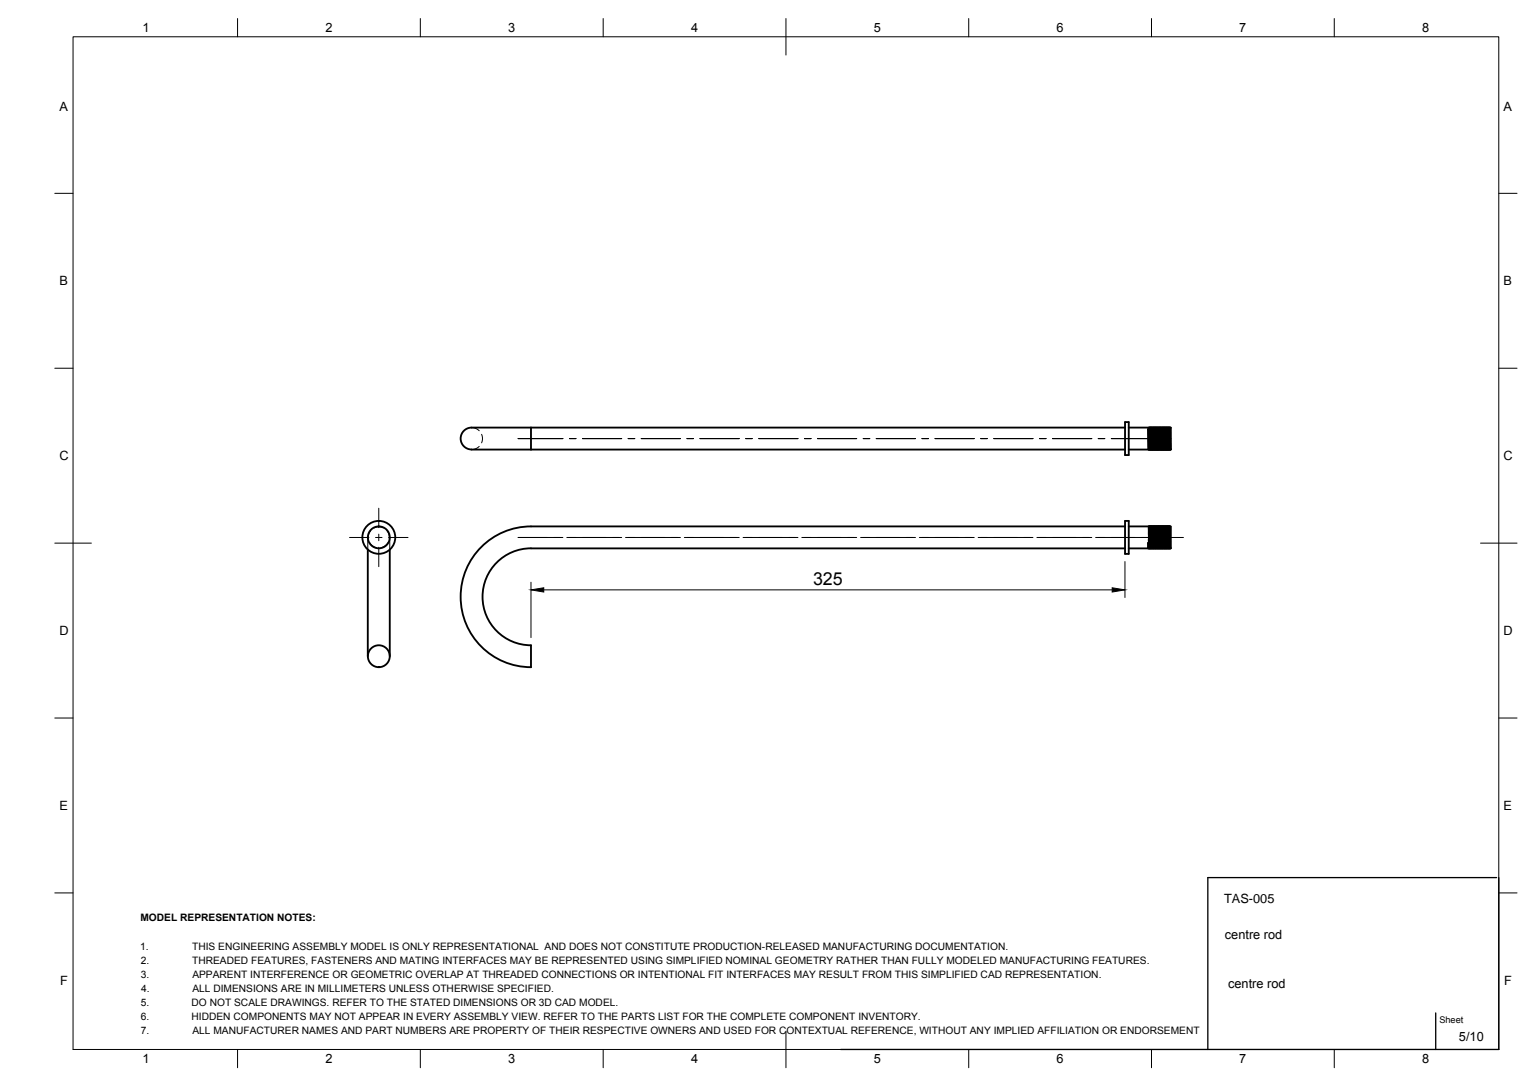
ISO-10303-21;
HEADER;
/* Generated by software containing ST-Developer
 * from STEP Tools, Inc. (www.steptools.com) 
 */

FILE_DESCRIPTION(
/* description */ ('STEP AP214'),
/* implementation_level */ '2;1');

FILE_NAME(
/* name */ 'centre rod.step',
/* time_stamp */ '2026-11-04T19:54:22-08:00',
/* author */ (''),
/* organization */ (''),
/* preprocessor_version */ 'ST-DEVELOPER v20.2',
/* originating_system */ 'Autodesk Translation Framework v15.17.0.0',
/* authorisation */ '');

FILE_SCHEMA (('AUTOMOTIVE_DESIGN { 1 0 10303 214 3 1 1 }'));
ENDSEC;

DATA;
#10=MECHANICAL_DESIGN_GEOMETRIC_PRESENTATION_REPRESENTATION('',(#241),#14084);
#61=(
BOUNDED_SURFACE()
B_SPLINE_SURFACE(1,2,((#7888,#7889,#7890,#7891,#7892,#7893,#7894,#7895,
#7896,#7897,#7898,#7899,#7900,#7901,#7902,#7903,#7904,#7905,#7906,#7907,
#7908,#7909,#7910,#7911,#7912,#7913,#7914,#7915,#7916,#7917,#7918,#7919,
#7920,#7921,#7922,#7923,#7924,#7925,#7926,#7927,#7928,#7929,#7930,#7931,
#7932,#7933,#7934,#7935,#7936,#7937,#7938,#7939,#7940,#7941,#7942,#7943,
#7944,#7945,#7946,#7947,#7948,#7949,#7950,#7951,#7952,#7953,#7954,#7955,
#7956,#7957,#7958,#7959,#7960,#7961,#7962,#7963,#7964,#7965,#7966,#7967,
#7968,#7969,#7970,#7971,#7972,#7973,#7974,#7975,#7976,#7977,#7978,#7979,
#7980,#7981,#7982,#7983,#7984,#7985,#7986,#7987,#7988,#7989,#7990,#7991,
#7992,#7993,#7994,#7995,#7996,#7997,#7998,#7999,#8000,#8001,#8002,#8003,
#8004,#8005,#8006,#8007,#8008,#8009,#8010,#8011,#8012,#8013,#8014,#8015,
#8016,#8017,#8018,#8019,#8020,#8021,#8022,#8023,#8024,#8025,#8026,#8027,
#8028,#8029,#8030,#8031,#8032,#8033,#8034,#8035,#8036,#8037,#8038,#8039,
#8040,#8041,#8042,#8043,#8044,#8045,#8046,#8047,#8048,#8049,#8050,#8051,
#8052,#8053,#8054,#8055,#8056,#8057,#8058,#8059,#8060,#8061,#8062,#8063,
#8064,#8065,#8066,#8067,#8068,#8069,#8070,#8071,#8072,#8073,#8074,#8075,
#8076,#8077,#8078,#8079,#8080,#8081,#8082,#8083,#8084,#8085,#8086,#8087,
#8088,#8089,#8090,#8091,#8092,#8093,#8094,#8095,#8096,#8097,#8098,#8099,
#8100,#8101,#8102,#8103,#8104,#8105,#8106,#8107,#8108,#8109,#8110,#8111,
#8112,#8113,#8114,#8115,#8116,#8117,#8118,#8119,#8120,#8121,#8122,#8123,
#8124,#8125,#8126,#8127,#8128,#8129,#8130,#8131,#8132,#8133,#8134,#8135,
#8136,#8137,#8138,#8139,#8140,#8141,#8142,#8143,#8144,#8145,#8146,#8147,
#8148,#8149,#8150,#8151,#8152,#8153,#8154,#8155,#8156,#8157,#8158,#8159,
#8160,#8161,#8162,#8163,#8164,#8165,#8166,#8167,#8168,#8169,#8170,#8171,
#8172,#8173,#8174,#8175,#8176,#8177,#8178,#8179,#8180,#8181,#8182,#8183,
#8184,#8185,#8186,#8187,#8188,#8189,#8190,#8191,#8192,#8193,#8194,#8195,
#8196,#8197,#8198,#8199,#8200,#8201,#8202,#8203,#8204,#8205,#8206,#8207,
#8208),(#8209,#8210,#8211,#8212,#8213,#8214,#8215,#8216,#8217,#8218,#8219,
#8220,#8221,#8222,#8223,#8224,#8225,#8226,#8227,#8228,#8229,#8230,#8231,
#8232,#8233,#8234,#8235,#8236,#8237,#8238,#8239,#8240,#8241,#8242,#8243,
#8244,#8245,#8246,#8247,#8248,#8249,#8250,#8251,#8252,#8253,#8254,#8255,
#8256,#8257,#8258,#8259,#8260,#8261,#8262,#8263,#8264,#8265,#8266,#8267,
#8268,#8269,#8270,#8271,#8272,#8273,#8274,#8275,#8276,#8277,#8278,#8279,
#8280,#8281,#8282,#8283,#8284,#8285,#8286,#8287,#8288,#8289,#8290,#8291,
#8292,#8293,#8294,#8295,#8296,#8297,#8298,#8299,#8300,#8301,#8302,#8303,
#8304,#8305,#8306,#8307,#8308,#8309,#8310,#8311,#8312,#8313,#8314,#8315,
#8316,#8317,#8318,#8319,#8320,#8321,#8322,#8323,#8324,#8325,#8326,#8327,
#8328,#8329,#8330,#8331,#8332,#8333,#8334,#8335,#8336,#8337,#8338,#8339,
#8340,#8341,#8342,#8343,#8344,#8345,#8346,#8347,#8348,#8349,#8350,#8351,
#8352,#8353,#8354,#8355,#8356,#8357,#8358,#8359,#8360,#8361,#8362,#8363,
#8364,#8365,#8366,#8367,#8368,#8369,#8370,#8371,#8372,#8373,#8374,#8375,
#8376,#8377,#8378,#8379,#8380,#8381,#8382,#8383,#8384,#8385,#8386,#8387,
#8388,#8389,#8390,#8391,#8392,#8393,#8394,#8395,#8396,#8397,#8398,#8399,
#8400,#8401,#8402,#8403,#8404,#8405,#8406,#8407,#8408,#8409,#8410,#8411,
#8412,#8413,#8414,#8415,#8416,#8417,#8418,#8419,#8420,#8421,#8422,#8423,
#8424,#8425,#8426,#8427,#8428,#8429,#8430,#8431,#8432,#8433,#8434,#8435,
#8436,#8437,#8438,#8439,#8440,#8441,#8442,#8443,#8444,#8445,#8446,#8447,
#8448,#8449,#8450,#8451,#8452,#8453,#8454,#8455,#8456,#8457,#8458,#8459,
#8460,#8461,#8462,#8463,#8464,#8465,#8466,#8467,#8468,#8469,#8470,#8471,
#8472,#8473,#8474,#8475,#8476,#8477,#8478,#8479,#8480,#8481,#8482,#8483,
#8484,#8485,#8486,#8487,#8488,#8489,#8490,#8491,#8492,#8493,#8494,#8495,
#8496,#8497,#8498,#8499,#8500,#8501,#8502,#8503,#8504,#8505,#8506,#8507,
#8508,#8509,#8510,#8511,#8512,#8513,#8514,#8515,#8516,#8517,#8518,#8519,
#8520,#8521,#8522,#8523,#8524,#8525,#8526,#8527,#8528,#8529)),
 .UNSPECIFIED.,.F.,.F.,.F.)
B_SPLINE_SURFACE_WITH_KNOTS((2,2),(3,2,2,2,2,2,2,2,2,2,2,2,2,2,2,2,2,2,
2,2,2,2,2,2,2,2,2,2,2,2,2,2,2,2,2,2,2,2,2,2,2,2,2,2,2,2,2,2,2,2,2,2,2,2,
2,2,2,2,2,2,2,2,2,2,2,2,2,2,2,2,2,2,2,2,2,2,2,2,2,2,2,2,2,2,2,2,2,2,2,2,
2,2,2,2,2,2,2,2,2,2,2,2,2,2,2,2,2,2,2,2,2,2,2,2,2,2,2,2,2,2,2,2,2,2,2,2,
2,2,2,2,2,2,2,2,2,2,2,2,2,2,2,2,2,2,2,2,2,2,2,2,2,2,2,2,2,2,2,2,2,2,3),
(0.,1.),(0.,0.00617283950617284,0.0123456790123457,0.0185185185185185,0.0246913580246914,
0.0308641975308642,0.037037037037037,0.0432098765432099,0.0493827160493827,
0.0555555555555556,0.0617283950617284,0.0679012345679012,0.0740740740740741,
0.0802469135802469,0.0864197530864197,0.0925925925925926,0.0987654320987654,
0.104938271604938,0.111111111111111,0.117283950617284,0.123456790123457,
0.12962962962963,0.135802469135802,0.141975308641975,0.148148148148148,
0.154320987654321,0.160493827160494,0.166666666666667,0.172839506172839,
0.179012345679012,0.185185185185185,0.191358024691358,0.197530864197531,
0.203703703703704,0.209876543209877,0.216049382716049,0.222222222222222,
0.228395061728395,0.234567901234568,0.240740740740741,0.246913580246914,
0.253086419753086,0.259259259259259,0.265432098765432,0.271604938271605,
0.277777777777778,0.283950617283951,0.290123456790123,0.296296296296296,
0.302469135802469,0.308641975308642,0.314814814814815,0.320987654320988,
0.327160493827161,0.333333333333333,0.339506172839506,0.345679012345679,
0.351851851851852,0.358024691358025,0.364197530864198,0.37037037037037,
0.376543209876543,0.382716049382716,0.388888888888889,0.395061728395062,
0.401234567901235,0.407407407407407,0.41358024691358,0.419753086419753,
0.425925925925926,0.432098765432099,0.438271604938272,0.444444444444444,
0.450617283950617,0.45679012345679,0.462962962962963,0.469135802469136,
0.475308641975309,0.481481481481481,0.487654320987654,0.493827160493827,
0.5,0.506172839506173,0.512345679012346,0.518518518518518,0.524691358024691,
0.530864197530864,0.537037037037037,0.54320987654321,0.549382716049383,
0.555555555555556,0.561728395061728,0.567901234567901,0.574074074074074,
0.580246913580247,0.58641975308642,0.592592592592593,0.598765432098765,
0.604938271604938,0.611111111111111,0.617283950617284,0.623456790123457,
0.62962962962963,0.635802469135803,0.641975308641975,0.648148148148148,
0.654320987654321,0.660493827160494,0.666666666666667,0.672839506172839,
0.679012345679012,0.685185185185185,0.691358024691358,0.697530864197531,
0.703703703703704,0.709876543209877,0.716049382716049,0.722222222222222,
0.728395061728395,0.734567901234568,0.740740740740741,0.746913580246914,
0.753086419753086,0.759259259259259,0.765432098765432,0.771604938271605,
0.777777777777778,0.783950617283951,0.790123456790123,0.796296296296296,
0.802469135802469,0.808641975308642,0.814814814814815,0.820987654320988,
0.827160493827161,0.833333333333333,0.839506172839506,0.845679012345679,
0.851851851851852,0.858024691358025,0.864197530864197,0.87037037037037,
0.876543209876543,0.882716049382716,0.888888888888889,0.895061728395062,
0.901234567901235,0.907407407407407,0.91358024691358,0.919753086419753,
0.925925925925926,0.932098765432099,0.938271604938272,0.944444444444444,
0.950617283950617,0.95679012345679,0.962962962962963,0.969135802469136,
0.975308641975309,0.981481481481482,0.987654320987654),.UNSPECIFIED.)
GEOMETRIC_REPRESENTATION_ITEM()
RATIONAL_B_SPLINE_SURFACE(((1.,0.866025403784439,1.,0.866025403784439,1.,
0.866025403784439,1.,0.866025403784439,1.,0.866025403784439,1.,0.866025403784439,
1.,0.866025403784439,1.,0.866025403784439,1.,0.866025403784439,1.,0.866025403784439,
1.,0.866025403784439,1.,0.866025403784439,1.,0.866025403784439,1.,0.866025403784439,
1.,0.866025403784439,1.,0.866025403784439,1.,0.866025403784439,1.,0.866025403784439,
1.,0.866025403784439,1.,0.866025403784439,1.,0.866025403784439,1.,0.866025403784439,
1.,0.866025403784439,1.,0.866025403784439,1.,0.866025403784439,1.,0.866025403784439,
1.,0.866025403784439,1.,0.866025403784439,1.,0.866025403784439,1.,0.866025403784439,
1.,0.866025403784439,1.,0.866025403784439,1.,0.866025403784439,1.,0.866025403784439,
1.,0.866025403784439,1.,0.866025403784439,1.,0.866025403784439,1.,0.866025403784439,
1.,0.866025403784439,1.,0.866025403784439,1.,0.866025403784439,1.,0.866025403784439,
1.,0.866025403784439,1.,0.866025403784439,1.,0.866025403784439,1.,0.866025403784439,
1.,0.866025403784439,1.,0.866025403784439,1.,0.866025403784439,1.,0.866025403784439,
1.,0.866025403784439,1.,0.866025403784439,1.,0.866025403784439,1.,0.866025403784439,
1.,0.866025403784439,1.,0.866025403784439,1.,0.866025403784439,1.,0.866025403784439,
1.,0.866025403784439,1.,0.866025403784439,1.,0.866025403784439,1.,0.866025403784439,
1.,0.866025403784439,1.,0.866025403784439,1.,0.866025403784439,1.,0.866025403784439,
1.,0.866025403784439,1.,0.866025403784439,1.,0.866025403784439,1.,0.866025403784439,
1.,0.866025403784439,1.,0.866025403784439,1.,0.866025403784439,1.,0.866025403784439,
1.,0.866025403784439,1.,0.866025403784439,1.,0.866025403784439,1.,0.866025403784439,
1.,0.866025403784439,1.,0.866025403784439,1.,0.866025403784439,1.,0.866025403784439,
1.,0.866025403784439,1.,0.866025403784439,1.,0.866025403784439,1.,0.866025403784439,
1.,0.866025403784439,1.,0.866025403784439,1.,0.866025403784439,1.,0.866025403784439,
1.,0.866025403784439,1.,0.866025403784439,1.,0.866025403784439,1.,0.866025403784439,
1.,0.866025403784439,1.,0.866025403784439,1.,0.866025403784439,1.,0.866025403784439,
1.,0.866025403784439,1.,0.866025403784439,1.,0.866025403784439,1.,0.866025403784439,
1.,0.866025403784439,1.,0.866025403784439,1.,0.866025403784439,1.,0.866025403784439,
1.,0.866025403784439,1.,0.866025403784439,1.,0.866025403784439,1.,0.866025403784439,
1.,0.866025403784439,1.,0.866025403784439,1.,0.866025403784439,1.,0.866025403784439,
1.,0.866025403784439,1.,0.866025403784439,1.,0.866025403784439,1.,0.866025403784439,
1.,0.866025403784439,1.,0.866025403784439,1.,0.866025403784439,1.,0.866025403784439,
1.,0.866025403784439,1.,0.866025403784439,1.,0.866025403784439,1.,0.866025403784439,
1.,0.866025403784439,1.,0.866025403784439,1.,0.866025403784439,1.,0.866025403784439,
1.,0.866025403784439,1.,0.866025403784439,1.,0.866025403784439,1.,0.866025403784439,
1.,0.866025403784439,1.,0.866025403784439,1.,0.866025403784439,1.,0.866025403784439,
1.,0.866025403784439,1.,0.866025403784439,1.,0.866025403784439,1.,0.866025403784439,
1.,0.866025403784439,1.,0.866025403784439,1.,0.866025403784439,1.,0.866025403784439,
1.,0.866025403784439,1.,0.866025403784439,1.,0.866025403784439,1.,0.866025403784439,
1.,0.866025403784439,1.,0.866025403784439,1.,0.866025403784439,1.,0.866025403784439,
1.,0.866025403784439,1.,0.866025403784439,1.,0.866025403784439,1.,0.866025403784439,
1.,0.866025403784439,1.,0.866025403784439,1.),(1.,0.866025403784439,1.,
0.866025403784439,1.,0.866025403784439,1.,0.866025403784439,1.,0.866025403784439,
1.,0.866025403784439,1.,0.866025403784439,1.,0.866025403784439,1.,0.866025403784439,
1.,0.866025403784439,1.,0.866025403784439,1.,0.866025403784439,1.,0.866025403784439,
1.,0.866025403784439,1.,0.866025403784439,1.,0.866025403784439,1.,0.866025403784439,
1.,0.866025403784439,1.,0.866025403784439,1.,0.866025403784439,1.,0.866025403784439,
1.,0.866025403784439,1.,0.866025403784439,1.,0.866025403784439,1.,0.866025403784439,
1.,0.866025403784439,1.,0.866025403784439,1.,0.866025403784439,1.,0.866025403784439,
1.,0.866025403784439,1.,0.866025403784439,1.,0.866025403784439,1.,0.866025403784439,
1.,0.866025403784439,1.,0.866025403784439,1.,0.866025403784439,1.,0.866025403784439,
1.,0.866025403784439,1.,0.866025403784439,1.,0.866025403784439,1.,0.866025403784439,
1.,0.866025403784439,1.,0.866025403784439,1.,0.866025403784439,1.,0.866025403784439,
1.,0.866025403784439,1.,0.866025403784439,1.,0.866025403784439,1.,0.866025403784439,
1.,0.866025403784439,1.,0.866025403784439,1.,0.866025403784439,1.,0.866025403784439,
1.,0.866025403784439,1.,0.866025403784439,1.,0.866025403784439,1.,0.866025403784439,
1.,0.866025403784439,1.,0.866025403784439,1.,0.866025403784439,1.,0.866025403784439,
1.,0.866025403784439,1.,0.866025403784439,1.,0.866025403784439,1.,0.866025403784439,
1.,0.866025403784439,1.,0.866025403784439,1.,0.866025403784439,1.,0.866025403784439,
1.,0.866025403784439,1.,0.866025403784439,1.,0.866025403784439,1.,0.866025403784439,
1.,0.866025403784439,1.,0.866025403784439,1.,0.866025403784439,1.,0.866025403784439,
1.,0.866025403784439,1.,0.866025403784439,1.,0.866025403784439,1.,0.866025403784439,
1.,0.866025403784439,1.,0.866025403784439,1.,0.866025403784439,1.,0.866025403784439,
1.,0.866025403784439,1.,0.866025403784439,1.,0.866025403784439,1.,0.866025403784439,
1.,0.866025403784439,1.,0.866025403784439,1.,0.866025403784439,1.,0.866025403784439,
1.,0.866025403784439,1.,0.866025403784439,1.,0.866025403784439,1.,0.866025403784439,
1.,0.866025403784439,1.,0.866025403784439,1.,0.866025403784439,1.,0.866025403784439,
1.,0.866025403784439,1.,0.866025403784439,1.,0.866025403784439,1.,0.866025403784439,
1.,0.866025403784439,1.,0.866025403784439,1.,0.866025403784439,1.,0.866025403784439,
1.,0.866025403784439,1.,0.866025403784439,1.,0.866025403784439,1.,0.866025403784439,
1.,0.866025403784439,1.,0.866025403784439,1.,0.866025403784439,1.,0.866025403784439,
1.,0.866025403784439,1.,0.866025403784439,1.,0.866025403784439,1.,0.866025403784439,
1.,0.866025403784439,1.,0.866025403784439,1.,0.866025403784439,1.,0.866025403784439,
1.,0.866025403784439,1.,0.866025403784439,1.,0.866025403784439,1.,0.866025403784439,
1.,0.866025403784439,1.,0.866025403784439,1.,0.866025403784439,1.,0.866025403784439,
1.,0.866025403784439,1.,0.866025403784439,1.,0.866025403784439,1.,0.866025403784439,
1.,0.866025403784439,1.,0.866025403784439,1.,0.866025403784439,1.,0.866025403784439,
1.,0.866025403784439,1.,0.866025403784439,1.,0.866025403784439,1.,0.866025403784439,
1.,0.866025403784439,1.,0.866025403784439,1.,0.866025403784439,1.,0.866025403784439,
1.,0.866025403784439,1.,0.866025403784439,1.,0.866025403784439,1.,0.866025403784439,
1.,0.866025403784439,1.,0.866025403784439,1.,0.866025403784439,1.,0.866025403784439,
1.,0.866025403784439,1.,0.866025403784439,1.,0.866025403784439,1.)))
REPRESENTATION_ITEM('')
SURFACE()
);
#62=(
BOUNDED_SURFACE()
B_SPLINE_SURFACE(1,2,((#8545,#8546,#8547,#8548,#8549,#8550,#8551,#8552,
#8553,#8554,#8555,#8556,#8557,#8558,#8559,#8560,#8561,#8562,#8563,#8564,
#8565,#8566,#8567,#8568,#8569,#8570,#8571,#8572,#8573,#8574,#8575,#8576,
#8577,#8578,#8579,#8580,#8581,#8582,#8583,#8584,#8585,#8586,#8587,#8588,
#8589,#8590,#8591,#8592,#8593,#8594,#8595,#8596,#8597,#8598,#8599,#8600,
#8601,#8602,#8603,#8604,#8605,#8606,#8607,#8608,#8609,#8610,#8611,#8612,
#8613,#8614,#8615,#8616,#8617,#8618,#8619,#8620,#8621,#8622,#8623,#8624,
#8625,#8626,#8627,#8628,#8629,#8630,#8631,#8632,#8633,#8634,#8635,#8636,
#8637,#8638,#8639,#8640,#8641,#8642,#8643,#8644,#8645,#8646,#8647,#8648,
#8649,#8650,#8651,#8652,#8653,#8654,#8655,#8656,#8657,#8658,#8659,#8660,
#8661,#8662,#8663,#8664,#8665,#8666,#8667,#8668,#8669,#8670,#8671,#8672,
#8673,#8674,#8675,#8676,#8677,#8678,#8679,#8680,#8681,#8682,#8683,#8684,
#8685,#8686,#8687,#8688,#8689,#8690,#8691,#8692,#8693,#8694,#8695,#8696,
#8697,#8698,#8699,#8700,#8701,#8702,#8703,#8704,#8705,#8706,#8707,#8708,
#8709,#8710,#8711,#8712,#8713,#8714,#8715,#8716,#8717,#8718,#8719,#8720,
#8721,#8722,#8723,#8724,#8725,#8726,#8727,#8728,#8729,#8730,#8731,#8732,
#8733,#8734,#8735,#8736,#8737,#8738,#8739,#8740,#8741,#8742,#8743,#8744,
#8745,#8746,#8747,#8748,#8749,#8750,#8751,#8752,#8753,#8754,#8755,#8756,
#8757,#8758,#8759,#8760,#8761,#8762,#8763,#8764,#8765,#8766,#8767,#8768,
#8769,#8770,#8771,#8772,#8773,#8774,#8775,#8776,#8777,#8778,#8779,#8780,
#8781,#8782,#8783,#8784,#8785,#8786,#8787,#8788,#8789,#8790,#8791,#8792,
#8793,#8794,#8795,#8796,#8797,#8798,#8799,#8800,#8801,#8802,#8803,#8804,
#8805,#8806,#8807,#8808,#8809,#8810,#8811,#8812,#8813,#8814,#8815,#8816,
#8817,#8818,#8819,#8820,#8821,#8822,#8823,#8824,#8825,#8826,#8827,#8828,
#8829,#8830,#8831,#8832,#8833,#8834,#8835,#8836,#8837,#8838,#8839,#8840,
#8841,#8842,#8843,#8844,#8845,#8846,#8847,#8848,#8849,#8850,#8851,#8852,
#8853,#8854,#8855,#8856,#8857,#8858,#8859,#8860,#8861,#8862,#8863,#8864,
#8865),(#8866,#8867,#8868,#8869,#8870,#8871,#8872,#8873,#8874,#8875,#8876,
#8877,#8878,#8879,#8880,#8881,#8882,#8883,#8884,#8885,#8886,#8887,#8888,
#8889,#8890,#8891,#8892,#8893,#8894,#8895,#8896,#8897,#8898,#8899,#8900,
#8901,#8902,#8903,#8904,#8905,#8906,#8907,#8908,#8909,#8910,#8911,#8912,
#8913,#8914,#8915,#8916,#8917,#8918,#8919,#8920,#8921,#8922,#8923,#8924,
#8925,#8926,#8927,#8928,#8929,#8930,#8931,#8932,#8933,#8934,#8935,#8936,
#8937,#8938,#8939,#8940,#8941,#8942,#8943,#8944,#8945,#8946,#8947,#8948,
#8949,#8950,#8951,#8952,#8953,#8954,#8955,#8956,#8957,#8958,#8959,#8960,
#8961,#8962,#8963,#8964,#8965,#8966,#8967,#8968,#8969,#8970,#8971,#8972,
#8973,#8974,#8975,#8976,#8977,#8978,#8979,#8980,#8981,#8982,#8983,#8984,
#8985,#8986,#8987,#8988,#8989,#8990,#8991,#8992,#8993,#8994,#8995,#8996,
#8997,#8998,#8999,#9000,#9001,#9002,#9003,#9004,#9005,#9006,#9007,#9008,
#9009,#9010,#9011,#9012,#9013,#9014,#9015,#9016,#9017,#9018,#9019,#9020,
#9021,#9022,#9023,#9024,#9025,#9026,#9027,#9028,#9029,#9030,#9031,#9032,
#9033,#9034,#9035,#9036,#9037,#9038,#9039,#9040,#9041,#9042,#9043,#9044,
#9045,#9046,#9047,#9048,#9049,#9050,#9051,#9052,#9053,#9054,#9055,#9056,
#9057,#9058,#9059,#9060,#9061,#9062,#9063,#9064,#9065,#9066,#9067,#9068,
#9069,#9070,#9071,#9072,#9073,#9074,#9075,#9076,#9077,#9078,#9079,#9080,
#9081,#9082,#9083,#9084,#9085,#9086,#9087,#9088,#9089,#9090,#9091,#9092,
#9093,#9094,#9095,#9096,#9097,#9098,#9099,#9100,#9101,#9102,#9103,#9104,
#9105,#9106,#9107,#9108,#9109,#9110,#9111,#9112,#9113,#9114,#9115,#9116,
#9117,#9118,#9119,#9120,#9121,#9122,#9123,#9124,#9125,#9126,#9127,#9128,
#9129,#9130,#9131,#9132,#9133,#9134,#9135,#9136,#9137,#9138,#9139,#9140,
#9141,#9142,#9143,#9144,#9145,#9146,#9147,#9148,#9149,#9150,#9151,#9152,
#9153,#9154,#9155,#9156,#9157,#9158,#9159,#9160,#9161,#9162,#9163,#9164,
#9165,#9166,#9167,#9168,#9169,#9170,#9171,#9172,#9173,#9174,#9175,#9176,
#9177,#9178,#9179,#9180,#9181,#9182,#9183,#9184,#9185,#9186)),
 .UNSPECIFIED.,.F.,.F.,.F.)
B_SPLINE_SURFACE_WITH_KNOTS((2,2),(3,2,2,2,2,2,2,2,2,2,2,2,2,2,2,2,2,2,
2,2,2,2,2,2,2,2,2,2,2,2,2,2,2,2,2,2,2,2,2,2,2,2,2,2,2,2,2,2,2,2,2,2,2,2,
2,2,2,2,2,2,2,2,2,2,2,2,2,2,2,2,2,2,2,2,2,2,2,2,2,2,2,2,2,2,2,2,2,2,2,2,
2,2,2,2,2,2,2,2,2,2,2,2,2,2,2,2,2,2,2,2,2,2,2,2,2,2,2,2,2,2,2,2,2,2,2,2,
2,2,2,2,2,2,2,2,2,2,2,2,2,2,2,2,2,2,2,2,2,2,2,2,2,2,2,2,2,2,2,2,2,2,3),
(0.,1.),(0.,0.00617283950617284,0.0123456790123457,0.0185185185185185,0.0246913580246914,
0.0308641975308642,0.037037037037037,0.0432098765432099,0.0493827160493827,
0.0555555555555556,0.0617283950617284,0.0679012345679012,0.0740740740740741,
0.0802469135802469,0.0864197530864197,0.0925925925925926,0.0987654320987654,
0.104938271604938,0.111111111111111,0.117283950617284,0.123456790123457,
0.12962962962963,0.135802469135802,0.141975308641975,0.148148148148148,
0.154320987654321,0.160493827160494,0.166666666666667,0.172839506172839,
0.179012345679012,0.185185185185185,0.191358024691358,0.197530864197531,
0.203703703703704,0.209876543209877,0.216049382716049,0.222222222222222,
0.228395061728395,0.234567901234568,0.240740740740741,0.246913580246914,
0.253086419753086,0.259259259259259,0.265432098765432,0.271604938271605,
0.277777777777778,0.283950617283951,0.290123456790123,0.296296296296296,
0.302469135802469,0.308641975308642,0.314814814814815,0.320987654320988,
0.327160493827161,0.333333333333333,0.339506172839506,0.345679012345679,
0.351851851851852,0.358024691358025,0.364197530864198,0.37037037037037,
0.376543209876543,0.382716049382716,0.388888888888889,0.395061728395062,
0.401234567901235,0.407407407407407,0.41358024691358,0.419753086419753,
0.425925925925926,0.432098765432099,0.438271604938272,0.444444444444444,
0.450617283950617,0.45679012345679,0.462962962962963,0.469135802469136,
0.475308641975309,0.481481481481481,0.487654320987654,0.493827160493827,
0.5,0.506172839506173,0.512345679012346,0.518518518518518,0.524691358024691,
0.530864197530864,0.537037037037037,0.54320987654321,0.549382716049383,
0.555555555555556,0.561728395061728,0.567901234567901,0.574074074074074,
0.580246913580247,0.58641975308642,0.592592592592593,0.598765432098765,
0.604938271604938,0.611111111111111,0.617283950617284,0.623456790123457,
0.62962962962963,0.635802469135803,0.641975308641975,0.648148148148148,
0.654320987654321,0.660493827160494,0.666666666666667,0.672839506172839,
0.679012345679012,0.685185185185185,0.691358024691358,0.697530864197531,
0.703703703703704,0.709876543209877,0.716049382716049,0.722222222222222,
0.728395061728395,0.734567901234568,0.740740740740741,0.746913580246914,
0.753086419753086,0.759259259259259,0.765432098765432,0.771604938271605,
0.777777777777778,0.783950617283951,0.790123456790123,0.796296296296296,
0.802469135802469,0.808641975308642,0.814814814814815,0.820987654320988,
0.827160493827161,0.833333333333333,0.839506172839506,0.845679012345679,
0.851851851851852,0.858024691358025,0.864197530864197,0.87037037037037,
0.876543209876543,0.882716049382716,0.888888888888889,0.895061728395062,
0.901234567901235,0.907407407407407,0.91358024691358,0.919753086419753,
0.925925925925926,0.932098765432099,0.938271604938272,0.944444444444444,
0.950617283950617,0.95679012345679,0.962962962962963,0.969135802469136,
0.975308641975309,0.981481481481482,0.987654320987654),.UNSPECIFIED.)
GEOMETRIC_REPRESENTATION_ITEM()
RATIONAL_B_SPLINE_SURFACE(((1.,0.866025403784439,1.,0.866025403784439,1.,
0.866025403784439,1.,0.866025403784439,1.,0.866025403784439,1.,0.866025403784439,
1.,0.866025403784439,1.,0.866025403784439,1.,0.866025403784439,1.,0.866025403784439,
1.,0.866025403784439,1.,0.866025403784439,1.,0.866025403784439,1.,0.866025403784439,
1.,0.866025403784439,1.,0.866025403784439,1.,0.866025403784439,1.,0.866025403784439,
1.,0.866025403784439,1.,0.866025403784439,1.,0.866025403784439,1.,0.866025403784439,
1.,0.866025403784439,1.,0.866025403784439,1.,0.866025403784439,1.,0.866025403784439,
1.,0.866025403784439,1.,0.866025403784439,1.,0.866025403784439,1.,0.866025403784439,
1.,0.866025403784439,1.,0.866025403784439,1.,0.866025403784439,1.,0.866025403784439,
1.,0.866025403784439,1.,0.866025403784439,1.,0.866025403784439,1.,0.866025403784439,
1.,0.866025403784439,1.,0.866025403784439,1.,0.866025403784439,1.,0.866025403784439,
1.,0.866025403784439,1.,0.866025403784439,1.,0.866025403784439,1.,0.866025403784439,
1.,0.866025403784439,1.,0.866025403784439,1.,0.866025403784439,1.,0.866025403784439,
1.,0.866025403784439,1.,0.866025403784439,1.,0.866025403784439,1.,0.866025403784439,
1.,0.866025403784439,1.,0.866025403784439,1.,0.866025403784439,1.,0.866025403784439,
1.,0.866025403784439,1.,0.866025403784439,1.,0.866025403784439,1.,0.866025403784439,
1.,0.866025403784439,1.,0.866025403784439,1.,0.866025403784439,1.,0.866025403784439,
1.,0.866025403784439,1.,0.866025403784439,1.,0.866025403784439,1.,0.866025403784439,
1.,0.866025403784439,1.,0.866025403784439,1.,0.866025403784439,1.,0.866025403784439,
1.,0.866025403784439,1.,0.866025403784439,1.,0.866025403784439,1.,0.866025403784439,
1.,0.866025403784439,1.,0.866025403784439,1.,0.866025403784439,1.,0.866025403784439,
1.,0.866025403784439,1.,0.866025403784439,1.,0.866025403784439,1.,0.866025403784439,
1.,0.866025403784439,1.,0.866025403784439,1.,0.866025403784439,1.,0.866025403784439,
1.,0.866025403784439,1.,0.866025403784439,1.,0.866025403784439,1.,0.866025403784439,
1.,0.866025403784439,1.,0.866025403784439,1.,0.866025403784439,1.,0.866025403784439,
1.,0.866025403784439,1.,0.866025403784439,1.,0.866025403784439,1.,0.866025403784439,
1.,0.866025403784439,1.,0.866025403784439,1.,0.866025403784439,1.,0.866025403784439,
1.,0.866025403784439,1.,0.866025403784439,1.,0.866025403784439,1.,0.866025403784439,
1.,0.866025403784439,1.,0.866025403784439,1.,0.866025403784439,1.,0.866025403784439,
1.,0.866025403784439,1.,0.866025403784439,1.,0.866025403784439,1.,0.866025403784439,
1.,0.866025403784439,1.,0.866025403784439,1.,0.866025403784439,1.,0.866025403784439,
1.,0.866025403784439,1.,0.866025403784439,1.,0.866025403784439,1.,0.866025403784439,
1.,0.866025403784439,1.,0.866025403784439,1.,0.866025403784439,1.,0.866025403784439,
1.,0.866025403784439,1.,0.866025403784439,1.,0.866025403784439,1.,0.866025403784439,
1.,0.866025403784439,1.,0.866025403784439,1.,0.866025403784439,1.,0.866025403784439,
1.,0.866025403784439,1.,0.866025403784439,1.,0.866025403784439,1.,0.866025403784439,
1.,0.866025403784439,1.,0.866025403784439,1.,0.866025403784439,1.,0.866025403784439,
1.,0.866025403784439,1.,0.866025403784439,1.,0.866025403784439,1.,0.866025403784439,
1.,0.866025403784439,1.,0.866025403784439,1.,0.866025403784439,1.,0.866025403784439,
1.,0.866025403784439,1.,0.866025403784439,1.,0.866025403784439,1.,0.866025403784439,
1.,0.866025403784439,1.,0.866025403784439,1.),(1.,0.866025403784439,1.,
0.866025403784439,1.,0.866025403784439,1.,0.866025403784439,1.,0.866025403784439,
1.,0.866025403784439,1.,0.866025403784439,1.,0.866025403784439,1.,0.866025403784439,
1.,0.866025403784439,1.,0.866025403784439,1.,0.866025403784439,1.,0.866025403784439,
1.,0.866025403784439,1.,0.866025403784439,1.,0.866025403784439,1.,0.866025403784439,
1.,0.866025403784439,1.,0.866025403784439,1.,0.866025403784439,1.,0.866025403784439,
1.,0.866025403784439,1.,0.866025403784439,1.,0.866025403784439,1.,0.866025403784439,
1.,0.866025403784439,1.,0.866025403784439,1.,0.866025403784439,1.,0.866025403784439,
1.,0.866025403784439,1.,0.866025403784439,1.,0.866025403784439,1.,0.866025403784439,
1.,0.866025403784439,1.,0.866025403784439,1.,0.866025403784439,1.,0.866025403784439,
1.,0.866025403784439,1.,0.866025403784439,1.,0.866025403784439,1.,0.866025403784439,
1.,0.866025403784439,1.,0.866025403784439,1.,0.866025403784439,1.,0.866025403784439,
1.,0.866025403784439,1.,0.866025403784439,1.,0.866025403784439,1.,0.866025403784439,
1.,0.866025403784439,1.,0.866025403784439,1.,0.866025403784439,1.,0.866025403784439,
1.,0.866025403784439,1.,0.866025403784439,1.,0.866025403784439,1.,0.866025403784439,
1.,0.866025403784439,1.,0.866025403784439,1.,0.866025403784439,1.,0.866025403784439,
1.,0.866025403784439,1.,0.866025403784439,1.,0.866025403784439,1.,0.866025403784439,
1.,0.866025403784439,1.,0.866025403784439,1.,0.866025403784439,1.,0.866025403784439,
1.,0.866025403784439,1.,0.866025403784439,1.,0.866025403784439,1.,0.866025403784439,
1.,0.866025403784439,1.,0.866025403784439,1.,0.866025403784439,1.,0.866025403784439,
1.,0.866025403784439,1.,0.866025403784439,1.,0.866025403784439,1.,0.866025403784439,
1.,0.866025403784439,1.,0.866025403784439,1.,0.866025403784439,1.,0.866025403784439,
1.,0.866025403784439,1.,0.866025403784439,1.,0.866025403784439,1.,0.866025403784439,
1.,0.866025403784439,1.,0.866025403784439,1.,0.866025403784439,1.,0.866025403784439,
1.,0.866025403784439,1.,0.866025403784439,1.,0.866025403784439,1.,0.866025403784439,
1.,0.866025403784439,1.,0.866025403784439,1.,0.866025403784439,1.,0.866025403784439,
1.,0.866025403784439,1.,0.866025403784439,1.,0.866025403784439,1.,0.866025403784439,
1.,0.866025403784439,1.,0.866025403784439,1.,0.866025403784439,1.,0.866025403784439,
1.,0.866025403784439,1.,0.866025403784439,1.,0.866025403784439,1.,0.866025403784439,
1.,0.866025403784439,1.,0.866025403784439,1.,0.866025403784439,1.,0.866025403784439,
1.,0.866025403784439,1.,0.866025403784439,1.,0.866025403784439,1.,0.866025403784439,
1.,0.866025403784439,1.,0.866025403784439,1.,0.866025403784439,1.,0.866025403784439,
1.,0.866025403784439,1.,0.866025403784439,1.,0.866025403784439,1.,0.866025403784439,
1.,0.866025403784439,1.,0.866025403784439,1.,0.866025403784439,1.,0.866025403784439,
1.,0.866025403784439,1.,0.866025403784439,1.,0.866025403784439,1.,0.866025403784439,
1.,0.866025403784439,1.,0.866025403784439,1.,0.866025403784439,1.,0.866025403784439,
1.,0.866025403784439,1.,0.866025403784439,1.,0.866025403784439,1.,0.866025403784439,
1.,0.866025403784439,1.,0.866025403784439,1.,0.866025403784439,1.,0.866025403784439,
1.,0.866025403784439,1.,0.866025403784439,1.,0.866025403784439,1.,0.866025403784439,
1.,0.866025403784439,1.,0.866025403784439,1.,0.866025403784439,1.,0.866025403784439,
1.,0.866025403784439,1.,0.866025403784439,1.,0.866025403784439,1.)))
REPRESENTATION_ITEM('')
SURFACE()
);
#71=TOROIDAL_SURFACE('',#3707,32.5,6.);
#73=B_SPLINE_CURVE_WITH_KNOTS('',3,(#5793,#5794,#5795,#5796,#5797,#5798,
#5799,#5800,#5801,#5802,#5803,#5804),.UNSPECIFIED.,.F.,.F.,(4,2,2,2,2,4),
(-0.945051167958466,-0.841574089668648,-0.613708642186743,-0.375417318601337,
-0.18453510953063,0.),.UNSPECIFIED.);
#74=B_SPLINE_CURVE_WITH_KNOTS('',3,(#5810,#5811,#5812,#5813,#5814,#5815,
#5816,#5817,#5818,#5819,#5820,#5821,#5822,#5823,#5824,#5825,#5826,#5827,
#5828,#5829,#5830,#5831,#5832,#5833,#5834,#5835,#5836,#5837,#5838,#5839,
#5840,#5841,#5842,#5843,#5844,#5845),.UNSPECIFIED.,.F.,.F.,(4,2,2,2,2,2,
2,2,2,2,2,2,2,2,2,2,2,4),(-4.72701070515396,-4.58342020211309,-4.35573092128894,
-4.11738182551202,-3.88511531766138,-3.65439161452862,-3.41571207551833,
-3.18605838418004,-2.94775202391993,-2.71206608145108,-2.48446949005175,
-2.24614932091124,-2.01315165334969,-1.78371039541636,-1.54421591254515,
-1.3138550329973,-1.07808333104171,-0.945051167958466),.UNSPECIFIED.);
#75=B_SPLINE_CURVE_WITH_KNOTS('',3,(#5849,#5850,#5851,#5852,#5853,#5854,
#5855,#5856,#5857,#5858,#5859,#5860),.UNSPECIFIED.,.F.,.F.,(4,2,2,2,2,4),
(-100.860857186755,-100.719016322246,-100.572167893934,-100.332434988478,
-100.10326726078,-99.9157943215848),.UNSPECIFIED.);
#76=B_SPLINE_CURVE_WITH_KNOTS('',3,(#5865,#5866,#5867,#5868,#5869,#5870,
#5871,#5872,#5873,#5874,#5875,#5876,#5877,#5878,#5879,#5880,#5881,#5882,
#5883,#5884,#5885,#5886,#5887,#5888,#5889,#5890,#5891,#5892,#5893,#5894,
#5895,#5896,#5897,#5898,#5899,#5900),.UNSPECIFIED.,.F.,.F.,(4,2,2,2,2,2,
2,2,2,2,2,2,2,2,2,2,2,4),(-8.50901118085528,-8.32791893771986,-8.0990928267591,
-7.85910788244872,-7.62832437277772,-7.39390458531972,-7.15690768647293,
-6.92871712936123,-6.69044824129429,-6.45624357767479,-6.22815323543594,
-5.98733458562093,-5.75583554263634,-5.52335400543344,-5.28554117046482,
-5.05664510291043,-4.81833115193754,-4.72701070515396),.UNSPECIFIED.);
#77=B_SPLINE_CURVE_WITH_KNOTS('',3,(#5901,#5902,#5903,#5904,#5905,#5906,
#5907,#5908,#5909,#5910,#5911,#5912,#5913,#5914,#5915,#5916,#5917,#5918,
#5919,#5920,#5921,#5922,#5923,#5924,#5925,#5926,#5927,#5928,#5929,#5930,
#5931,#5932,#5933,#5934,#5935,#5936),.UNSPECIFIED.,.F.,.F.,(4,2,2,2,2,2,
2,2,2,2,2,2,2,2,2,2,2,4),(-99.9157943215848,-99.8700528920271,-99.6317245970861,
-99.4040778368149,-99.1681604611512,-98.9305377965158,-98.7006844014331,
-98.4617770049481,-98.2314058094206,-97.9989345477104,-97.7605772193135,
-97.5329301202136,-97.2978042552567,-97.0574907391568,-96.8283107464464,
-96.590175509048,-96.3583458899543,-96.1336669438351),.UNSPECIFIED.);
#78=B_SPLINE_CURVE_WITH_KNOTS('',3,(#5941,#5942,#5943,#5944,#5945,#5946,
#5947,#5948,#5949,#5950,#5951,#5952,#5953,#5954,#5955,#5956,#5957,#5958,
#5959,#5960,#5961,#5962,#5963,#5964,#5965,#5966,#5967,#5968,#5969,#5970,
#5971,#5972,#5973,#5974,#5975,#5976),.UNSPECIFIED.,.F.,.F.,(4,2,2,2,2,2,
2,2,2,2,2,2,2,2,2,2,2,4),(-12.2907867440871,-12.0718236771256,-11.8405116446575,
-11.602154571369,-11.3727826264931,-11.13338422805,-10.8980284551473,-10.670441358598,
-10.4321155432753,-10.1994280209644,-9.96950449632101,-9.73035393254469,
-9.50029148770774,-9.26352608944506,-9.02736214272124,-8.79965739283195,
-8.56136063203866,-8.50901118085528),.UNSPECIFIED.);
#79=B_SPLINE_CURVE_WITH_KNOTS('',3,(#5977,#5978,#5979,#5980,#5981,#5982,
#5983,#5984,#5985,#5986,#5987,#5988,#5989,#5990,#5991,#5992,#5993,#5994,
#5995,#5996,#5997,#5998,#5999,#6000,#6001,#6002,#6003,#6004,#6005,#6006,
#6007,#6008,#6009,#6010,#6011,#6012,#6013,#6014),.UNSPECIFIED.,.F.,.F.,
(4,2,2,2,2,2,2,2,2,2,2,2,2,2,2,2,2,2,4),(-96.1336669438351,-96.1265611334031,
-95.8881753300681,-95.6602076690697,-95.4257999831089,-95.1875195318992,
-94.9591189897511,-94.7218709411051,-94.4879625687659,-94.2569562534328,
-94.0167165913897,-93.7880836305017,-93.5544076599296,-93.3160825836461,
-93.0882520436014,-92.8518366239696,-92.6156796890001,-92.3853966159876,
-92.3513747143654),.UNSPECIFIED.);
#80=B_SPLINE_CURVE_WITH_KNOTS('',3,(#6019,#6020,#6021,#6022,#6023,#6024,
#6025,#6026,#6027,#6028,#6029,#6030,#6031,#6032,#6033,#6034,#6035,#6036,
#6037,#6038,#6039,#6040,#6041,#6042,#6043,#6044,#6045,#6046,#6047,#6048,
#6049,#6050,#6051,#6052,#6053,#6054,#6055,#6056),.UNSPECIFIED.,.F.,.F.,
(4,2,2,2,2,2,2,2,2,2,2,2,2,2,2,2,2,2,4),(-16.0726421798861,-16.0448513456216,
-15.8143696875198,-15.5789960071959,-15.3423470933369,-15.1144009066226,
-14.8761154158147,-14.6422274147382,-14.4138663966335,-14.1733928484136,
-13.9421888767155,-13.708935835368,-13.4714587727836,-13.2428582790979,
-13.0045799578113,-12.7699694473923,-12.5421573893674,-12.3038028906354,
-12.2907867440871),.UNSPECIFIED.);
#81=B_SPLINE_CURVE_WITH_KNOTS('',3,(#6057,#6058,#6059,#6060,#6061,#6062,
#6063,#6064,#6065,#6066,#6067,#6068,#6069,#6070,#6071,#6072,#6073,#6074,
#6075,#6076,#6077,#6078,#6079,#6080,#6081,#6082,#6083,#6084,#6085,#6086,
#6087,#6088,#6089,#6090,#6091,#6092),.UNSPECIFIED.,.F.,.F.,(4,2,2,2,2,2,
2,2,2,2,2,2,2,2,2,2,2,4),(-92.3513747143654,-92.1459953794631,-91.9163548635556,
-91.6834391927834,-91.4450851548889,-91.2174685300907,-90.9818718133715,
-90.7431410078649,-90.5135598140373,-90.2749665782474,-90.044002763264,
-89.8118106876991,-89.5734277997817,-89.345669086319,-89.110837285638,-88.8725049462534,
-88.6436870106884,-88.5689774530533),.UNSPECIFIED.);
#82=B_SPLINE_CURVE_WITH_KNOTS('',3,(#6097,#6098,#6099,#6100,#6101,#6102,
#6103,#6104,#6105,#6106,#6107,#6108,#6109,#6110,#6111,#6112,#6113,#6114,
#6115,#6116,#6117,#6118,#6119,#6120,#6121,#6122,#6123,#6124,#6125,#6126,
#6127,#6128,#6129,#6130,#6131,#6132),.UNSPECIFIED.,.F.,.F.,(4,2,2,2,2,2,
2,2,2,2,2,2,2,2,2,2,2,4),(-19.8545421250936,-19.7886210374653,-19.5595194352788,
-19.3189557440687,-19.0839201041549,-18.8562708334143,-18.6179276836627,
-18.3855426708408,-18.1550554085007,-17.9162429867753,-17.6864737489498,
-17.4486140745901,-17.2127927161367,-16.9851780130659,-16.746863863508,
-16.5137398595355,-16.2844857040836,-16.0726421798861),.UNSPECIFIED.);
#83=B_SPLINE_CURVE_WITH_KNOTS('',3,(#6133,#6134,#6135,#6136,#6137,#6138,
#6139,#6140,#6141,#6142,#6143,#6144,#6145,#6146,#6147,#6148,#6149,#6150,
#6151,#6152,#6153,#6154,#6155,#6156,#6157,#6158,#6159,#6160,#6161,#6162,
#6163,#6164,#6165,#6166,#6167,#6168),.UNSPECIFIED.,.F.,.F.,(4,2,2,2,2,2,
2,2,2,2,2,2,2,2,2,2,2,4),(-88.5689774530533,-88.4059660126083,-88.1731764713921,
-87.9417553066357,-87.7010318555137,-87.4728183271102,-87.2386994385408,
-87.000392596865,-86.7722693783642,-86.5353697816887,-86.3005728167057,
-86.0698705375273,-85.8299838138407,-85.6009757129622,-85.3676210877026,
-85.129286020926,-84.9015921002416,-84.7864811960255),.UNSPECIFIED.);
#84=B_SPLINE_CURVE_WITH_KNOTS('',3,(#6173,#6174,#6175,#6176,#6177,#6178,
#6179,#6180,#6181,#6182,#6183,#6184,#6185,#6186,#6187,#6188,#6189,#6190,
#6191,#6192,#6193,#6194,#6195,#6196,#6197,#6198,#6199,#6200,#6201,#6202,
#6203,#6204,#6205,#6206,#6207,#6208),.UNSPECIFIED.,.F.,.F.,(4,2,2,2,2,2,
2,2,2,2,2,2,2,2,2,2,2,4),(-23.6364428905114,-23.5280727188282,-23.3003170968824,
-23.0620315711668,-22.8284660746515,-22.599797428317,-22.3596760760626,
-22.1287758117826,-21.8947223471241,-21.6575908713894,-21.4292896926289,
-21.1910315806139,-20.9567054769666,-20.7287091966259,-20.4903376329144,
-20.2586320072491,-20.0266683991165,-19.8545421250936),.UNSPECIFIED.);
#85=B_SPLINE_CURVE_WITH_KNOTS('',3,(#6209,#6210,#6211,#6212,#6213,#6214,
#6215,#6216,#6217,#6218,#6219,#6220,#6221,#6222,#6223,#6224,#6225,#6226,
#6227,#6228,#6229,#6230,#6231,#6232,#6233,#6234,#6235,#6236,#6237,#6238,
#6239,#6240,#6241,#6242,#6243,#6244),.UNSPECIFIED.,.F.,.F.,(4,2,2,2,2,2,
2,2,2,2,2,2,2,2,2,2,2,4),(-84.7864811960255,-84.6655244516862,-84.4283266068344,
-84.1983430392082,-83.9592870567852,-83.7291292347511,-83.4965240136712,
-83.2581598823036,-83.0305262715843,-82.795259343992,-82.5553979452392,
-82.3260971111831,-82.0878248655658,-81.8562429676943,-81.6243359927227,
-81.3859432768132,-81.1580373792479,-81.0040618503967),.UNSPECIFIED.);
#86=B_SPLINE_CURVE_WITH_KNOTS('',3,(#6249,#6250,#6251,#6252,#6253,#6254,
#6255,#6256,#6257,#6258,#6259,#6260,#6261,#6262,#6263,#6264,#6265,#6266,
#6267,#6268,#6269,#6270,#6271,#6272,#6273,#6274,#6275,#6276,#6277,#6278,
#6279,#6280,#6281,#6282,#6283,#6284),.UNSPECIFIED.,.F.,.F.,(4,2,2,2,2,2,
2,2,2,2,2,2,2,2,2,2,2,4),(-27.4182083858629,-27.2701824506046,-27.0424357273862,
-26.8040924069698,-26.5720037208871,-26.340949280599,-26.1024683172712,
-25.8729888257624,-25.634057144684,-25.3985738820072,-25.1709986113392,
-24.9326840817343,-24.6998769564909,-24.4701692126494,-24.2308851039948,
-24.0007075184348,-23.7643712325812,-23.6364428905114),.UNSPECIFIED.);
#87=B_SPLINE_CURVE_WITH_KNOTS('',3,(#6285,#6286,#6287,#6288,#6289,#6290,
#6291,#6292,#6293,#6294,#6295,#6296,#6297,#6298,#6299,#6300,#6301,#6302,
#6303,#6304,#6305,#6306,#6307,#6308,#6309,#6310,#6311,#6312,#6313,#6314,
#6315,#6316,#6317,#6318,#6319,#6320),.UNSPECIFIED.,.F.,.F.,(4,2,2,2,2,2,
2,2,2,2,2,2,2,2,2,2,2,4),(-81.0040618503967,-80.92350308096,-80.6852010443942,
-80.4566759266639,-80.2192876137424,-79.9856970630905,-79.7545672730092,
-79.5141847658083,-79.2856734462051,-79.0518665659799,-78.8135388051234,
-78.5856317966836,-78.3490744232575,-78.113299330973,-77.8828928362824,
-77.643349760312,-77.413888713748,-77.2215001553636),.UNSPECIFIED.);
#88=B_SPLINE_CURVE_WITH_KNOTS('',3,(#6325,#6326,#6327,#6328,#6329,#6330,
#6331,#6332,#6333,#6334,#6335,#6336,#6337,#6338,#6339,#6340,#6341,#6342,
#6343,#6344,#6345,#6346,#6347,#6348,#6349,#6350,#6351,#6352,#6353,#6354,
#6355,#6356,#6357,#6358,#6359,#6360),.UNSPECIFIED.,.F.,.F.,(4,2,2,2,2,2,
2,2,2,2,2,2,2,2,2,2,2,4),(-31.2000580417808,-31.0140725636771,-30.7850089289431,
-30.5452410020026,-30.3146451340147,-30.079677015553,-29.8428951155429,
-29.6148653852519,-29.3765956140283,-29.1425869882947,-28.9143527457507,
-28.6737469858917,-28.4424308234987,-28.2095103262391,-27.9719044243992,
-27.7431911460644,-27.5049074861638,-27.4182083858629),.UNSPECIFIED.);
#89=B_SPLINE_CURVE_WITH_KNOTS('',3,(#6361,#6362,#6363,#6364,#6365,#6366,
#6367,#6368,#6369,#6370,#6371,#6372,#6373,#6374,#6375,#6376,#6377,#6378,
#6379,#6380,#6381,#6382,#6383,#6384,#6385,#6386,#6387,#6388,#6389,#6390,
#6391,#6392,#6393,#6394,#6395,#6396,#6397,#6398),.UNSPECIFIED.,.F.,.F.,
(4,2,2,2,2,2,2,2,2,2,2,2,2,2,2,2,2,2,4),(-77.2215001553636,-77.1808445817772,
-76.9424879838381,-76.7148550360144,-76.4791214839487,-76.24081517708,-76.0111164482566,
-75.7723890603129,-75.5416493168672,-75.309337139177,-75.0709516032645,
-74.8432306674689,-74.6082731469132,-74.3699212863644,-74.1409797468126,
-73.9031186514559,-73.6706272268202,-73.4390822861619,-73.4390542992583),
 .UNSPECIFIED.);
#90=B_SPLINE_CURVE_WITH_KNOTS('',3,(#6403,#6404,#6405,#6406,#6407,#6408,
#6409,#6410,#6411,#6412,#6413,#6414,#6415,#6416,#6417,#6418,#6419,#6420,
#6421,#6422,#6423,#6424,#6425,#6426,#6427,#6428,#6429,#6430,#6431,#6432,
#6433,#6434,#6435,#6436,#6437,#6438),.UNSPECIFIED.,.F.,.F.,(4,2,2,2,2,2,
2,2,2,2,2,2,2,2,2,2,2,4),(-34.9817405379481,-34.7583828467543,-34.5266960718299,
-34.2885333255229,-34.0593317151714,-33.8192528633057,-33.5840972266921,
-33.3564889441506,-33.1181617298444,-32.8856634252833,-32.6554200731001,
-32.4164800124183,-32.1866008400906,-31.949200980976,-31.7132497196655,
-31.4856149669365,-31.2473168000567,-31.2000580417808),.UNSPECIFIED.);
#91=B_SPLINE_CURVE_WITH_KNOTS('',3,(#6439,#6440,#6441,#6442,#6443,#6444,
#6445,#6446,#6447,#6448,#6449,#6450,#6451,#6452,#6453,#6454,#6455,#6456,
#6457,#6458,#6459,#6460,#6461,#6462,#6463,#6464,#6465,#6466,#6467,#6468,
#6469,#6470,#6471,#6472,#6473,#6474),.UNSPECIFIED.,.F.,.F.,(4,2,2,2,2,2,
2,2,2,2,2,2,2,2,2,2,2,4),(-73.4390542992583,-73.1982145373766,-72.9700975195046,
-72.7358457406193,-72.4975408236058,-72.2693054491002,-72.0322598549638,
-71.7978365151172,-71.5670068623664,-71.3269726164317,-71.0981253205832,
-70.8646364649506,-70.6263037079221,-70.3985595539543,-70.1623470914066,
-69.9255831849977,-69.6954748942385,-69.6566458982394),.UNSPECIFIED.);
#92=B_SPLINE_CURVE_WITH_KNOTS('',3,(#6479,#6480,#6481,#6482,#6483,#6484,
#6485,#6486,#6487,#6488,#6489,#6490,#6491,#6492,#6493,#6494,#6495,#6496,
#6497,#6498,#6499,#6500,#6501,#6502,#6503,#6504,#6505,#6506,#6507,#6508,
#6509,#6510,#6511,#6512,#6513,#6514,#6515,#6516),.UNSPECIFIED.,.F.,.F.,
(4,2,2,2,2,2,2,2,2,2,2,2,2,2,2,2,2,2,4),(-38.7635679894171,-38.730951426609,
-38.5006459899062,-38.2646912803571,-38.0282461533568,-37.8004147265788,
-37.5621215735029,-37.3284203348966,-37.0998739613677,-36.8596046467075,
-36.6285759264362,-36.3948415542348,-36.1575645239461,-35.9291406831464,
-35.6908838834915,-35.4564528376755,-35.2285451591809,-34.9901894258272,
-34.9817405379481),.UNSPECIFIED.);
#93=B_SPLINE_CURVE_WITH_KNOTS('',3,(#6517,#6518,#6519,#6520,#6521,#6522,
#6523,#6524,#6525,#6526,#6527,#6528,#6529,#6530,#6531,#6532,#6533,#6534,
#6535,#6536,#6537,#6538,#6539,#6540,#6541,#6542,#6543,#6544,#6545,#6546,
#6547,#6548,#6549,#6550,#6551,#6552),.UNSPECIFIED.,.F.,.F.,(4,2,2,2,2,2,
2,2,2,2,2,2,2,2,2,2,2,4),(-69.6566458982394,-69.4562754604573,-69.2263356551233,
-68.9936015034485,-68.7552396899331,-68.5276187183144,-68.292215225518,
-68.052821027123,-67.8234040515846,-67.5849991258093,-67.353674141074,-67.1216493381286,
-66.8832588270564,-66.6554174863463,-66.4207605499414,-66.1824448046608,
-65.9537989682913,-65.8742130838229),.UNSPECIFIED.);
#94=B_SPLINE_CURVE_WITH_KNOTS('',3,(#6557,#6558,#6559,#6560,#6561,#6562,
#6563,#6564,#6565,#6566,#6567,#6568,#6569,#6570,#6571,#6572,#6573,#6574,
#6575,#6576,#6577,#6578,#6579,#6580,#6581,#6582,#6583,#6584,#6585,#6586,
#6587,#6588,#6589,#6590,#6591,#6592),.UNSPECIFIED.,.F.,.F.,(4,2,2,2,2,2,
2,2,2,2,2,2,2,2,2,2,2,4),(-42.5454845738913,-42.4722250372372,-42.2433846535402,
-42.0050768911068,-41.7702225547603,-41.5425130766005,-41.304162127578,
-41.0719495737161,-40.8411173069286,-40.6024982836502,-40.3728973337731,
-40.1343873884848,-39.8987632388426,-39.6711722063643,-39.4328501439237,
-39.1999103036718,-38.9703818511288,-38.7635679894171),.UNSPECIFIED.);
#95=B_SPLINE_CURVE_WITH_KNOTS('',3,(#6593,#6594,#6595,#6596,#6597,#6598,
#6599,#6600,#6601,#6602,#6603,#6604,#6605,#6606,#6607,#6608,#6609,#6610,
#6611,#6612,#6613,#6614,#6615,#6616,#6617,#6618,#6619,#6620,#6621,#6622,
#6623,#6624,#6625,#6626,#6627,#6628),.UNSPECIFIED.,.F.,.F.,(4,2,2,2,2,2,
2,2,2,2,2,2,2,2,2,2,2,4),(-65.8742130838229,-65.7162737876648,-65.4830140253136,
-65.2517643749619,-65.0112419678356,-64.7828569895144,-64.5489221737502,
-64.3106010757685,-64.0826126583152,-63.8459154416866,-63.6105409825893,
-63.3800136247092,-63.1403304694885,-62.9110577329829,-62.6778871130127,
-62.4395373717821,-62.2118860415347,-62.0916342174998),.UNSPECIFIED.);
#96=B_SPLINE_CURVE_WITH_KNOTS('',3,(#6633,#6634,#6635,#6636,#6637,#6638,
#6639,#6640,#6641,#6642,#6643,#6644,#6645,#6646,#6647,#6648,#6649,#6650,
#6651,#6652,#6653,#6654,#6655,#6656,#6657,#6658,#6659,#6660,#6661,#6662,
#6663,#6664,#6665,#6666,#6667,#6668),.UNSPECIFIED.,.F.,.F.,(4,2,2,2,2,2,
2,2,2,2,2,2,2,2,2,2,2,4),(-46.3274862212502,-46.2139349710691,-45.9862520631046,
-45.7479510822666,-45.514570222929,-45.2856655043703,-45.0457476103363,
-44.8150216716406,-44.5804220517271,-44.3434914755233,-44.1153521114665,
-43.877079193963,-43.642934622709,-43.4147962866385,-43.1740430399489,-42.9425997608968,
-42.7099744625215,-42.5454845738913),.UNSPECIFIED.);
#97=B_SPLINE_CURVE_WITH_KNOTS('',3,(#6669,#6670,#6671,#6672,#6673,#6674,
#6675,#6676,#6677,#6678,#6679,#6680,#6681,#6682,#6683,#6684,#6685,#6686,
#6687,#6688,#6689,#6690,#6691,#6692,#6693,#6694,#6695,#6696,#6697,#6698,
#6699,#6700,#6701,#6702,#6703,#6704),.UNSPECIFIED.,.F.,.F.,(4,2,2,2,2,2,
2,2,2,2,2,2,2,2,2,2,2,4),(-62.0916342174998,-61.9760168268649,-61.7381605371751,
-61.5083461244539,-61.2694855976273,-61.0389840970219,-60.80655322902,-60.5681744778011,
-60.3404938262001,-60.1054113560928,-59.8648525874502,-59.6357068116143,
-59.3976125670906,-59.1656371959061,-58.9338869248346,-58.6954797464671,
-58.4674560570048,-58.3090769307648),.UNSPECIFIED.);
#98=B_SPLINE_CURVE_WITH_KNOTS('',3,(#6709,#6710,#6711,#6712,#6713,#6714,
#6715,#6716,#6717,#6718,#6719,#6720,#6721,#6722,#6723,#6724,#6725,#6726,
#6727,#6728,#6729,#6730,#6731,#6732,#6733,#6734,#6735,#6736,#6737,#6738,
#6739,#6740,#6741,#6742,#6743,#6744),.UNSPECIFIED.,.F.,.F.,(4,2,2,2,2,2,
2,2,2,2,2,2,2,2,2,2,2,4),(-50.1093942211471,-49.9567830768948,-49.7289379381517,
-49.4905792650358,-49.2586532650307,-49.0272163525885,-48.7889194778806,
-48.5595999453668,-48.3199763649759,-48.0846826473659,-47.857087398902,
-47.6187573557871,-47.3861282487955,-47.156098687667,-46.9170133518871,
-46.6870073167293,-46.4500330423276,-46.3274862212502),.UNSPECIFIED.);
#99=B_SPLINE_CURVE_WITH_KNOTS('',3,(#6745,#6746,#6747,#6748,#6749,#6750,
#6751,#6752,#6753,#6754,#6755,#6756,#6757,#6758,#6759,#6760,#6761,#6762,
#6763,#6764,#6765,#6766,#6767,#6768,#6769,#6770,#6771,#6772,#6773,#6774,
#6775,#6776,#6777,#6778,#6779,#6780),.UNSPECIFIED.,.F.,.F.,(4,2,2,2,2,2,
2,2,2,2,2,2,2,2,2,2,2,4),(-58.3090769307648,-58.2330845708498,-57.994791177349,
-57.7664459669195,-57.5292676010225,-57.295207858664,-57.064263082704,-56.8240942169975,
-56.595403200837,-56.3617921973811,-56.1234714272172,-55.8956766402114,
-55.6593313097667,-55.4229936465461,-55.1927717434584,-54.9534404271447,
-54.7237149766201,-54.5267363962688),.UNSPECIFIED.);
#100=B_SPLINE_CURVE_WITH_KNOTS('',3,(#6785,#6786,#6787,#6788,#6789,#6790,
#6791,#6792,#6793,#6794,#6795,#6796,#6797,#6798,#6799,#6800,#6801,#6802,
#6803,#6804,#6805,#6806,#6807,#6808,#6809,#6810,#6811,#6812,#6813,#6814,
#6815,#6816,#6817,#6818,#6819,#6820),.UNSPECIFIED.,.F.,.F.,(4,2,2,2,2,2,
2,2,2,2,2,2,2,2,2,2,2,4),(-53.8914326771441,-53.6942463180612,-53.4641320716806,
-53.231536971558,-52.9931960827502,-52.765586112647,-52.5290010051772,-52.30109163005,
-52.0627998313959,-51.828969941831,-51.6005463821193,-51.3601365561174,
-51.1289868370583,-50.8955735447212,-50.6581587562352,-50.4296129262629,
-50.1913380824163,-50.1093942211471),.UNSPECIFIED.);
#101=B_SPLINE_CURVE_WITH_KNOTS('',3,(#6821,#6822,#6823,#6824,#6825,#6826,
#6827,#6828,#6829,#6830,#6831,#6832,#6833,#6834,#6835,#6836,#6837,#6838,
#6839,#6840,#6841,#6842,#6843,#6844,#6845,#6846,#6847,#6848,#6849,#6850,
#6851,#6852,#6853,#6854,#6855,#6856),.UNSPECIFIED.,.F.,.F.,(4,2,2,2,2,2,
2,2,2,2,2,2,2,2,2,2,2,4),(-54.5267363962688,-54.4908627524364,-54.2525129803029,
-54.0249036906896,-53.7893742600372,-53.5504440838935,-53.3209209565464,
-53.0823936458037,-52.8534147673518,-52.6135121188718,-52.382796618409,
-52.1480599607188,-51.911144561536,-51.6830108878803,-51.4447097678497,
-51.2105768919698,-50.9823832511243,-50.744421786252),.UNSPECIFIED.);
#102=B_SPLINE_CURVE_WITH_KNOTS('',3,(#6861,#6862,#6863,#6864,#6865,#6866,
#6867,#6868,#6869,#6870,#6871,#6872,#6873,#6874,#6875,#6876,#6877,#6878,
#6879,#6880,#6881,#6882,#6883,#6884,#6885,#6886,#6887,#6888,#6889,#6890,
#6891,#6892,#6893,#6894,#6895,#6896),.UNSPECIFIED.,.F.,.F.,(4,2,2,2,2,2,
2,2,2,2,2,2,2,2,2,2,2,4),(-57.6734244832962,-57.4356455965062,-57.207463872803,
-56.9733547726644,-56.7350711356582,-56.5069595853773,-56.2700688004548,
-56.0353309893982,-55.8046387301499,-55.5647609815634,-55.3357909413717,
-55.1024459514368,-54.864134125454,-54.6364578442597,-54.400399095822,-54.163266274685,
-53.9332929597696,-53.8914326771441),.UNSPECIFIED.);
#103=B_SPLINE_CURVE_WITH_KNOTS('',3,(#6897,#6898,#6899,#6900,#6901,#6902,
#6903,#6904,#6905,#6906,#6907,#6908,#6909,#6910,#6911,#6912,#6913,#6914,
#6915,#6916,#6917,#6918,#6919,#6920,#6921,#6922,#6923,#6924,#6925,#6926,
#6927,#6928,#6929,#6930,#6931,#6932,#6933,#6934),.UNSPECIFIED.,.F.,.F.,
(4,2,2,2,2,2,2,2,2,2,2,2,2,2,2,2,2,2,4),(-50.744421786252,-50.7416442860852,
-50.5102103743226,-50.2774702301927,-50.0397342334648,-49.8109034923061,
-49.5725737752064,-49.3377290004435,-49.1099815298265,-48.8716037031331,
-48.63939939237,-48.4084741501181,-48.1698667577858,-47.9402736227072,-47.7016109703721,
-47.4659996105955,-47.2383863882127,-47.0000374246888,-46.9621556460553),
 .UNSPECIFIED.);
#104=B_SPLINE_CURVE_WITH_KNOTS('',3,(#6939,#6940,#6941,#6942,#6943,#6944,
#6945,#6946,#6947,#6948,#6949,#6950,#6951,#6952,#6953,#6954,#6955,#6956,
#6957,#6958,#6959,#6960,#6961,#6962,#6963,#6964,#6965,#6966,#6967,#6968,
#6969,#6970,#6971,#6972,#6973,#6974,#6975,#6976),.UNSPECIFIED.,.F.,.F.,
(4,2,2,2,2,2,2,2,2,2,2,2,2,2,2,2,2,2,4),(-61.4554063830696,-61.4176876659541,
-61.1793564073111,-60.9517606003038,-60.7161733529179,-60.4775072406849,
-60.2479368198683,-60.0093536212889,-59.7784342335843,-59.5462529494306,
-59.3078928343578,-59.0801601502359,-58.8453388664692,-58.6070276784985,
-58.3782198817519,-58.140508292822,-57.9077705088657,-57.6763597347384,
-57.6734244832962),.UNSPECIFIED.);
#105=B_SPLINE_CURVE_WITH_KNOTS('',3,(#6977,#6978,#6979,#6980,#6981,#6982,
#6983,#6984,#6985,#6986,#6987,#6988,#6989,#6990,#6991,#6992,#6993,#6994,
#6995,#6996,#6997,#6998,#6999,#7000,#7001,#7002,#7003,#7004,#7005,#7006,
#7007,#7008,#7009,#7010,#7011,#7012),.UNSPECIFIED.,.F.,.F.,(4,2,2,2,2,2,
2,2,2,2,2,2,2,2,2,2,2,4),(-46.9621556460553,-46.7671082522818,-46.5374999065735,
-46.2980833389991,-46.0677874195046,-45.8316925770558,-45.5952617136895,
-45.3674257432928,-45.129105725766,-44.8954158475436,-44.6668066136594,
-44.4265514218191,-44.1955322085225,-43.9616766247489,-43.7244133311704,
-43.4959996459181,-43.2577215083365,-43.1798021454525),.UNSPECIFIED.);
#106=B_SPLINE_CURVE_WITH_KNOTS('',3,(#7017,#7018,#7019,#7020,#7021,#7022,
#7023,#7024,#7025,#7026,#7027,#7028,#7029,#7030,#7031,#7032,#7033,#7034,
#7035,#7036,#7037,#7038,#7039,#7040,#7041,#7042,#7043,#7044,#7045,#7046,
#7047,#7048,#7049,#7050,#7051,#7052),.UNSPECIFIED.,.F.,.F.,(4,2,2,2,2,2,
2,2,2,2,2,2,2,2,2,2,2,4),(-65.2374739513206,-65.1597137841198,-64.9214542750747,
-64.6930636066121,-64.4558247570368,-64.2219705028162,-63.9909744370199,
-63.7507440295899,-63.5221454619045,-63.2884792888966,-63.0501769792657,
-62.8223614114859,-62.5859549937987,-62.3498585298257,-62.1195856839448,
-61.8801937683809,-61.6505933291242,-61.4554063830696),.UNSPECIFIED.);
#107=B_SPLINE_CURVE_WITH_KNOTS('',3,(#7053,#7054,#7055,#7056,#7057,#7058,
#7059,#7060,#7061,#7062,#7063,#7064,#7065,#7066,#7067,#7068,#7069,#7070,
#7071,#7072,#7073,#7074,#7075,#7076,#7077,#7078,#7079,#7080,#7081,#7082,
#7083,#7084,#7085,#7086,#7087,#7088),.UNSPECIFIED.,.F.,.F.,(4,2,2,2,2,2,
2,2,2,2,2,2,2,2,2,2,2,4),(-43.1798021454525,-43.0233005184053,-42.7953477083257,
-42.5569663446575,-42.3251688520465,-42.0933816876821,-41.8552316604598,
-41.6260390539229,-41.3857985088062,-41.1506571598224,-40.9230178905739,
-40.6846650171423,-40.4521792375946,-40.2218455910818,-39.9829216392961,
-39.7530542026248,-39.5155007168095,-39.3976161936097),.UNSPECIFIED.);
#108=B_SPLINE_CURVE_WITH_KNOTS('',3,(#7093,#7094,#7095,#7096,#7097,#7098,
#7099,#7100,#7101,#7102,#7103,#7104,#7105,#7106,#7107,#7108,#7109,#7110,
#7111,#7112,#7113,#7114,#7115,#7116,#7117,#7118,#7119,#7120,#7121,#7122,
#7123,#7124,#7125,#7126,#7127,#7128),.UNSPECIFIED.,.F.,.F.,(4,2,2,2,2,2,
2,2,2,2,2,2,2,2,2,2,2,4),(-69.019372509275,-68.9016766044539,-68.6641192632124,
-68.434275259458,-68.1953763224697,-67.9650488487731,-67.7325868762516,
-67.4942519163572,-67.266628578738,-67.0315115784664,-66.7912661109365,
-66.5620964052668,-66.3239707395895,-66.0921882104742,-65.8604138727514,
-65.6220504300927,-65.3941112139331,-65.2374739513206),.UNSPECIFIED.);
#109=B_SPLINE_CURVE_WITH_KNOTS('',3,(#7129,#7130,#7131,#7132,#7133,#7134,
#7135,#7136,#7137,#7138,#7139,#7140,#7141,#7142,#7143,#7144,#7145,#7146,
#7147,#7148,#7149,#7150,#7151,#7152,#7153,#7154,#7155,#7156,#7157,#7158,
#7159,#7160,#7161,#7162,#7163,#7164),.UNSPECIFIED.,.F.,.F.,(4,2,2,2,2,2,
2,2,2,2,2,2,2,2,2,2,2,4),(-39.3976161936097,-39.2795664375483,-39.0519185558299,
-38.8135947219172,-38.580364848747,-38.3512267997343,-38.1114765039187,
-37.8808934389617,-37.6457880904805,-37.4090238643793,-37.1809993170469,
-36.9427039654236,-36.7087096301277,-36.4804196120852,-36.2398308864171,
-36.0085267678092,-35.7754906149688,-35.6153851283096),.UNSPECIFIED.);
#110=B_SPLINE_CURVE_WITH_KNOTS('',3,(#7169,#7170,#7171,#7172,#7173,#7174,
#7175,#7176,#7177,#7178,#7179,#7180,#7181,#7182,#7183,#7184,#7185,#7186,
#7187,#7188,#7189,#7190,#7191,#7192,#7193,#7194,#7195,#7196,#7197,#7198,
#7199,#7200,#7201,#7202,#7203,#7204),.UNSPECIFIED.,.F.,.F.,(4,2,2,2,2,2,
2,2,2,2,2,2,2,2,2,2,2,4),(-72.8013143187673,-72.6413921294953,-72.4083580675375,
-72.1770775857943,-71.9365142073292,-71.7082359793028,-71.4742659088467,
-71.2359884777822,-71.0079860078507,-70.771246873831,-70.5361401782511,
-70.3055808023638,-70.0658558659785,-69.8367265402269,-69.6035208632225,
-69.3652149385238,-69.1375859965796,-69.019372509275),.UNSPECIFIED.);
#111=B_SPLINE_CURVE_WITH_KNOTS('',3,(#7205,#7206,#7207,#7208,#7209,#7210,
#7211,#7212,#7213,#7214,#7215,#7216,#7217,#7218,#7219,#7220,#7221,#7222,
#7223,#7224,#7225,#7226,#7227,#7228,#7229,#7230,#7231,#7232,#7233,#7234,
#7235,#7236,#7237,#7238,#7239,#7240),.UNSPECIFIED.,.F.,.F.,(4,2,2,2,2,2,
2,2,2,2,2,2,2,2,2,2,2,4),(-35.6153851283096,-35.5379009882013,-35.3092001135616,
-35.0708970177155,-34.8361843624883,-34.6083995726921,-34.3700319850573,
-34.137954416543,-33.9068062025092,-33.668339927752,-33.4388711908287,-33.1997849001402,
-32.96431758397,-32.736719856299,-32.4983810318796,-32.2655877758767,-32.0357987356091,
-31.8332798855205),.UNSPECIFIED.);
#112=B_SPLINE_CURVE_WITH_KNOTS('',3,(#7245,#7246,#7247,#7248,#7249,#7250,
#7251,#7252,#7253,#7254,#7255,#7256,#7257,#7258,#7259,#7260,#7261,#7262,
#7263,#7264,#7265,#7266,#7267,#7268,#7269,#7270,#7271,#7272,#7273,#7274,
#7275,#7276,#7277,#7278,#7279,#7280),.UNSPECIFIED.,.F.,.F.,(4,2,2,2,2,2,
2,2,2,2,2,2,2,2,2,2,2,4),(-76.5831287300173,-76.3807946254889,-76.1510131669601,
-75.918244010913,-75.6799233281813,-75.4523429669146,-75.2169003495295,
-74.9778100888382,-74.7483646077869,-74.5099230950359,-74.2787804977059,
-74.0467264872251,-73.8083770487214,-73.580607008871,-73.3459183688024,
-73.1076342303079,-72.8789568137339,-72.8013143187673),.UNSPECIFIED.);
#113=B_SPLINE_CURVE_WITH_KNOTS('',3,(#7281,#7282,#7283,#7284,#7285,#7286,
#7287,#7288,#7289,#7290,#7291,#7292,#7293,#7294,#7295,#7296,#7297,#7298,
#7299,#7300,#7301,#7302,#7303,#7304,#7305,#7306,#7307,#7308,#7309,#7310,
#7311,#7312,#7313,#7314,#7315,#7316,#7317,#7318),.UNSPECIFIED.,.F.,.F.,
(4,2,2,2,2,2,2,2,2,2,2,2,2,2,2,2,2,2,4),(-31.8332798855205,-31.7965319071712,
-31.5663670970833,-31.3298877331002,-31.093607007729,-30.8658469576634,
-30.6275371592618,-30.39398655729,-30.1652536288997,-29.9251501787876,-29.6942629804963,
-29.4600849911831,-29.222971107908,-28.9946824297206,-28.7564001881208,
-28.5220881224759,-28.294045785471,-28.0556511973426,-28.051200537517),
 .UNSPECIFIED.);
#114=B_SPLINE_CURVE_WITH_KNOTS('',3,(#7323,#7324,#7325,#7326,#7327,#7328,
#7329,#7330,#7331,#7332,#7333,#7334,#7335,#7336,#7337,#7338,#7339,#7340,
#7341,#7342,#7343,#7344,#7345,#7346,#7347,#7348,#7349,#7350,#7351,#7352,
#7353,#7354,#7355,#7356,#7357,#7358,#7359,#7360),.UNSPECIFIED.,.F.,.F.,
(4,2,2,2,2,2,2,2,2,2,2,2,2,2,2,2,2,2,4),(-80.3649154835294,-80.3606244670685,
-80.1222482405985,-79.8942192990533,-79.6599315218819,-79.4216674436202,
-79.1934021475701,-78.9563134160552,-78.7221360441692,-78.4912726435801,
-78.251194673345,-78.0224721048771,-77.7889458569104,-77.5506542008286,
-77.3229145925487,-77.086658964388,-76.8501773059356,-76.62003616798,-76.5831287300173),
 .UNSPECIFIED.);
#115=B_SPLINE_CURVE_WITH_KNOTS('',3,(#7361,#7362,#7363,#7364,#7365,#7366,
#7367,#7368,#7369,#7370,#7371,#7372,#7373,#7374,#7375,#7376,#7377,#7378,
#7379,#7380,#7381,#7382,#7383,#7384,#7385,#7386,#7387,#7388,#7389,#7390,
#7391,#7392,#7393,#7394,#7395,#7396),.UNSPECIFIED.,.F.,.F.,(4,2,2,2,2,2,
2,2,2,2,2,2,2,2,2,2,2,4),(-28.051200537517,-27.8239586602662,-27.5918911071802,
-27.3538607998307,-27.1247722659998,-26.8840400858967,-26.6490232225647,
-26.4213420375868,-26.1829758350914,-25.9506078282134,-25.7200260903725,
-25.4812346407419,-25.2514816603531,-25.0134603157911,-24.7776609496024,
-24.5500328914262,-24.3116956709026,-24.2689961176951),.UNSPECIFIED.);
#116=B_SPLINE_CURVE_WITH_KNOTS('',3,(#7401,#7402,#7403,#7404,#7405,#7406,
#7407,#7408,#7409,#7410,#7411,#7412,#7413,#7414,#7415,#7416,#7417,#7418,
#7419,#7420,#7421,#7422,#7423,#7424,#7425,#7426,#7427,#7428,#7429,#7430,
#7431,#7432,#7433,#7434,#7435,#7436),.UNSPECIFIED.,.F.,.F.,(4,2,2,2,2,2,
2,2,2,2,2,2,2,2,2,2,2,4),(-84.1468249045191,-84.1043126875934,-83.8659938152791,
-83.6383846593357,-83.4026110967519,-83.1645843112362,-82.9348555875407,
-82.6960900426385,-82.4655136497021,-82.2331702678459,-81.9948224196279,
-81.7671569850544,-81.5321652925085,-81.2914268126568,-81.0623619202666,
-80.8243567680345,-80.5922931190962,-80.3649154835294),.UNSPECIFIED.);
#117=B_SPLINE_CURVE_WITH_KNOTS('',3,(#7437,#7438,#7439,#7440,#7441,#7442,
#7443,#7444,#7445,#7446,#7447,#7448,#7449,#7450,#7451,#7452,#7453,#7454,
#7455,#7456,#7457,#7458,#7459,#7460,#7461,#7462,#7463,#7464,#7465,#7466,
#7467,#7468,#7469,#7470,#7471,#7472),.UNSPECIFIED.,.F.,.F.,(4,2,2,2,2,2,
2,2,2,2,2,2,2,2,2,2,2,4),(-24.2689961176951,-24.0785909762214,-23.8492583670617,
-23.6096469956339,-23.3791830773827,-23.1436638044798,-22.9070380265563,
-22.6790982154573,-22.4407897223783,-22.2069213281478,-21.9785014716679,
-21.7380506822129,-21.5068639881352,-21.2734876567242,-21.0360326284573,
-20.8074498777589,-20.5691549873554,-20.4866764542111),.UNSPECIFIED.);
#118=B_SPLINE_CURVE_WITH_KNOTS('',3,(#7477,#7478,#7479,#7480,#7481,#7482,
#7483,#7484,#7485,#7486,#7487,#7488,#7489,#7490,#7491,#7492,#7493,#7494,
#7495,#7496,#7497,#7498,#7499,#7500,#7501,#7502,#7503,#7504,#7505,#7506,
#7507,#7508,#7509,#7510,#7511,#7512),.UNSPECIFIED.,.F.,.F.,(4,2,2,2,2,2,
2,2,2,2,2,2,2,2,2,2,2,4),(-87.928847460831,-87.846547736004,-87.6082722965554,
-87.3797139714847,-87.142284932425,-86.9089092219722,-86.6777471135071,
-86.4373227129817,-86.208914054241,-85.9750708910875,-85.7367807546045,
-85.5088632525325,-85.2722635629587,-85.036741320696,-84.8063019891483,
-84.5667169550491,-84.3373922845944,-84.1468249045191),.UNSPECIFIED.);
#119=B_SPLINE_CURVE_WITH_KNOTS('',3,(#7513,#7514,#7515,#7516,#7517,#7518,
#7519,#7520,#7521,#7522,#7523,#7524,#7525,#7526,#7527,#7528,#7529,#7530,
#7531,#7532,#7533,#7534,#7535,#7536,#7537,#7538,#7539,#7540,#7541,#7542,
#7543,#7544,#7545,#7546,#7547,#7548),.UNSPECIFIED.,.F.,.F.,(4,2,2,2,2,2,
2,2,2,2,2,2,2,2,2,2,2,4),(-20.4866764542111,-20.3345622966439,-20.1067107417864,
-19.8683346358064,-19.6363719390965,-19.4049599798345,-19.1666234905078,
-18.9372677343282,-18.6977030787119,-18.4623693329401,-18.2347591407509,
-17.9964116855308,-17.7637440061976,-17.5337330948493,-17.2946063174558,
-17.064562599015,-16.8276419602436,-16.7044808578381),.UNSPECIFIED.);
#120=B_SPLINE_CURVE_WITH_KNOTS('',3,(#7553,#7554,#7555,#7556,#7557,#7558,
#7559,#7560,#7561,#7562,#7563,#7564,#7565,#7566,#7567,#7568,#7569,#7570,
#7571,#7572,#7573,#7574,#7575,#7576,#7577,#7578,#7579,#7580,#7581,#7582,
#7583,#7584,#7585,#7586,#7587,#7588),.UNSPECIFIED.,.F.,.F.,(4,2,2,2,2,2,
2,2,2,2,2,2,2,2,2,2,2,4),(-91.7107443282099,-91.5877900079935,-91.3508647690065,
-91.1208457987438,-90.8817454870173,-90.6517409965148,-90.4190984985508,
-90.1807696362717,-89.9531766812327,-89.7178687370554,-89.478297886019,
-89.2489663680631,-89.0106557095446,-88.7792481826981,-88.5473100207957,
-88.3089525160693,-88.0811154260341,-87.928847460831),.UNSPECIFIED.);
#121=B_SPLINE_CURVE_WITH_KNOTS('',3,(#7589,#7590,#7591,#7592,#7593,#7594,
#7595,#7596,#7597,#7598,#7599,#7600,#7601,#7602,#7603,#7604,#7605,#7606,
#7607,#7608,#7609,#7610,#7611,#7612,#7613,#7614,#7615,#7616,#7617,#7618,
#7619,#7620,#7621,#7622,#7623,#7624),.UNSPECIFIED.,.F.,.F.,(4,2,2,2,2,2,
2,2,2,2,2,2,2,2,2,2,2,4),(-16.7044808578381,-16.5915024478014,-16.3637942465863,
-16.1254758543967,-15.8920554985378,-15.6631600972239,-15.4232000339098,
-15.1924359257727,-14.9578801876124,-14.7209079174785,-14.492733046275,
-14.2544426559687,-14.0202587552228,-13.7921192193288,-13.5513242752337,
-13.3198433681694,-13.0872496764959,-12.9221852831127),.UNSPECIFIED.);
#122=B_SPLINE_CURVE_WITH_KNOTS('',3,(#7629,#7630,#7631,#7632,#7633,#7634,
#7635,#7636,#7637,#7638,#7639,#7640,#7641,#7642,#7643,#7644,#7645,#7646,
#7647,#7648,#7649,#7650,#7651,#7652,#7653,#7654,#7655,#7656,#7657,#7658,
#7659,#7660,#7661,#7662,#7663,#7664),.UNSPECIFIED.,.F.,.F.,(4,2,2,2,2,2,
2,2,2,2,2,2,2,2,2,2,2,4),(-95.4927391051041,-95.3278706246628,-95.0952792884395,
-94.8638231831889,-94.6230548711802,-94.394928126947,-94.160769729705,-93.922497949396,
-93.6943470425071,-93.4574011982426,-93.2228439197167,-92.9921047539345,
-92.7521714347657,-92.523285440264,-92.2898906043006,-92.0515908033591,
-91.8239032182906,-91.7107443282099),.UNSPECIFIED.);
#123=B_SPLINE_CURVE_WITH_KNOTS('',3,(#7665,#7666,#7667,#7668,#7669,#7670,
#7671,#7672,#7673,#7674,#7675,#7676,#7677,#7678,#7679,#7680,#7681,#7682,
#7683,#7684,#7685,#7686,#7687,#7688,#7689,#7690,#7691,#7692,#7693,#7694,
#7695,#7696,#7697,#7698,#7699,#7700),.UNSPECIFIED.,.F.,.F.,(4,2,2,2,2,2,
2,2,2,2,2,2,2,2,2,2,2,4),(-12.9221852831127,-12.849459470145,-12.6205816823612,
-12.3822529170638,-12.1473603796708,-11.9196400813886,-11.681270901826,
-11.4490212687812,-11.2182085684104,-10.9795496790003,-10.7499122681144,
-10.5114542542116,-10.275790022471,-10.0481792806899,-9.80983900430133,
-9.57686066008535,-9.34734453006419,-9.1399695593726),.UNSPECIFIED.);
#124=B_SPLINE_CURVE_WITH_KNOTS('',3,(#7707,#7708,#7709,#7710,#7711,#7712,
#7713,#7714,#7715,#7716,#7717,#7718,#7719,#7720,#7721,#7722),
 .UNSPECIFIED.,.F.,.F.,(4,2,2,2,2,2,2,4),(-1.57584202720539,-1.390382595907,
-1.16132802380548,-0.921516936716486,-0.690881872470536,-0.455956835676362,
-0.224750643073495,0.),.UNSPECIFIED.);
#125=B_SPLINE_CURVE_WITH_KNOTS('',3,(#7726,#7727,#7728,#7729,#7730,#7731,
#7732,#7733,#7734,#7735,#7736,#7737,#7738,#7739,#7740,#7741,#7742,#7743),
 .UNSPECIFIED.,.F.,.F.,(4,2,2,2,2,2,2,2,4),(-100.849969952809,-100.666021642914,
-100.475737478142,-100.237444951456,-100.009605932478,-99.7731459818133,
-99.5372345319227,-99.3069163027839,-99.274652338909),.UNSPECIFIED.);
#126=B_SPLINE_CURVE_WITH_KNOTS('',3,(#7746,#7747,#7748,#7749,#7750,#7751,
#7752,#7753,#7754,#7755,#7756,#7757,#7758,#7759,#7760,#7761,#7762,#7763,
#7764,#7765,#7766,#7767,#7768,#7769,#7770,#7771,#7772,#7773,#7774,#7775,
#7776,#7777,#7778,#7779,#7780,#7781),.UNSPECIFIED.,.F.,.F.,(4,2,2,2,2,2,
2,2,2,2,2,2,2,2,2,2,2,4),(-5.35783695894723,-5.13494169831662,-4.90327828502939,
-4.66507524967157,-4.43583667566184,-4.19581412819847,-3.96061776270199,
-3.73299466112997,-3.49464853513548,-3.26211086848107,-3.03188532854683,
-2.79290302357929,-2.56298530835372,-2.32563744780847,-2.08964389026301,
-1.86198435100643,-1.62366727961924,-1.57584202720539),.UNSPECIFIED.);
#127=B_SPLINE_CURVE_WITH_KNOTS('',3,(#7791,#7792,#7793,#7794,#7795,#7796,
#7797,#7798,#7799,#7800,#7801,#7802,#7803,#7804,#7805,#7806,#7807,#7808,
#7809,#7810,#7811,#7812,#7813,#7814,#7815,#7816,#7817,#7818,#7819,#7820,
#7821,#7822,#7823,#7824,#7825,#7826),.UNSPECIFIED.,.F.,.F.,(4,2,2,2,2,2,
2,2,2,2,2,2,2,2,2,2,2,4),(-99.274652338909,-99.0674710790479,-98.8379634210678,
-98.6050102399715,-98.3666888177901,-98.1390968625289,-97.9034584541038,
-97.664996507285,-97.4353834154336,-97.1967504427233,-96.965943920785,-96.733718950633,
-96.495368632197,-96.2676642307138,-96.0327968656458,-95.7944878626794,
-95.5656346615004,-95.4927391051041),.UNSPECIFIED.);
#128=B_SPLINE_CURVE_WITH_KNOTS('',3,(#7827,#7828,#7829,#7830,#7831,#7832,
#7833,#7834,#7835,#7836,#7837,#7838,#7839,#7840,#7841,#7842,#7843,#7844,
#7845,#7846,#7847,#7848,#7849,#7850,#7851,#7852,#7853,#7854,#7855,#7856,
#7857,#7858,#7859,#7860,#7861,#7862,#7863,#7864),.UNSPECIFIED.,.F.,.F.,
(4,2,2,2,2,2,2,2,2,2,2,2,2,2,2,2,2,2,4),(-9.1399695593726,-9.10787291928304,
-8.87753000492313,-8.64162039097332,-8.40513428345374,-8.17727324440492,
-7.93896185891339,-7.7052216609661,-7.47667817446303,-7.23636744989055,
-7.00530119291182,-6.77160155078404,-6.5342837597148,-6.30582239728129,
-6.06754425945498,-5.83307490876647,-5.60516032837488,-5.36678566314923,
-5.35783695894723),.UNSPECIFIED.);
#151=(
BOUNDED_CURVE()
B_SPLINE_CURVE(2,(#5000,#5001,#5002),.UNSPECIFIED.,.F.,.F.)
B_SPLINE_CURVE_WITH_KNOTS((3,3),(0.981481481481482,0.987654320987654),
 .UNSPECIFIED.)
CURVE()
GEOMETRIC_REPRESENTATION_ITEM()
RATIONAL_B_SPLINE_CURVE((1.,0.866025403784439,1.))
REPRESENTATION_ITEM('')
);
#152=(
BOUNDED_CURVE()
B_SPLINE_CURVE(2,(#5005,#5006,#5007),.UNSPECIFIED.,.F.,.F.)
B_SPLINE_CURVE_WITH_KNOTS((3,3),(0.981481481481482,0.987654320987654),
 .UNSPECIFIED.)
CURVE()
GEOMETRIC_REPRESENTATION_ITEM()
RATIONAL_B_SPLINE_CURVE((1.,0.866025403784439,1.))
REPRESENTATION_ITEM('')
);
#153=(
BOUNDED_CURVE()
B_SPLINE_CURVE(2,(#5012,#5013,#5014,#5015,#5016,#5017,#5018,#5019,#5020,
#5021,#5022,#5023,#5024),.UNSPECIFIED.,.F.,.F.)
B_SPLINE_CURVE_WITH_KNOTS((3,2,2,2,2,2,3),(0.944444444444444,0.950617283950617,
0.95679012345679,0.962962962962963,0.969135802469136,0.975308641975309,
0.981481481481482),.UNSPECIFIED.)
CURVE()
GEOMETRIC_REPRESENTATION_ITEM()
RATIONAL_B_SPLINE_CURVE((1.,0.866025403784439,1.,0.866025403784439,1.,0.866025403784439,
1.,0.866025403784439,1.,0.866025403784439,1.,0.866025403784439,1.))
REPRESENTATION_ITEM('')
);
#154=(
BOUNDED_CURVE()
B_SPLINE_CURVE(2,(#5025,#5026,#5027,#5028,#5029,#5030,#5031,#5032,#5033,
#5034,#5035,#5036,#5037),.UNSPECIFIED.,.F.,.F.)
B_SPLINE_CURVE_WITH_KNOTS((3,2,2,2,2,2,3),(0.944444444444444,0.950617283950617,
0.95679012345679,0.962962962962963,0.969135802469136,0.975308641975309,
0.981481481481482),.UNSPECIFIED.)
CURVE()
GEOMETRIC_REPRESENTATION_ITEM()
RATIONAL_B_SPLINE_CURVE((1.,0.866025403784439,1.,0.866025403784439,1.,0.866025403784439,
1.,0.866025403784439,1.,0.866025403784439,1.,0.866025403784439,1.))
REPRESENTATION_ITEM('')
);
#155=(
BOUNDED_CURVE()
B_SPLINE_CURVE(2,(#5042,#5043,#5044,#5045,#5046,#5047,#5048,#5049,#5050,
#5051,#5052,#5053,#5054),.UNSPECIFIED.,.F.,.F.)
B_SPLINE_CURVE_WITH_KNOTS((3,2,2,2,2,2,3),(0.907407407407407,0.91358024691358,
0.919753086419753,0.925925925925926,0.932098765432099,0.938271604938272,
0.944444444444444),.UNSPECIFIED.)
CURVE()
GEOMETRIC_REPRESENTATION_ITEM()
RATIONAL_B_SPLINE_CURVE((1.,0.866025403784439,1.,0.866025403784439,1.,0.866025403784439,
1.,0.866025403784439,1.,0.866025403784439,1.,0.866025403784439,1.))
REPRESENTATION_ITEM('')
);
#156=(
BOUNDED_CURVE()
B_SPLINE_CURVE(2,(#5055,#5056,#5057,#5058,#5059,#5060,#5061,#5062,#5063,
#5064,#5065,#5066,#5067),.UNSPECIFIED.,.F.,.F.)
B_SPLINE_CURVE_WITH_KNOTS((3,2,2,2,2,2,3),(0.907407407407407,0.91358024691358,
0.919753086419753,0.925925925925926,0.932098765432099,0.938271604938272,
0.944444444444444),.UNSPECIFIED.)
CURVE()
GEOMETRIC_REPRESENTATION_ITEM()
RATIONAL_B_SPLINE_CURVE((1.,0.866025403784439,1.,0.866025403784439,1.,0.866025403784439,
1.,0.866025403784439,1.,0.866025403784439,1.,0.866025403784439,1.))
REPRESENTATION_ITEM('')
);
#157=(
BOUNDED_CURVE()
B_SPLINE_CURVE(2,(#5072,#5073,#5074,#5075,#5076,#5077,#5078,#5079,#5080,
#5081,#5082,#5083,#5084),.UNSPECIFIED.,.F.,.F.)
B_SPLINE_CURVE_WITH_KNOTS((3,2,2,2,2,2,3),(0.87037037037037,0.876543209876543,
0.882716049382716,0.888888888888889,0.895061728395062,0.901234567901235,
0.907407407407407),.UNSPECIFIED.)
CURVE()
GEOMETRIC_REPRESENTATION_ITEM()
RATIONAL_B_SPLINE_CURVE((1.,0.866025403784439,1.,0.866025403784439,1.,0.866025403784439,
1.,0.866025403784439,1.,0.866025403784439,1.,0.866025403784439,1.))
REPRESENTATION_ITEM('')
);
#158=(
BOUNDED_CURVE()
B_SPLINE_CURVE(2,(#5085,#5086,#5087,#5088,#5089,#5090,#5091,#5092,#5093,
#5094,#5095,#5096,#5097),.UNSPECIFIED.,.F.,.F.)
B_SPLINE_CURVE_WITH_KNOTS((3,2,2,2,2,2,3),(0.87037037037037,0.876543209876543,
0.882716049382716,0.888888888888889,0.895061728395062,0.901234567901235,
0.907407407407407),.UNSPECIFIED.)
CURVE()
GEOMETRIC_REPRESENTATION_ITEM()
RATIONAL_B_SPLINE_CURVE((1.,0.866025403784439,1.,0.866025403784439,1.,0.866025403784439,
1.,0.866025403784439,1.,0.866025403784439,1.,0.866025403784439,1.))
REPRESENTATION_ITEM('')
);
#159=(
BOUNDED_CURVE()
B_SPLINE_CURVE(2,(#5102,#5103,#5104,#5105,#5106,#5107,#5108,#5109,#5110,
#5111,#5112,#5113,#5114),.UNSPECIFIED.,.F.,.F.)
B_SPLINE_CURVE_WITH_KNOTS((3,2,2,2,2,2,3),(0.833333333333333,0.839506172839506,
0.845679012345679,0.851851851851852,0.858024691358025,0.864197530864197,
0.87037037037037),.UNSPECIFIED.)
CURVE()
GEOMETRIC_REPRESENTATION_ITEM()
RATIONAL_B_SPLINE_CURVE((1.,0.866025403784439,1.,0.866025403784439,1.,0.866025403784439,
1.,0.866025403784439,1.,0.866025403784439,1.,0.866025403784439,1.))
REPRESENTATION_ITEM('')
);
#160=(
BOUNDED_CURVE()
B_SPLINE_CURVE(2,(#5115,#5116,#5117,#5118,#5119,#5120,#5121,#5122,#5123,
#5124,#5125,#5126,#5127),.UNSPECIFIED.,.F.,.F.)
B_SPLINE_CURVE_WITH_KNOTS((3,2,2,2,2,2,3),(0.833333333333333,0.839506172839506,
0.845679012345679,0.851851851851852,0.858024691358025,0.864197530864197,
0.87037037037037),.UNSPECIFIED.)
CURVE()
GEOMETRIC_REPRESENTATION_ITEM()
RATIONAL_B_SPLINE_CURVE((1.,0.866025403784439,1.,0.866025403784439,1.,0.866025403784439,
1.,0.866025403784439,1.,0.866025403784439,1.,0.866025403784439,1.))
REPRESENTATION_ITEM('')
);
#161=(
BOUNDED_CURVE()
B_SPLINE_CURVE(2,(#5132,#5133,#5134,#5135,#5136,#5137,#5138,#5139,#5140,
#5141,#5142,#5143,#5144),.UNSPECIFIED.,.F.,.F.)
B_SPLINE_CURVE_WITH_KNOTS((3,2,2,2,2,2,3),(0.796296296296296,0.802469135802469,
0.808641975308642,0.814814814814815,0.820987654320988,0.827160493827161,
0.833333333333333),.UNSPECIFIED.)
CURVE()
GEOMETRIC_REPRESENTATION_ITEM()
RATIONAL_B_SPLINE_CURVE((1.,0.866025403784439,1.,0.866025403784439,1.,0.866025403784439,
1.,0.866025403784439,1.,0.866025403784439,1.,0.866025403784439,1.))
REPRESENTATION_ITEM('')
);
#162=(
BOUNDED_CURVE()
B_SPLINE_CURVE(2,(#5145,#5146,#5147,#5148,#5149,#5150,#5151,#5152,#5153,
#5154,#5155,#5156,#5157),.UNSPECIFIED.,.F.,.F.)
B_SPLINE_CURVE_WITH_KNOTS((3,2,2,2,2,2,3),(0.796296296296296,0.802469135802469,
0.808641975308642,0.814814814814815,0.820987654320988,0.827160493827161,
0.833333333333333),.UNSPECIFIED.)
CURVE()
GEOMETRIC_REPRESENTATION_ITEM()
RATIONAL_B_SPLINE_CURVE((1.,0.866025403784439,1.,0.866025403784439,1.,0.866025403784439,
1.,0.866025403784439,1.,0.866025403784439,1.,0.866025403784439,1.))
REPRESENTATION_ITEM('')
);
#163=(
BOUNDED_CURVE()
B_SPLINE_CURVE(2,(#5162,#5163,#5164,#5165,#5166,#5167,#5168,#5169,#5170,
#5171,#5172,#5173,#5174),.UNSPECIFIED.,.F.,.F.)
B_SPLINE_CURVE_WITH_KNOTS((3,2,2,2,2,2,3),(0.759259259259259,0.765432098765432,
0.771604938271605,0.777777777777778,0.783950617283951,0.790123456790123,
0.796296296296296),.UNSPECIFIED.)
CURVE()
GEOMETRIC_REPRESENTATION_ITEM()
RATIONAL_B_SPLINE_CURVE((1.,0.866025403784439,1.,0.866025403784439,1.,0.866025403784439,
1.,0.866025403784439,1.,0.866025403784439,1.,0.866025403784439,1.))
REPRESENTATION_ITEM('')
);
#164=(
BOUNDED_CURVE()
B_SPLINE_CURVE(2,(#5175,#5176,#5177,#5178,#5179,#5180,#5181,#5182,#5183,
#5184,#5185,#5186,#5187),.UNSPECIFIED.,.F.,.F.)
B_SPLINE_CURVE_WITH_KNOTS((3,2,2,2,2,2,3),(0.759259259259259,0.765432098765432,
0.771604938271605,0.777777777777778,0.783950617283951,0.790123456790123,
0.796296296296296),.UNSPECIFIED.)
CURVE()
GEOMETRIC_REPRESENTATION_ITEM()
RATIONAL_B_SPLINE_CURVE((1.,0.866025403784439,1.,0.866025403784439,1.,0.866025403784439,
1.,0.866025403784439,1.,0.866025403784439,1.,0.866025403784439,1.))
REPRESENTATION_ITEM('')
);
#165=(
BOUNDED_CURVE()
B_SPLINE_CURVE(2,(#5192,#5193,#5194,#5195,#5196,#5197,#5198,#5199,#5200,
#5201,#5202,#5203,#5204),.UNSPECIFIED.,.F.,.F.)
B_SPLINE_CURVE_WITH_KNOTS((3,2,2,2,2,2,3),(0.722222222222222,0.728395061728395,
0.734567901234568,0.740740740740741,0.746913580246914,0.753086419753086,
0.759259259259259),.UNSPECIFIED.)
CURVE()
GEOMETRIC_REPRESENTATION_ITEM()
RATIONAL_B_SPLINE_CURVE((1.,0.866025403784439,1.,0.866025403784439,1.,0.866025403784439,
1.,0.866025403784439,1.,0.866025403784439,1.,0.866025403784439,1.))
REPRESENTATION_ITEM('')
);
#166=(
BOUNDED_CURVE()
B_SPLINE_CURVE(2,(#5205,#5206,#5207,#5208,#5209,#5210,#5211,#5212,#5213,
#5214,#5215,#5216,#5217),.UNSPECIFIED.,.F.,.F.)
B_SPLINE_CURVE_WITH_KNOTS((3,2,2,2,2,2,3),(0.722222222222222,0.728395061728395,
0.734567901234568,0.740740740740741,0.746913580246914,0.753086419753086,
0.759259259259259),.UNSPECIFIED.)
CURVE()
GEOMETRIC_REPRESENTATION_ITEM()
RATIONAL_B_SPLINE_CURVE((1.,0.866025403784439,1.,0.866025403784439,1.,0.866025403784439,
1.,0.866025403784439,1.,0.866025403784439,1.,0.866025403784439,1.))
REPRESENTATION_ITEM('')
);
#167=(
BOUNDED_CURVE()
B_SPLINE_CURVE(2,(#5222,#5223,#5224,#5225,#5226,#5227,#5228,#5229,#5230,
#5231,#5232,#5233,#5234),.UNSPECIFIED.,.F.,.F.)
B_SPLINE_CURVE_WITH_KNOTS((3,2,2,2,2,2,3),(0.685185185185185,0.691358024691358,
0.697530864197531,0.703703703703704,0.709876543209877,0.716049382716049,
0.722222222222222),.UNSPECIFIED.)
CURVE()
GEOMETRIC_REPRESENTATION_ITEM()
RATIONAL_B_SPLINE_CURVE((1.,0.866025403784439,1.,0.866025403784439,1.,0.866025403784439,
1.,0.866025403784439,1.,0.866025403784439,1.,0.866025403784439,1.))
REPRESENTATION_ITEM('')
);
#168=(
BOUNDED_CURVE()
B_SPLINE_CURVE(2,(#5235,#5236,#5237,#5238,#5239,#5240,#5241,#5242,#5243,
#5244,#5245,#5246,#5247),.UNSPECIFIED.,.F.,.F.)
B_SPLINE_CURVE_WITH_KNOTS((3,2,2,2,2,2,3),(0.685185185185185,0.691358024691358,
0.697530864197531,0.703703703703704,0.709876543209877,0.716049382716049,
0.722222222222222),.UNSPECIFIED.)
CURVE()
GEOMETRIC_REPRESENTATION_ITEM()
RATIONAL_B_SPLINE_CURVE((1.,0.866025403784439,1.,0.866025403784439,1.,0.866025403784439,
1.,0.866025403784439,1.,0.866025403784439,1.,0.866025403784439,1.))
REPRESENTATION_ITEM('')
);
#169=(
BOUNDED_CURVE()
B_SPLINE_CURVE(2,(#5252,#5253,#5254,#5255,#5256,#5257,#5258,#5259,#5260,
#5261,#5262,#5263,#5264),.UNSPECIFIED.,.F.,.F.)
B_SPLINE_CURVE_WITH_KNOTS((3,2,2,2,2,2,3),(0.648148148148148,0.654320987654321,
0.660493827160494,0.666666666666667,0.672839506172839,0.679012345679012,
0.685185185185185),.UNSPECIFIED.)
CURVE()
GEOMETRIC_REPRESENTATION_ITEM()
RATIONAL_B_SPLINE_CURVE((1.,0.866025403784439,1.,0.866025403784439,1.,0.866025403784439,
1.,0.866025403784439,1.,0.866025403784439,1.,0.866025403784439,1.))
REPRESENTATION_ITEM('')
);
#170=(
BOUNDED_CURVE()
B_SPLINE_CURVE(2,(#5265,#5266,#5267,#5268,#5269,#5270,#5271,#5272,#5273,
#5274,#5275,#5276,#5277),.UNSPECIFIED.,.F.,.F.)
B_SPLINE_CURVE_WITH_KNOTS((3,2,2,2,2,2,3),(0.648148148148148,0.654320987654321,
0.660493827160494,0.666666666666667,0.672839506172839,0.679012345679012,
0.685185185185185),.UNSPECIFIED.)
CURVE()
GEOMETRIC_REPRESENTATION_ITEM()
RATIONAL_B_SPLINE_CURVE((1.,0.866025403784439,1.,0.866025403784439,1.,0.866025403784439,
1.,0.866025403784439,1.,0.866025403784439,1.,0.866025403784439,1.))
REPRESENTATION_ITEM('')
);
#171=(
BOUNDED_CURVE()
B_SPLINE_CURVE(2,(#5282,#5283,#5284,#5285,#5286,#5287,#5288,#5289,#5290,
#5291,#5292,#5293,#5294),.UNSPECIFIED.,.F.,.F.)
B_SPLINE_CURVE_WITH_KNOTS((3,2,2,2,2,2,3),(0.611111111111111,0.617283950617284,
0.623456790123457,0.62962962962963,0.635802469135803,0.641975308641975,
0.648148148148148),.UNSPECIFIED.)
CURVE()
GEOMETRIC_REPRESENTATION_ITEM()
RATIONAL_B_SPLINE_CURVE((1.,0.866025403784439,1.,0.866025403784439,1.,0.866025403784439,
1.,0.866025403784439,1.,0.866025403784439,1.,0.866025403784439,1.))
REPRESENTATION_ITEM('')
);
#172=(
BOUNDED_CURVE()
B_SPLINE_CURVE(2,(#5295,#5296,#5297,#5298,#5299,#5300,#5301,#5302,#5303,
#5304,#5305,#5306,#5307),.UNSPECIFIED.,.F.,.F.)
B_SPLINE_CURVE_WITH_KNOTS((3,2,2,2,2,2,3),(0.611111111111111,0.617283950617284,
0.623456790123457,0.62962962962963,0.635802469135803,0.641975308641975,
0.648148148148148),.UNSPECIFIED.)
CURVE()
GEOMETRIC_REPRESENTATION_ITEM()
RATIONAL_B_SPLINE_CURVE((1.,0.866025403784439,1.,0.866025403784439,1.,0.866025403784439,
1.,0.866025403784439,1.,0.866025403784439,1.,0.866025403784439,1.))
REPRESENTATION_ITEM('')
);
#173=(
BOUNDED_CURVE()
B_SPLINE_CURVE(2,(#5312,#5313,#5314,#5315,#5316,#5317,#5318,#5319,#5320,
#5321,#5322,#5323,#5324),.UNSPECIFIED.,.F.,.F.)
B_SPLINE_CURVE_WITH_KNOTS((3,2,2,2,2,2,3),(0.574074074074074,0.580246913580247,
0.58641975308642,0.592592592592593,0.598765432098765,0.604938271604938,
0.611111111111111),.UNSPECIFIED.)
CURVE()
GEOMETRIC_REPRESENTATION_ITEM()
RATIONAL_B_SPLINE_CURVE((1.,0.866025403784439,1.,0.866025403784439,1.,0.866025403784439,
1.,0.866025403784439,1.,0.866025403784439,1.,0.866025403784439,1.))
REPRESENTATION_ITEM('')
);
#174=(
BOUNDED_CURVE()
B_SPLINE_CURVE(2,(#5325,#5326,#5327,#5328,#5329,#5330,#5331,#5332,#5333,
#5334,#5335,#5336,#5337),.UNSPECIFIED.,.F.,.F.)
B_SPLINE_CURVE_WITH_KNOTS((3,2,2,2,2,2,3),(0.574074074074074,0.580246913580247,
0.58641975308642,0.592592592592593,0.598765432098765,0.604938271604938,
0.611111111111111),.UNSPECIFIED.)
CURVE()
GEOMETRIC_REPRESENTATION_ITEM()
RATIONAL_B_SPLINE_CURVE((1.,0.866025403784439,1.,0.866025403784439,1.,0.866025403784439,
1.,0.866025403784439,1.,0.866025403784439,1.,0.866025403784439,1.))
REPRESENTATION_ITEM('')
);
#175=(
BOUNDED_CURVE()
B_SPLINE_CURVE(2,(#5342,#5343,#5344,#5345,#5346,#5347,#5348,#5349,#5350,
#5351,#5352,#5353,#5354),.UNSPECIFIED.,.F.,.F.)
B_SPLINE_CURVE_WITH_KNOTS((3,2,2,2,2,2,3),(0.537037037037037,0.54320987654321,
0.549382716049383,0.555555555555556,0.561728395061728,0.567901234567901,
0.574074074074074),.UNSPECIFIED.)
CURVE()
GEOMETRIC_REPRESENTATION_ITEM()
RATIONAL_B_SPLINE_CURVE((1.,0.866025403784439,1.,0.866025403784439,1.,0.866025403784439,
1.,0.866025403784439,1.,0.866025403784439,1.,0.866025403784439,1.))
REPRESENTATION_ITEM('')
);
#176=(
BOUNDED_CURVE()
B_SPLINE_CURVE(2,(#5355,#5356,#5357,#5358,#5359,#5360,#5361,#5362,#5363,
#5364,#5365,#5366,#5367),.UNSPECIFIED.,.F.,.F.)
B_SPLINE_CURVE_WITH_KNOTS((3,2,2,2,2,2,3),(0.537037037037037,0.54320987654321,
0.549382716049383,0.555555555555556,0.561728395061728,0.567901234567901,
0.574074074074074),.UNSPECIFIED.)
CURVE()
GEOMETRIC_REPRESENTATION_ITEM()
RATIONAL_B_SPLINE_CURVE((1.,0.866025403784439,1.,0.866025403784439,1.,0.866025403784439,
1.,0.866025403784439,1.,0.866025403784439,1.,0.866025403784439,1.))
REPRESENTATION_ITEM('')
);
#177=(
BOUNDED_CURVE()
B_SPLINE_CURVE(2,(#5372,#5373,#5374,#5375,#5376,#5377,#5378,#5379,#5380,
#5381,#5382,#5383,#5384),.UNSPECIFIED.,.F.,.F.)
B_SPLINE_CURVE_WITH_KNOTS((3,2,2,2,2,2,3),(0.5,0.506172839506173,0.512345679012346,
0.518518518518518,0.524691358024691,0.530864197530864,0.537037037037037),
 .UNSPECIFIED.)
CURVE()
GEOMETRIC_REPRESENTATION_ITEM()
RATIONAL_B_SPLINE_CURVE((1.,0.866025403784439,1.,0.866025403784439,1.,0.866025403784439,
1.,0.866025403784439,1.,0.866025403784439,1.,0.866025403784439,1.))
REPRESENTATION_ITEM('')
);
#178=(
BOUNDED_CURVE()
B_SPLINE_CURVE(2,(#5385,#5386,#5387,#5388,#5389,#5390,#5391,#5392,#5393,
#5394,#5395,#5396,#5397),.UNSPECIFIED.,.F.,.F.)
B_SPLINE_CURVE_WITH_KNOTS((3,2,2,2,2,2,3),(0.5,0.506172839506173,0.512345679012346,
0.518518518518518,0.524691358024691,0.530864197530864,0.537037037037037),
 .UNSPECIFIED.)
CURVE()
GEOMETRIC_REPRESENTATION_ITEM()
RATIONAL_B_SPLINE_CURVE((1.,0.866025403784439,1.,0.866025403784439,1.,0.866025403784439,
1.,0.866025403784439,1.,0.866025403784439,1.,0.866025403784439,1.))
REPRESENTATION_ITEM('')
);
#179=(
BOUNDED_CURVE()
B_SPLINE_CURVE(2,(#5402,#5403,#5404,#5405,#5406,#5407,#5408,#5409,#5410,
#5411,#5412,#5413,#5414),.UNSPECIFIED.,.F.,.F.)
B_SPLINE_CURVE_WITH_KNOTS((3,2,2,2,2,2,3),(0.462962962962963,0.469135802469136,
0.475308641975309,0.481481481481481,0.487654320987654,0.493827160493827,
0.5),.UNSPECIFIED.)
CURVE()
GEOMETRIC_REPRESENTATION_ITEM()
RATIONAL_B_SPLINE_CURVE((1.,0.866025403784439,1.,0.866025403784439,1.,0.866025403784439,
1.,0.866025403784439,1.,0.866025403784439,1.,0.866025403784439,1.))
REPRESENTATION_ITEM('')
);
#180=(
BOUNDED_CURVE()
B_SPLINE_CURVE(2,(#5415,#5416,#5417,#5418,#5419,#5420,#5421,#5422,#5423,
#5424,#5425,#5426,#5427),.UNSPECIFIED.,.F.,.F.)
B_SPLINE_CURVE_WITH_KNOTS((3,2,2,2,2,2,3),(0.462962962962963,0.469135802469136,
0.475308641975309,0.481481481481481,0.487654320987654,0.493827160493827,
0.5),.UNSPECIFIED.)
CURVE()
GEOMETRIC_REPRESENTATION_ITEM()
RATIONAL_B_SPLINE_CURVE((1.,0.866025403784439,1.,0.866025403784439,1.,0.866025403784439,
1.,0.866025403784439,1.,0.866025403784439,1.,0.866025403784439,1.))
REPRESENTATION_ITEM('')
);
#181=(
BOUNDED_CURVE()
B_SPLINE_CURVE(2,(#5432,#5433,#5434,#5435,#5436,#5437,#5438,#5439,#5440,
#5441,#5442,#5443,#5444),.UNSPECIFIED.,.F.,.F.)
B_SPLINE_CURVE_WITH_KNOTS((3,2,2,2,2,2,3),(0.425925925925926,0.432098765432099,
0.438271604938272,0.444444444444444,0.450617283950617,0.45679012345679,
0.462962962962963),.UNSPECIFIED.)
CURVE()
GEOMETRIC_REPRESENTATION_ITEM()
RATIONAL_B_SPLINE_CURVE((1.,0.866025403784439,1.,0.866025403784439,1.,0.866025403784439,
1.,0.866025403784439,1.,0.866025403784439,1.,0.866025403784439,1.))
REPRESENTATION_ITEM('')
);
#182=(
BOUNDED_CURVE()
B_SPLINE_CURVE(2,(#5445,#5446,#5447,#5448,#5449,#5450,#5451,#5452,#5453,
#5454,#5455,#5456,#5457),.UNSPECIFIED.,.F.,.F.)
B_SPLINE_CURVE_WITH_KNOTS((3,2,2,2,2,2,3),(0.425925925925926,0.432098765432099,
0.438271604938272,0.444444444444444,0.450617283950617,0.45679012345679,
0.462962962962963),.UNSPECIFIED.)
CURVE()
GEOMETRIC_REPRESENTATION_ITEM()
RATIONAL_B_SPLINE_CURVE((1.,0.866025403784439,1.,0.866025403784439,1.,0.866025403784439,
1.,0.866025403784439,1.,0.866025403784439,1.,0.866025403784439,1.))
REPRESENTATION_ITEM('')
);
#183=(
BOUNDED_CURVE()
B_SPLINE_CURVE(2,(#5462,#5463,#5464,#5465,#5466,#5467,#5468,#5469,#5470,
#5471,#5472,#5473,#5474),.UNSPECIFIED.,.F.,.F.)
B_SPLINE_CURVE_WITH_KNOTS((3,2,2,2,2,2,3),(0.388888888888889,0.395061728395062,
0.401234567901235,0.407407407407407,0.41358024691358,0.419753086419753,
0.425925925925926),.UNSPECIFIED.)
CURVE()
GEOMETRIC_REPRESENTATION_ITEM()
RATIONAL_B_SPLINE_CURVE((1.,0.866025403784439,1.,0.866025403784439,1.,0.866025403784439,
1.,0.866025403784439,1.,0.866025403784439,1.,0.866025403784439,1.))
REPRESENTATION_ITEM('')
);
#184=(
BOUNDED_CURVE()
B_SPLINE_CURVE(2,(#5475,#5476,#5477,#5478,#5479,#5480,#5481,#5482,#5483,
#5484,#5485,#5486,#5487),.UNSPECIFIED.,.F.,.F.)
B_SPLINE_CURVE_WITH_KNOTS((3,2,2,2,2,2,3),(0.388888888888889,0.395061728395062,
0.401234567901235,0.407407407407407,0.41358024691358,0.419753086419753,
0.425925925925926),.UNSPECIFIED.)
CURVE()
GEOMETRIC_REPRESENTATION_ITEM()
RATIONAL_B_SPLINE_CURVE((1.,0.866025403784439,1.,0.866025403784439,1.,0.866025403784439,
1.,0.866025403784439,1.,0.866025403784439,1.,0.866025403784439,1.))
REPRESENTATION_ITEM('')
);
#185=(
BOUNDED_CURVE()
B_SPLINE_CURVE(2,(#5492,#5493,#5494,#5495,#5496,#5497,#5498,#5499,#5500,
#5501,#5502,#5503,#5504),.UNSPECIFIED.,.F.,.F.)
B_SPLINE_CURVE_WITH_KNOTS((3,2,2,2,2,2,3),(0.351851851851852,0.358024691358025,
0.364197530864198,0.37037037037037,0.376543209876543,0.382716049382716,
0.388888888888889),.UNSPECIFIED.)
CURVE()
GEOMETRIC_REPRESENTATION_ITEM()
RATIONAL_B_SPLINE_CURVE((1.,0.866025403784439,1.,0.866025403784439,1.,0.866025403784439,
1.,0.866025403784439,1.,0.866025403784439,1.,0.866025403784439,1.))
REPRESENTATION_ITEM('')
);
#186=(
BOUNDED_CURVE()
B_SPLINE_CURVE(2,(#5505,#5506,#5507,#5508,#5509,#5510,#5511,#5512,#5513,
#5514,#5515,#5516,#5517),.UNSPECIFIED.,.F.,.F.)
B_SPLINE_CURVE_WITH_KNOTS((3,2,2,2,2,2,3),(0.351851851851852,0.358024691358025,
0.364197530864198,0.37037037037037,0.376543209876543,0.382716049382716,
0.388888888888889),.UNSPECIFIED.)
CURVE()
GEOMETRIC_REPRESENTATION_ITEM()
RATIONAL_B_SPLINE_CURVE((1.,0.866025403784439,1.,0.866025403784439,1.,0.866025403784439,
1.,0.866025403784439,1.,0.866025403784439,1.,0.866025403784439,1.))
REPRESENTATION_ITEM('')
);
#187=(
BOUNDED_CURVE()
B_SPLINE_CURVE(2,(#5522,#5523,#5524,#5525,#5526,#5527,#5528,#5529,#5530,
#5531,#5532,#5533,#5534),.UNSPECIFIED.,.F.,.F.)
B_SPLINE_CURVE_WITH_KNOTS((3,2,2,2,2,2,3),(0.314814814814815,0.320987654320988,
0.327160493827161,0.333333333333333,0.339506172839506,0.345679012345679,
0.351851851851852),.UNSPECIFIED.)
CURVE()
GEOMETRIC_REPRESENTATION_ITEM()
RATIONAL_B_SPLINE_CURVE((1.,0.866025403784439,1.,0.866025403784439,1.,0.866025403784439,
1.,0.866025403784439,1.,0.866025403784439,1.,0.866025403784439,1.))
REPRESENTATION_ITEM('')
);
#188=(
BOUNDED_CURVE()
B_SPLINE_CURVE(2,(#5535,#5536,#5537,#5538,#5539,#5540,#5541,#5542,#5543,
#5544,#5545,#5546,#5547),.UNSPECIFIED.,.F.,.F.)
B_SPLINE_CURVE_WITH_KNOTS((3,2,2,2,2,2,3),(0.314814814814815,0.320987654320988,
0.327160493827161,0.333333333333333,0.339506172839506,0.345679012345679,
0.351851851851852),.UNSPECIFIED.)
CURVE()
GEOMETRIC_REPRESENTATION_ITEM()
RATIONAL_B_SPLINE_CURVE((1.,0.866025403784439,1.,0.866025403784439,1.,0.866025403784439,
1.,0.866025403784439,1.,0.866025403784439,1.,0.866025403784439,1.))
REPRESENTATION_ITEM('')
);
#189=(
BOUNDED_CURVE()
B_SPLINE_CURVE(2,(#5552,#5553,#5554,#5555,#5556,#5557,#5558,#5559,#5560,
#5561,#5562,#5563,#5564),.UNSPECIFIED.,.F.,.F.)
B_SPLINE_CURVE_WITH_KNOTS((3,2,2,2,2,2,3),(0.277777777777778,0.283950617283951,
0.290123456790123,0.296296296296296,0.302469135802469,0.308641975308642,
0.314814814814815),.UNSPECIFIED.)
CURVE()
GEOMETRIC_REPRESENTATION_ITEM()
RATIONAL_B_SPLINE_CURVE((1.,0.866025403784439,1.,0.866025403784439,1.,0.866025403784439,
1.,0.866025403784439,1.,0.866025403784439,1.,0.866025403784439,1.))
REPRESENTATION_ITEM('')
);
#190=(
BOUNDED_CURVE()
B_SPLINE_CURVE(2,(#5565,#5566,#5567,#5568,#5569,#5570,#5571,#5572,#5573,
#5574,#5575,#5576,#5577),.UNSPECIFIED.,.F.,.F.)
B_SPLINE_CURVE_WITH_KNOTS((3,2,2,2,2,2,3),(0.277777777777778,0.283950617283951,
0.290123456790123,0.296296296296296,0.302469135802469,0.308641975308642,
0.314814814814815),.UNSPECIFIED.)
CURVE()
GEOMETRIC_REPRESENTATION_ITEM()
RATIONAL_B_SPLINE_CURVE((1.,0.866025403784439,1.,0.866025403784439,1.,0.866025403784439,
1.,0.866025403784439,1.,0.866025403784439,1.,0.866025403784439,1.))
REPRESENTATION_ITEM('')
);
#191=(
BOUNDED_CURVE()
B_SPLINE_CURVE(2,(#5582,#5583,#5584,#5585,#5586,#5587,#5588,#5589,#5590,
#5591,#5592,#5593,#5594),.UNSPECIFIED.,.F.,.F.)
B_SPLINE_CURVE_WITH_KNOTS((3,2,2,2,2,2,3),(0.240740740740741,0.246913580246914,
0.253086419753086,0.259259259259259,0.265432098765432,0.271604938271605,
0.277777777777778),.UNSPECIFIED.)
CURVE()
GEOMETRIC_REPRESENTATION_ITEM()
RATIONAL_B_SPLINE_CURVE((1.,0.866025403784439,1.,0.866025403784439,1.,0.866025403784439,
1.,0.866025403784439,1.,0.866025403784439,1.,0.866025403784439,1.))
REPRESENTATION_ITEM('')
);
#192=(
BOUNDED_CURVE()
B_SPLINE_CURVE(2,(#5595,#5596,#5597,#5598,#5599,#5600,#5601,#5602,#5603,
#5604,#5605,#5606,#5607),.UNSPECIFIED.,.F.,.F.)
B_SPLINE_CURVE_WITH_KNOTS((3,2,2,2,2,2,3),(0.240740740740741,0.246913580246914,
0.253086419753086,0.259259259259259,0.265432098765432,0.271604938271605,
0.277777777777778),.UNSPECIFIED.)
CURVE()
GEOMETRIC_REPRESENTATION_ITEM()
RATIONAL_B_SPLINE_CURVE((1.,0.866025403784439,1.,0.866025403784439,1.,0.866025403784439,
1.,0.866025403784439,1.,0.866025403784439,1.,0.866025403784439,1.))
REPRESENTATION_ITEM('')
);
#193=(
BOUNDED_CURVE()
B_SPLINE_CURVE(2,(#5612,#5613,#5614,#5615,#5616,#5617,#5618,#5619,#5620,
#5621,#5622,#5623,#5624),.UNSPECIFIED.,.F.,.F.)
B_SPLINE_CURVE_WITH_KNOTS((3,2,2,2,2,2,3),(0.203703703703704,0.209876543209877,
0.216049382716049,0.222222222222222,0.228395061728395,0.234567901234568,
0.240740740740741),.UNSPECIFIED.)
CURVE()
GEOMETRIC_REPRESENTATION_ITEM()
RATIONAL_B_SPLINE_CURVE((1.,0.866025403784439,1.,0.866025403784439,1.,0.866025403784439,
1.,0.866025403784439,1.,0.866025403784439,1.,0.866025403784439,1.))
REPRESENTATION_ITEM('')
);
#194=(
BOUNDED_CURVE()
B_SPLINE_CURVE(2,(#5625,#5626,#5627,#5628,#5629,#5630,#5631,#5632,#5633,
#5634,#5635,#5636,#5637),.UNSPECIFIED.,.F.,.F.)
B_SPLINE_CURVE_WITH_KNOTS((3,2,2,2,2,2,3),(0.203703703703704,0.209876543209877,
0.216049382716049,0.222222222222222,0.228395061728395,0.234567901234568,
0.240740740740741),.UNSPECIFIED.)
CURVE()
GEOMETRIC_REPRESENTATION_ITEM()
RATIONAL_B_SPLINE_CURVE((1.,0.866025403784439,1.,0.866025403784439,1.,0.866025403784439,
1.,0.866025403784439,1.,0.866025403784439,1.,0.866025403784439,1.))
REPRESENTATION_ITEM('')
);
#195=(
BOUNDED_CURVE()
B_SPLINE_CURVE(2,(#5642,#5643,#5644,#5645,#5646,#5647,#5648,#5649,#5650,
#5651,#5652,#5653,#5654),.UNSPECIFIED.,.F.,.F.)
B_SPLINE_CURVE_WITH_KNOTS((3,2,2,2,2,2,3),(0.166666666666667,0.172839506172839,
0.179012345679012,0.185185185185185,0.191358024691358,0.197530864197531,
0.203703703703704),.UNSPECIFIED.)
CURVE()
GEOMETRIC_REPRESENTATION_ITEM()
RATIONAL_B_SPLINE_CURVE((1.,0.866025403784439,1.,0.866025403784439,1.,0.866025403784439,
1.,0.866025403784439,1.,0.866025403784439,1.,0.866025403784439,1.))
REPRESENTATION_ITEM('')
);
#196=(
BOUNDED_CURVE()
B_SPLINE_CURVE(2,(#5655,#5656,#5657,#5658,#5659,#5660,#5661,#5662,#5663,
#5664,#5665,#5666,#5667),.UNSPECIFIED.,.F.,.F.)
B_SPLINE_CURVE_WITH_KNOTS((3,2,2,2,2,2,3),(0.166666666666667,0.172839506172839,
0.179012345679012,0.185185185185185,0.191358024691358,0.197530864197531,
0.203703703703704),.UNSPECIFIED.)
CURVE()
GEOMETRIC_REPRESENTATION_ITEM()
RATIONAL_B_SPLINE_CURVE((1.,0.866025403784439,1.,0.866025403784439,1.,0.866025403784439,
1.,0.866025403784439,1.,0.866025403784439,1.,0.866025403784439,1.))
REPRESENTATION_ITEM('')
);
#197=(
BOUNDED_CURVE()
B_SPLINE_CURVE(2,(#5672,#5673,#5674,#5675,#5676,#5677,#5678,#5679,#5680,
#5681,#5682,#5683,#5684),.UNSPECIFIED.,.F.,.F.)
B_SPLINE_CURVE_WITH_KNOTS((3,2,2,2,2,2,3),(0.12962962962963,0.135802469135802,
0.141975308641975,0.148148148148148,0.154320987654321,0.160493827160494,
0.166666666666667),.UNSPECIFIED.)
CURVE()
GEOMETRIC_REPRESENTATION_ITEM()
RATIONAL_B_SPLINE_CURVE((1.,0.866025403784439,1.,0.866025403784439,1.,0.866025403784439,
1.,0.866025403784439,1.,0.866025403784439,1.,0.866025403784439,1.))
REPRESENTATION_ITEM('')
);
#198=(
BOUNDED_CURVE()
B_SPLINE_CURVE(2,(#5685,#5686,#5687,#5688,#5689,#5690,#5691,#5692,#5693,
#5694,#5695,#5696,#5697),.UNSPECIFIED.,.F.,.F.)
B_SPLINE_CURVE_WITH_KNOTS((3,2,2,2,2,2,3),(0.12962962962963,0.135802469135802,
0.141975308641975,0.148148148148148,0.154320987654321,0.160493827160494,
0.166666666666667),.UNSPECIFIED.)
CURVE()
GEOMETRIC_REPRESENTATION_ITEM()
RATIONAL_B_SPLINE_CURVE((1.,0.866025403784439,1.,0.866025403784439,1.,0.866025403784439,
1.,0.866025403784439,1.,0.866025403784439,1.,0.866025403784439,1.))
REPRESENTATION_ITEM('')
);
#199=(
BOUNDED_CURVE()
B_SPLINE_CURVE(2,(#5702,#5703,#5704,#5705,#5706,#5707,#5708,#5709,#5710,
#5711,#5712,#5713,#5714),.UNSPECIFIED.,.F.,.F.)
B_SPLINE_CURVE_WITH_KNOTS((3,2,2,2,2,2,3),(0.0925925925925926,0.0987654320987654,
0.104938271604938,0.111111111111111,0.117283950617284,0.123456790123457,
0.12962962962963),.UNSPECIFIED.)
CURVE()
GEOMETRIC_REPRESENTATION_ITEM()
RATIONAL_B_SPLINE_CURVE((1.,0.866025403784439,1.,0.866025403784439,1.,0.866025403784439,
1.,0.866025403784439,1.,0.866025403784439,1.,0.866025403784439,1.))
REPRESENTATION_ITEM('')
);
#200=(
BOUNDED_CURVE()
B_SPLINE_CURVE(2,(#5715,#5716,#5717,#5718,#5719,#5720,#5721,#5722,#5723,
#5724,#5725,#5726,#5727),.UNSPECIFIED.,.F.,.F.)
B_SPLINE_CURVE_WITH_KNOTS((3,2,2,2,2,2,3),(0.0925925925925926,0.0987654320987654,
0.104938271604938,0.111111111111111,0.117283950617284,0.123456790123457,
0.12962962962963),.UNSPECIFIED.)
CURVE()
GEOMETRIC_REPRESENTATION_ITEM()
RATIONAL_B_SPLINE_CURVE((1.,0.866025403784439,1.,0.866025403784439,1.,0.866025403784439,
1.,0.866025403784439,1.,0.866025403784439,1.,0.866025403784439,1.))
REPRESENTATION_ITEM('')
);
#201=(
BOUNDED_CURVE()
B_SPLINE_CURVE(2,(#5732,#5733,#5734,#5735,#5736,#5737,#5738,#5739,#5740,
#5741,#5742,#5743,#5744),.UNSPECIFIED.,.F.,.F.)
B_SPLINE_CURVE_WITH_KNOTS((3,2,2,2,2,2,3),(0.0555555555555556,0.0617283950617284,
0.0679012345679012,0.0740740740740741,0.0802469135802469,0.0864197530864197,
0.0925925925925926),.UNSPECIFIED.)
CURVE()
GEOMETRIC_REPRESENTATION_ITEM()
RATIONAL_B_SPLINE_CURVE((1.,0.866025403784439,1.,0.866025403784439,1.,0.866025403784439,
1.,0.866025403784439,1.,0.866025403784439,1.,0.866025403784439,1.))
REPRESENTATION_ITEM('')
);
#202=(
BOUNDED_CURVE()
B_SPLINE_CURVE(2,(#5745,#5746,#5747,#5748,#5749,#5750,#5751,#5752,#5753,
#5754,#5755,#5756,#5757),.UNSPECIFIED.,.F.,.F.)
B_SPLINE_CURVE_WITH_KNOTS((3,2,2,2,2,2,3),(0.0555555555555556,0.0617283950617284,
0.0679012345679012,0.0740740740740741,0.0802469135802469,0.0864197530864197,
0.0925925925925926),.UNSPECIFIED.)
CURVE()
GEOMETRIC_REPRESENTATION_ITEM()
RATIONAL_B_SPLINE_CURVE((1.,0.866025403784439,1.,0.866025403784439,1.,0.866025403784439,
1.,0.866025403784439,1.,0.866025403784439,1.,0.866025403784439,1.))
REPRESENTATION_ITEM('')
);
#203=(
BOUNDED_CURVE()
B_SPLINE_CURVE(2,(#5762,#5763,#5764,#5765,#5766,#5767,#5768,#5769,#5770,
#5771,#5772,#5773,#5774),.UNSPECIFIED.,.F.,.F.)
B_SPLINE_CURVE_WITH_KNOTS((3,2,2,2,2,2,3),(0.0185185185185185,0.0246913580246914,
0.0308641975308642,0.037037037037037,0.0432098765432099,0.0493827160493827,
0.0555555555555556),.UNSPECIFIED.)
CURVE()
GEOMETRIC_REPRESENTATION_ITEM()
RATIONAL_B_SPLINE_CURVE((1.,0.866025403784439,1.,0.866025403784439,1.,0.866025403784439,
1.,0.866025403784439,1.,0.866025403784439,1.,0.866025403784439,1.))
REPRESENTATION_ITEM('')
);
#204=(
BOUNDED_CURVE()
B_SPLINE_CURVE(2,(#5775,#5776,#5777,#5778,#5779,#5780,#5781,#5782,#5783,
#5784,#5785,#5786,#5787),.UNSPECIFIED.,.F.,.F.)
B_SPLINE_CURVE_WITH_KNOTS((3,2,2,2,2,2,3),(0.0185185185185185,0.0246913580246914,
0.0308641975308642,0.037037037037037,0.0432098765432099,0.0493827160493827,
0.0555555555555556),.UNSPECIFIED.)
CURVE()
GEOMETRIC_REPRESENTATION_ITEM()
RATIONAL_B_SPLINE_CURVE((1.,0.866025403784439,1.,0.866025403784439,1.,0.866025403784439,
1.,0.866025403784439,1.,0.866025403784439,1.,0.866025403784439,1.))
REPRESENTATION_ITEM('')
);
#205=(
BOUNDED_CURVE()
B_SPLINE_CURVE(2,(#8530,#8531,#8532,#8533,#8534,#8535,#8536),
 .UNSPECIFIED.,.F.,.F.)
B_SPLINE_CURVE_WITH_KNOTS((3,2,2,3),(0.,0.00617283950617284,0.0123456790123457,
0.0185185185185185),.UNSPECIFIED.)
CURVE()
GEOMETRIC_REPRESENTATION_ITEM()
RATIONAL_B_SPLINE_CURVE((1.,0.866025403784439,1.,0.866025403784439,1.,0.866025403784439,
1.))
REPRESENTATION_ITEM('')
);
#206=(
BOUNDED_CURVE()
B_SPLINE_CURVE(2,(#8538,#8539,#8540,#8541,#8542,#8543,#8544),
 .UNSPECIFIED.,.F.,.F.)
B_SPLINE_CURVE_WITH_KNOTS((3,2,2,3),(0.,0.00617283950617284,0.0123456790123457,
0.0185185185185185),.UNSPECIFIED.)
CURVE()
GEOMETRIC_REPRESENTATION_ITEM()
RATIONAL_B_SPLINE_CURVE((1.,0.866025403784439,1.,0.866025403784439,1.,0.866025403784439,
1.))
REPRESENTATION_ITEM('')
);
#223=SHAPE_REPRESENTATION_RELATIONSHIP('SRR','None',#14122,#232);
#232=ADVANCED_BREP_SHAPE_REPRESENTATION('',(#250),#14077);
#241=STYLED_ITEM('',(#14176),#250);
#250=MANIFOLD_SOLID_BREP('Body1',#3467);
#265=FACE_BOUND('',#673,.T.);
#266=FACE_BOUND('',#675,.T.);
#324=PLANE('',#3718);
#325=PLANE('',#3719);
#326=PLANE('',#3720);
#327=PLANE('',#3721);
#328=PLANE('',#3722);
#329=PLANE('',#3723);
#415=FACE_OUTER_BOUND('',#613,.T.);
#416=FACE_OUTER_BOUND('',#614,.T.);
#417=FACE_OUTER_BOUND('',#615,.T.);
#418=FACE_OUTER_BOUND('',#616,.T.);
#419=FACE_OUTER_BOUND('',#617,.T.);
#420=FACE_OUTER_BOUND('',#618,.T.);
#421=FACE_OUTER_BOUND('',#619,.T.);
#422=FACE_OUTER_BOUND('',#620,.T.);
#423=FACE_OUTER_BOUND('',#621,.T.);
#424=FACE_OUTER_BOUND('',#622,.T.);
#425=FACE_OUTER_BOUND('',#623,.T.);
#426=FACE_OUTER_BOUND('',#624,.T.);
#427=FACE_OUTER_BOUND('',#625,.T.);
#428=FACE_OUTER_BOUND('',#626,.T.);
#429=FACE_OUTER_BOUND('',#627,.T.);
#430=FACE_OUTER_BOUND('',#628,.T.);
#431=FACE_OUTER_BOUND('',#629,.T.);
#432=FACE_OUTER_BOUND('',#630,.T.);
#433=FACE_OUTER_BOUND('',#631,.T.);
#434=FACE_OUTER_BOUND('',#632,.T.);
#435=FACE_OUTER_BOUND('',#633,.T.);
#436=FACE_OUTER_BOUND('',#634,.T.);
#437=FACE_OUTER_BOUND('',#635,.T.);
#438=FACE_OUTER_BOUND('',#636,.T.);
#439=FACE_OUTER_BOUND('',#637,.T.);
#440=FACE_OUTER_BOUND('',#638,.T.);
#441=FACE_OUTER_BOUND('',#639,.T.);
#442=FACE_OUTER_BOUND('',#640,.T.);
#443=FACE_OUTER_BOUND('',#641,.T.);
#444=FACE_OUTER_BOUND('',#642,.T.);
#445=FACE_OUTER_BOUND('',#643,.T.);
#446=FACE_OUTER_BOUND('',#644,.T.);
#447=FACE_OUTER_BOUND('',#645,.T.);
#448=FACE_OUTER_BOUND('',#646,.T.);
#449=FACE_OUTER_BOUND('',#647,.T.);
#450=FACE_OUTER_BOUND('',#648,.T.);
#451=FACE_OUTER_BOUND('',#649,.T.);
#452=FACE_OUTER_BOUND('',#650,.T.);
#453=FACE_OUTER_BOUND('',#651,.T.);
#454=FACE_OUTER_BOUND('',#652,.T.);
#455=FACE_OUTER_BOUND('',#653,.T.);
#456=FACE_OUTER_BOUND('',#654,.T.);
#457=FACE_OUTER_BOUND('',#655,.T.);
#458=FACE_OUTER_BOUND('',#656,.T.);
#459=FACE_OUTER_BOUND('',#657,.T.);
#460=FACE_OUTER_BOUND('',#658,.T.);
#461=FACE_OUTER_BOUND('',#659,.T.);
#462=FACE_OUTER_BOUND('',#660,.T.);
#463=FACE_OUTER_BOUND('',#661,.T.);
#464=FACE_OUTER_BOUND('',#662,.T.);
#465=FACE_OUTER_BOUND('',#663,.T.);
#466=FACE_OUTER_BOUND('',#664,.T.);
#467=FACE_OUTER_BOUND('',#665,.T.);
#468=FACE_OUTER_BOUND('',#666,.T.);
#469=FACE_OUTER_BOUND('',#667,.T.);
#470=FACE_OUTER_BOUND('',#668,.T.);
#471=FACE_OUTER_BOUND('',#669,.T.);
#472=FACE_OUTER_BOUND('',#670,.T.);
#473=FACE_OUTER_BOUND('',#671,.T.);
#474=FACE_OUTER_BOUND('',#672,.T.);
#475=FACE_OUTER_BOUND('',#674,.T.);
#476=FACE_OUTER_BOUND('',#676,.T.);
#477=FACE_OUTER_BOUND('',#677,.T.);
#478=FACE_OUTER_BOUND('',#678,.T.);
#479=FACE_OUTER_BOUND('',#679,.T.);
#480=FACE_OUTER_BOUND('',#680,.T.);
#481=FACE_OUTER_BOUND('',#681,.T.);
#613=EDGE_LOOP('',(#2485,#2486,#2487,#2488));
#614=EDGE_LOOP('',(#2489,#2490,#2491,#2492));
#615=EDGE_LOOP('',(#2493,#2494,#2495,#2496));
#616=EDGE_LOOP('',(#2497,#2498,#2499,#2500));
#617=EDGE_LOOP('',(#2501,#2502,#2503,#2504));
#618=EDGE_LOOP('',(#2505,#2506,#2507,#2508));
#619=EDGE_LOOP('',(#2509,#2510,#2511,#2512));
#620=EDGE_LOOP('',(#2513,#2514,#2515,#2516));
#621=EDGE_LOOP('',(#2517,#2518,#2519,#2520));
#622=EDGE_LOOP('',(#2521,#2522,#2523,#2524));
#623=EDGE_LOOP('',(#2525,#2526,#2527,#2528));
#624=EDGE_LOOP('',(#2529,#2530,#2531,#2532));
#625=EDGE_LOOP('',(#2533,#2534,#2535,#2536));
#626=EDGE_LOOP('',(#2537,#2538,#2539,#2540));
#627=EDGE_LOOP('',(#2541,#2542,#2543,#2544));
#628=EDGE_LOOP('',(#2545,#2546,#2547,#2548));
#629=EDGE_LOOP('',(#2549,#2550,#2551,#2552));
#630=EDGE_LOOP('',(#2553,#2554,#2555,#2556));
#631=EDGE_LOOP('',(#2557,#2558,#2559,#2560));
#632=EDGE_LOOP('',(#2561,#2562,#2563,#2564));
#633=EDGE_LOOP('',(#2565,#2566,#2567,#2568));
#634=EDGE_LOOP('',(#2569,#2570,#2571,#2572));
#635=EDGE_LOOP('',(#2573,#2574,#2575,#2576));
#636=EDGE_LOOP('',(#2577,#2578,#2579,#2580));
#637=EDGE_LOOP('',(#2581,#2582,#2583,#2584));
#638=EDGE_LOOP('',(#2585,#2586,#2587,#2588));
#639=EDGE_LOOP('',(#2589,#2590,#2591,#2592));
#640=EDGE_LOOP('',(#2593,#2594,#2595));
#641=EDGE_LOOP('',(#2596,#2597,#2598,#2599,#2600,#2601));
#642=EDGE_LOOP('',(#2602,#2603,#2604,#2605));
#643=EDGE_LOOP('',(#2606,#2607,#2608,#2609));
#644=EDGE_LOOP('',(#2610,#2611,#2612,#2613));
#645=EDGE_LOOP('',(#2614,#2615,#2616,#2617));
#646=EDGE_LOOP('',(#2618,#2619,#2620,#2621));
#647=EDGE_LOOP('',(#2622,#2623,#2624,#2625));
#648=EDGE_LOOP('',(#2626,#2627,#2628,#2629));
#649=EDGE_LOOP('',(#2630,#2631,#2632,#2633));
#650=EDGE_LOOP('',(#2634,#2635,#2636,#2637));
#651=EDGE_LOOP('',(#2638,#2639,#2640,#2641));
#652=EDGE_LOOP('',(#2642,#2643,#2644,#2645));
#653=EDGE_LOOP('',(#2646,#2647,#2648,#2649));
#654=EDGE_LOOP('',(#2650,#2651,#2652,#2653));
#655=EDGE_LOOP('',(#2654,#2655,#2656,#2657));
#656=EDGE_LOOP('',(#2658,#2659,#2660,#2661));
#657=EDGE_LOOP('',(#2662,#2663,#2664,#2665));
#658=EDGE_LOOP('',(#2666,#2667,#2668,#2669));
#659=EDGE_LOOP('',(#2670,#2671,#2672,#2673));
#660=EDGE_LOOP('',(#2674,#2675,#2676,#2677));
#661=EDGE_LOOP('',(#2678,#2679,#2680,#2681));
#662=EDGE_LOOP('',(#2682,#2683,#2684,#2685));
#663=EDGE_LOOP('',(#2686,#2687,#2688,#2689));
#664=EDGE_LOOP('',(#2690,#2691,#2692,#2693));
#665=EDGE_LOOP('',(#2694,#2695,#2696,#2697));
#666=EDGE_LOOP('',(#2698,#2699,#2700,#2701,#2702,#2703,#2704,#2705));
#667=EDGE_LOOP('',(#2706,#2707,#2708,#2709,#2710));
#668=EDGE_LOOP('',(#2711,#2712,#2713,#2714));
#669=EDGE_LOOP('',(#2715,#2716,#2717,#2718));
#670=EDGE_LOOP('',(#2719,#2720,#2721,#2722,#2723));
#671=EDGE_LOOP('',(#2724));
#672=EDGE_LOOP('',(#2725));
#673=EDGE_LOOP('',(#2726));
#674=EDGE_LOOP('',(#2727));
#675=EDGE_LOOP('',(#2728));
#676=EDGE_LOOP('',(#2729,#2730));
#677=EDGE_LOOP('',(#2731,#2732,#2733,#2734));
#678=EDGE_LOOP('',(#2735,#2736,#2737,#2738));
#679=EDGE_LOOP('',(#2739,#2740,#2741,#2742,#2743,#2744,#2745,#2746,#2747,
#2748,#2749,#2750,#2751,#2752,#2753,#2754,#2755,#2756,#2757,#2758,#2759,
#2760,#2761,#2762,#2763,#2764,#2765,#2766,#2767,#2768,#2769,#2770,#2771,
#2772,#2773,#2774,#2775,#2776,#2777,#2778,#2779,#2780,#2781,#2782,#2783,
#2784,#2785,#2786,#2787,#2788,#2789,#2790,#2791,#2792,#2793,#2794,#2795,
#2796));
#680=EDGE_LOOP('',(#2797,#2798,#2799,#2800));
#681=EDGE_LOOP('',(#2801,#2802,#2803,#2804,#2805,#2806,#2807,#2808,#2809,
#2810,#2811,#2812,#2813,#2814,#2815,#2816,#2817,#2818,#2819,#2820,#2821,
#2822,#2823,#2824,#2825,#2826,#2827,#2828,#2829,#2830,#2831,#2832,#2833,
#2834,#2835,#2836,#2837,#2838,#2839,#2840,#2841,#2842,#2843,#2844,#2845,
#2846,#2847,#2848,#2849,#2850,#2851,#2852,#2853,#2854,#2855,#2856,#2857,
#2858));
#895=LINE('',#4998,#1152);
#896=LINE('',#5004,#1153);
#897=LINE('',#5011,#1154);
#898=LINE('',#5041,#1155);
#899=LINE('',#5071,#1156);
#900=LINE('',#5101,#1157);
#901=LINE('',#5131,#1158);
#902=LINE('',#5161,#1159);
#903=LINE('',#5191,#1160);
#904=LINE('',#5221,#1161);
#905=LINE('',#5251,#1162);
#906=LINE('',#5281,#1163);
#907=LINE('',#5311,#1164);
#908=LINE('',#5341,#1165);
#909=LINE('',#5371,#1166);
#910=LINE('',#5401,#1167);
#911=LINE('',#5431,#1168);
#912=LINE('',#5461,#1169);
#913=LINE('',#5491,#1170);
#914=LINE('',#5521,#1171);
#915=LINE('',#5551,#1172);
#916=LINE('',#5581,#1173);
#917=LINE('',#5611,#1174);
#918=LINE('',#5641,#1175);
#919=LINE('',#5671,#1176);
#920=LINE('',#5701,#1177);
#921=LINE('',#5731,#1178);
#922=LINE('',#5761,#1179);
#923=LINE('',#5791,#1180);
#924=LINE('',#5809,#1181);
#925=LINE('',#5848,#1182);
#926=LINE('',#5864,#1183);
#927=LINE('',#5940,#1184);
#928=LINE('',#6018,#1185);
#929=LINE('',#6096,#1186);
#930=LINE('',#6172,#1187);
#931=LINE('',#6248,#1188);
#932=LINE('',#6324,#1189);
#933=LINE('',#6402,#1190);
#934=LINE('',#6478,#1191);
#935=LINE('',#6556,#1192);
#936=LINE('',#6632,#1193);
#937=LINE('',#6708,#1194);
#938=LINE('',#6784,#1195);
#939=LINE('',#6860,#1196);
#940=LINE('',#6938,#1197);
#941=LINE('',#7016,#1198);
#942=LINE('',#7092,#1199);
#943=LINE('',#7168,#1200);
#944=LINE('',#7244,#1201);
#945=LINE('',#7322,#1202);
#946=LINE('',#7400,#1203);
#947=LINE('',#7476,#1204);
#948=LINE('',#7552,#1205);
#949=LINE('',#7628,#1206);
#950=LINE('',#7705,#1207);
#951=LINE('',#7724,#1208);
#952=LINE('',#7745,#1209);
#953=LINE('',#7869,#1210);
#954=LINE('',#7873,#1211);
#955=LINE('',#7881,#1212);
#956=LINE('',#7883,#1213);
#957=LINE('',#7884,#1214);
#958=LINE('',#7886,#1215);
#959=LINE('',#7887,#1216);
#1152=VECTOR('',#4140,5.75643035625);
#1153=VECTOR('',#4141,10.);
#1154=VECTOR('',#4144,5.75643035625);
#1155=VECTOR('',#4147,5.75643035625);
#1156=VECTOR('',#4150,5.75643035625);
#1157=VECTOR('',#4153,5.75643035625);
#1158=VECTOR('',#4156,5.75643035625);
#1159=VECTOR('',#4159,5.75643035625);
#1160=VECTOR('',#4162,5.75643035625);
#1161=VECTOR('',#4165,5.75643035625);
#1162=VECTOR('',#4168,5.75643035625);
#1163=VECTOR('',#4171,5.75643035625);
#1164=VECTOR('',#4174,5.75643035625);
#1165=VECTOR('',#4177,5.75643035625);
#1166=VECTOR('',#4180,5.75643035625);
#1167=VECTOR('',#4183,5.75643035625);
#1168=VECTOR('',#4186,5.75643035625);
#1169=VECTOR('',#4189,5.75643035625);
#1170=VECTOR('',#4192,5.75643035625);
#1171=VECTOR('',#4195,5.75643035625);
#1172=VECTOR('',#4198,5.75643035625);
#1173=VECTOR('',#4201,5.75643035625);
#1174=VECTOR('',#4204,5.75643035625);
#1175=VECTOR('',#4207,5.75643035625);
#1176=VECTOR('',#4210,5.75643035625);
#1177=VECTOR('',#4213,5.75643035625);
#1178=VECTOR('',#4216,5.75643035625);
#1179=VECTOR('',#4219,5.75643035625);
#1180=VECTOR('',#4222,6.);
#1181=VECTOR('',#4227,6.);
#1182=VECTOR('',#4230,1000.);
#1183=VECTOR('',#4233,6.);
#1184=VECTOR('',#4236,6.);
#1185=VECTOR('',#4239,6.);
#1186=VECTOR('',#4242,6.);
#1187=VECTOR('',#4245,6.);
#1188=VECTOR('',#4248,6.);
#1189=VECTOR('',#4251,6.);
#1190=VECTOR('',#4254,6.);
#1191=VECTOR('',#4257,6.);
#1192=VECTOR('',#4260,6.);
#1193=VECTOR('',#4263,6.);
#1194=VECTOR('',#4266,6.);
#1195=VECTOR('',#4269,6.);
#1196=VECTOR('',#4272,6.);
#1197=VECTOR('',#4275,6.);
#1198=VECTOR('',#4278,6.);
#1199=VECTOR('',#4281,6.);
#1200=VECTOR('',#4284,6.);
#1201=VECTOR('',#4287,6.);
#1202=VECTOR('',#4290,6.);
#1203=VECTOR('',#4293,6.);
#1204=VECTOR('',#4296,6.);
#1205=VECTOR('',#4299,6.);
#1206=VECTOR('',#4302,6.);
#1207=VECTOR('',#4307,6.);
#1208=VECTOR('',#4308,1000.);
#1209=VECTOR('',#4309,6.);
#1210=VECTOR('',#4326,9.);
#1211=VECTOR('',#4331,6.);
#1212=VECTOR('',#4344,1000.);
#1213=VECTOR('',#4345,1000.);
#1214=VECTOR('',#4346,1000.);
#1215=VECTOR('',#4349,10.);
#1216=VECTOR('',#4350,10.);
#1309=CIRCLE('',#3678,6.);
#1310=CIRCLE('',#3680,6.);
#1311=CIRCLE('',#3706,6.);
#1312=CIRCLE('',#3708,6.00000000000001);
#1313=CIRCLE('',#3709,26.5);
#1314=CIRCLE('',#3710,6.);
#1315=CIRCLE('',#3711,6.);
#1316=CIRCLE('',#3714,9.);
#1317=CIRCLE('',#3715,9.);
#1318=CIRCLE('',#3717,6.);
#1473=VERTEX_POINT('',#4996);
#1474=VERTEX_POINT('',#4997);
#1475=VERTEX_POINT('',#4999);
#1476=VERTEX_POINT('',#5003);
#1477=VERTEX_POINT('',#5009);
#1478=VERTEX_POINT('',#5010);
#1479=VERTEX_POINT('',#5039);
#1480=VERTEX_POINT('',#5040);
#1481=VERTEX_POINT('',#5069);
#1482=VERTEX_POINT('',#5070);
#1483=VERTEX_POINT('',#5099);
#1484=VERTEX_POINT('',#5100);
#1485=VERTEX_POINT('',#5129);
#1486=VERTEX_POINT('',#5130);
#1487=VERTEX_POINT('',#5159);
#1488=VERTEX_POINT('',#5160);
#1489=VERTEX_POINT('',#5189);
#1490=VERTEX_POINT('',#5190);
#1491=VERTEX_POINT('',#5219);
#1492=VERTEX_POINT('',#5220);
#1493=VERTEX_POINT('',#5249);
#1494=VERTEX_POINT('',#5250);
#1495=VERTEX_POINT('',#5279);
#1496=VERTEX_POINT('',#5280);
#1497=VERTEX_POINT('',#5309);
#1498=VERTEX_POINT('',#5310);
#1499=VERTEX_POINT('',#5339);
#1500=VERTEX_POINT('',#5340);
#1501=VERTEX_POINT('',#5369);
#1502=VERTEX_POINT('',#5370);
#1503=VERTEX_POINT('',#5399);
#1504=VERTEX_POINT('',#5400);
#1505=VERTEX_POINT('',#5429);
#1506=VERTEX_POINT('',#5430);
#1507=VERTEX_POINT('',#5459);
#1508=VERTEX_POINT('',#5460);
#1509=VERTEX_POINT('',#5489);
#1510=VERTEX_POINT('',#5490);
#1511=VERTEX_POINT('',#5519);
#1512=VERTEX_POINT('',#5520);
#1513=VERTEX_POINT('',#5549);
#1514=VERTEX_POINT('',#5550);
#1515=VERTEX_POINT('',#5579);
#1516=VERTEX_POINT('',#5580);
#1517=VERTEX_POINT('',#5609);
#1518=VERTEX_POINT('',#5610);
#1519=VERTEX_POINT('',#5639);
#1520=VERTEX_POINT('',#5640);
#1521=VERTEX_POINT('',#5669);
#1522=VERTEX_POINT('',#5670);
#1523=VERTEX_POINT('',#5699);
#1524=VERTEX_POINT('',#5700);
#1525=VERTEX_POINT('',#5729);
#1526=VERTEX_POINT('',#5730);
#1527=VERTEX_POINT('',#5759);
#1528=VERTEX_POINT('',#5760);
#1529=VERTEX_POINT('',#5789);
#1530=VERTEX_POINT('',#5790);
#1531=VERTEX_POINT('',#5792);
#1532=VERTEX_POINT('',#5807);
#1533=VERTEX_POINT('',#5808);
#1534=VERTEX_POINT('',#5847);
#1535=VERTEX_POINT('',#5862);
#1536=VERTEX_POINT('',#5863);
#1537=VERTEX_POINT('',#5938);
#1538=VERTEX_POINT('',#5939);
#1539=VERTEX_POINT('',#6016);
#1540=VERTEX_POINT('',#6017);
#1541=VERTEX_POINT('',#6094);
#1542=VERTEX_POINT('',#6095);
#1543=VERTEX_POINT('',#6170);
#1544=VERTEX_POINT('',#6171);
#1545=VERTEX_POINT('',#6246);
#1546=VERTEX_POINT('',#6247);
#1547=VERTEX_POINT('',#6322);
#1548=VERTEX_POINT('',#6323);
#1549=VERTEX_POINT('',#6400);
#1550=VERTEX_POINT('',#6401);
#1551=VERTEX_POINT('',#6476);
#1552=VERTEX_POINT('',#6477);
#1553=VERTEX_POINT('',#6554);
#1554=VERTEX_POINT('',#6555);
#1555=VERTEX_POINT('',#6630);
#1556=VERTEX_POINT('',#6631);
#1557=VERTEX_POINT('',#6706);
#1558=VERTEX_POINT('',#6707);
#1559=VERTEX_POINT('',#6782);
#1560=VERTEX_POINT('',#6783);
#1561=VERTEX_POINT('',#6858);
#1562=VERTEX_POINT('',#6859);
#1563=VERTEX_POINT('',#6936);
#1564=VERTEX_POINT('',#6937);
#1565=VERTEX_POINT('',#7014);
#1566=VERTEX_POINT('',#7015);
#1567=VERTEX_POINT('',#7090);
#1568=VERTEX_POINT('',#7091);
#1569=VERTEX_POINT('',#7166);
#1570=VERTEX_POINT('',#7167);
#1571=VERTEX_POINT('',#7242);
#1572=VERTEX_POINT('',#7243);
#1573=VERTEX_POINT('',#7320);
#1574=VERTEX_POINT('',#7321);
#1575=VERTEX_POINT('',#7398);
#1576=VERTEX_POINT('',#7399);
#1577=VERTEX_POINT('',#7474);
#1578=VERTEX_POINT('',#7475);
#1579=VERTEX_POINT('',#7550);
#1580=VERTEX_POINT('',#7551);
#1581=VERTEX_POINT('',#7626);
#1582=VERTEX_POINT('',#7627);
#1583=VERTEX_POINT('',#7702);
#1584=VERTEX_POINT('',#7704);
#1585=VERTEX_POINT('',#7706);
#1586=VERTEX_POINT('',#7723);
#1587=VERTEX_POINT('',#7725);
#1588=VERTEX_POINT('',#7744);
#1589=VERTEX_POINT('',#7783);
#1590=VERTEX_POINT('',#7785);
#1591=VERTEX_POINT('',#7787);
#1592=VERTEX_POINT('',#7866);
#1593=VERTEX_POINT('',#7868);
#1594=VERTEX_POINT('',#7872);
#1595=VERTEX_POINT('',#7880);
#1596=VERTEX_POINT('',#7882);
#1846=EDGE_CURVE('',#1473,#1474,#895,.T.);
#1847=EDGE_CURVE('',#1473,#1475,#151,.T.);
#1848=EDGE_CURVE('',#1475,#1476,#896,.T.);
#1849=EDGE_CURVE('',#1474,#1476,#152,.T.);
#1850=EDGE_CURVE('',#1477,#1478,#897,.T.);
#1851=EDGE_CURVE('',#1477,#1473,#153,.T.);
#1852=EDGE_CURVE('',#1478,#1474,#154,.T.);
#1853=EDGE_CURVE('',#1479,#1480,#898,.T.);
#1854=EDGE_CURVE('',#1479,#1477,#155,.T.);
#1855=EDGE_CURVE('',#1480,#1478,#156,.T.);
#1856=EDGE_CURVE('',#1481,#1482,#899,.T.);
#1857=EDGE_CURVE('',#1481,#1479,#157,.T.);
#1858=EDGE_CURVE('',#1482,#1480,#158,.T.);
#1859=EDGE_CURVE('',#1483,#1484,#900,.T.);
#1860=EDGE_CURVE('',#1483,#1481,#159,.T.);
#1861=EDGE_CURVE('',#1484,#1482,#160,.T.);
#1862=EDGE_CURVE('',#1485,#1486,#901,.T.);
#1863=EDGE_CURVE('',#1485,#1483,#161,.T.);
#1864=EDGE_CURVE('',#1486,#1484,#162,.T.);
#1865=EDGE_CURVE('',#1487,#1488,#902,.T.);
#1866=EDGE_CURVE('',#1487,#1485,#163,.T.);
#1867=EDGE_CURVE('',#1488,#1486,#164,.T.);
#1868=EDGE_CURVE('',#1489,#1490,#903,.T.);
#1869=EDGE_CURVE('',#1489,#1487,#165,.T.);
#1870=EDGE_CURVE('',#1490,#1488,#166,.T.);
#1871=EDGE_CURVE('',#1491,#1492,#904,.T.);
#1872=EDGE_CURVE('',#1491,#1489,#167,.T.);
#1873=EDGE_CURVE('',#1492,#1490,#168,.T.);
#1874=EDGE_CURVE('',#1493,#1494,#905,.T.);
#1875=EDGE_CURVE('',#1493,#1491,#169,.T.);
#1876=EDGE_CURVE('',#1494,#1492,#170,.T.);
#1877=EDGE_CURVE('',#1495,#1496,#906,.T.);
#1878=EDGE_CURVE('',#1495,#1493,#171,.T.);
#1879=EDGE_CURVE('',#1496,#1494,#172,.T.);
#1880=EDGE_CURVE('',#1497,#1498,#907,.T.);
#1881=EDGE_CURVE('',#1497,#1495,#173,.T.);
#1882=EDGE_CURVE('',#1498,#1496,#174,.T.);
#1883=EDGE_CURVE('',#1499,#1500,#908,.T.);
#1884=EDGE_CURVE('',#1499,#1497,#175,.T.);
#1885=EDGE_CURVE('',#1500,#1498,#176,.T.);
#1886=EDGE_CURVE('',#1501,#1502,#909,.T.);
#1887=EDGE_CURVE('',#1501,#1499,#177,.T.);
#1888=EDGE_CURVE('',#1502,#1500,#178,.T.);
#1889=EDGE_CURVE('',#1503,#1504,#910,.T.);
#1890=EDGE_CURVE('',#1503,#1501,#179,.T.);
#1891=EDGE_CURVE('',#1504,#1502,#180,.T.);
#1892=EDGE_CURVE('',#1505,#1506,#911,.T.);
#1893=EDGE_CURVE('',#1505,#1503,#181,.T.);
#1894=EDGE_CURVE('',#1506,#1504,#182,.T.);
#1895=EDGE_CURVE('',#1507,#1508,#912,.T.);
#1896=EDGE_CURVE('',#1507,#1505,#183,.T.);
#1897=EDGE_CURVE('',#1508,#1506,#184,.T.);
#1898=EDGE_CURVE('',#1509,#1510,#913,.T.);
#1899=EDGE_CURVE('',#1509,#1507,#185,.T.);
#1900=EDGE_CURVE('',#1510,#1508,#186,.T.);
#1901=EDGE_CURVE('',#1511,#1512,#914,.T.);
#1902=EDGE_CURVE('',#1511,#1509,#187,.T.);
#1903=EDGE_CURVE('',#1512,#1510,#188,.T.);
#1904=EDGE_CURVE('',#1513,#1514,#915,.T.);
#1905=EDGE_CURVE('',#1513,#1511,#189,.T.);
#1906=EDGE_CURVE('',#1514,#1512,#190,.T.);
#1907=EDGE_CURVE('',#1515,#1516,#916,.T.);
#1908=EDGE_CURVE('',#1515,#1513,#191,.T.);
#1909=EDGE_CURVE('',#1516,#1514,#192,.T.);
#1910=EDGE_CURVE('',#1517,#1518,#917,.T.);
#1911=EDGE_CURVE('',#1517,#1515,#193,.T.);
#1912=EDGE_CURVE('',#1518,#1516,#194,.T.);
#1913=EDGE_CURVE('',#1519,#1520,#918,.T.);
#1914=EDGE_CURVE('',#1519,#1517,#195,.T.);
#1915=EDGE_CURVE('',#1520,#1518,#196,.T.);
#1916=EDGE_CURVE('',#1521,#1522,#919,.T.);
#1917=EDGE_CURVE('',#1521,#1519,#197,.T.);
#1918=EDGE_CURVE('',#1522,#1520,#198,.T.);
#1919=EDGE_CURVE('',#1523,#1524,#920,.T.);
#1920=EDGE_CURVE('',#1523,#1521,#199,.T.);
#1921=EDGE_CURVE('',#1524,#1522,#200,.T.);
#1922=EDGE_CURVE('',#1525,#1526,#921,.T.);
#1923=EDGE_CURVE('',#1525,#1523,#201,.T.);
#1924=EDGE_CURVE('',#1526,#1524,#202,.T.);
#1925=EDGE_CURVE('',#1527,#1528,#922,.T.);
#1926=EDGE_CURVE('',#1527,#1525,#203,.T.);
#1927=EDGE_CURVE('',#1528,#1526,#204,.T.);
#1928=EDGE_CURVE('',#1529,#1530,#923,.T.);
#1929=EDGE_CURVE('',#1531,#1529,#73,.F.);
#1930=EDGE_CURVE('',#1530,#1531,#1309,.T.);
#1931=EDGE_CURVE('',#1532,#1533,#924,.T.);
#1932=EDGE_CURVE('',#1529,#1532,#74,.F.);
#1933=EDGE_CURVE('',#1531,#1530,#1310,.T.);
#1934=EDGE_CURVE('',#1531,#1534,#925,.T.);
#1935=EDGE_CURVE('',#1534,#1533,#75,.T.);
#1936=EDGE_CURVE('',#1535,#1536,#926,.T.);
#1937=EDGE_CURVE('',#1532,#1535,#76,.F.);
#1938=EDGE_CURVE('',#1533,#1536,#77,.T.);
#1939=EDGE_CURVE('',#1537,#1538,#927,.T.);
#1940=EDGE_CURVE('',#1535,#1537,#78,.F.);
#1941=EDGE_CURVE('',#1536,#1538,#79,.T.);
#1942=EDGE_CURVE('',#1539,#1540,#928,.T.);
#1943=EDGE_CURVE('',#1537,#1539,#80,.F.);
#1944=EDGE_CURVE('',#1538,#1540,#81,.T.);
#1945=EDGE_CURVE('',#1541,#1542,#929,.T.);
#1946=EDGE_CURVE('',#1539,#1541,#82,.F.);
#1947=EDGE_CURVE('',#1540,#1542,#83,.T.);
#1948=EDGE_CURVE('',#1543,#1544,#930,.T.);
#1949=EDGE_CURVE('',#1541,#1543,#84,.F.);
#1950=EDGE_CURVE('',#1542,#1544,#85,.T.);
#1951=EDGE_CURVE('',#1545,#1546,#931,.T.);
#1952=EDGE_CURVE('',#1543,#1545,#86,.F.);
#1953=EDGE_CURVE('',#1544,#1546,#87,.T.);
#1954=EDGE_CURVE('',#1547,#1548,#932,.T.);
#1955=EDGE_CURVE('',#1545,#1547,#88,.F.);
#1956=EDGE_CURVE('',#1546,#1548,#89,.T.);
#1957=EDGE_CURVE('',#1549,#1550,#933,.T.);
#1958=EDGE_CURVE('',#1547,#1549,#90,.F.);
#1959=EDGE_CURVE('',#1548,#1550,#91,.T.);
#1960=EDGE_CURVE('',#1551,#1552,#934,.T.);
#1961=EDGE_CURVE('',#1549,#1551,#92,.F.);
#1962=EDGE_CURVE('',#1550,#1552,#93,.T.);
#1963=EDGE_CURVE('',#1553,#1554,#935,.T.);
#1964=EDGE_CURVE('',#1551,#1553,#94,.F.);
#1965=EDGE_CURVE('',#1552,#1554,#95,.T.);
#1966=EDGE_CURVE('',#1555,#1556,#936,.T.);
#1967=EDGE_CURVE('',#1553,#1555,#96,.F.);
#1968=EDGE_CURVE('',#1554,#1556,#97,.T.);
#1969=EDGE_CURVE('',#1557,#1558,#937,.T.);
#1970=EDGE_CURVE('',#1555,#1557,#98,.F.);
#1971=EDGE_CURVE('',#1556,#1558,#99,.T.);
#1972=EDGE_CURVE('',#1559,#1560,#938,.T.);
#1973=EDGE_CURVE('',#1557,#1559,#100,.F.);
#1974=EDGE_CURVE('',#1558,#1560,#101,.T.);
#1975=EDGE_CURVE('',#1561,#1562,#939,.T.);
#1976=EDGE_CURVE('',#1559,#1561,#102,.F.);
#1977=EDGE_CURVE('',#1560,#1562,#103,.T.);
#1978=EDGE_CURVE('',#1563,#1564,#940,.T.);
#1979=EDGE_CURVE('',#1561,#1563,#104,.F.);
#1980=EDGE_CURVE('',#1562,#1564,#105,.T.);
#1981=EDGE_CURVE('',#1565,#1566,#941,.T.);
#1982=EDGE_CURVE('',#1563,#1565,#106,.F.);
#1983=EDGE_CURVE('',#1564,#1566,#107,.T.);
#1984=EDGE_CURVE('',#1567,#1568,#942,.T.);
#1985=EDGE_CURVE('',#1565,#1567,#108,.F.);
#1986=EDGE_CURVE('',#1566,#1568,#109,.T.);
#1987=EDGE_CURVE('',#1569,#1570,#943,.T.);
#1988=EDGE_CURVE('',#1567,#1569,#110,.F.);
#1989=EDGE_CURVE('',#1568,#1570,#111,.T.);
#1990=EDGE_CURVE('',#1571,#1572,#944,.T.);
#1991=EDGE_CURVE('',#1569,#1571,#112,.F.);
#1992=EDGE_CURVE('',#1570,#1572,#113,.T.);
#1993=EDGE_CURVE('',#1573,#1574,#945,.T.);
#1994=EDGE_CURVE('',#1571,#1573,#114,.F.);
#1995=EDGE_CURVE('',#1572,#1574,#115,.T.);
#1996=EDGE_CURVE('',#1575,#1576,#946,.T.);
#1997=EDGE_CURVE('',#1573,#1575,#116,.F.);
#1998=EDGE_CURVE('',#1574,#1576,#117,.T.);
#1999=EDGE_CURVE('',#1577,#1578,#947,.T.);
#2000=EDGE_CURVE('',#1575,#1577,#118,.F.);
#2001=EDGE_CURVE('',#1576,#1578,#119,.T.);
#2002=EDGE_CURVE('',#1579,#1580,#948,.T.);
#2003=EDGE_CURVE('',#1577,#1579,#120,.F.);
#2004=EDGE_CURVE('',#1578,#1580,#121,.T.);
#2005=EDGE_CURVE('',#1581,#1582,#949,.T.);
#2006=EDGE_CURVE('',#1579,#1581,#122,.F.);
#2007=EDGE_CURVE('',#1580,#1582,#123,.T.);
#2008=EDGE_CURVE('',#1583,#1583,#1311,.T.);
#2009=EDGE_CURVE('',#1583,#1584,#950,.T.);
#2010=EDGE_CURVE('',#1584,#1585,#124,.T.);
#2011=EDGE_CURVE('',#1585,#1586,#951,.T.);
#2012=EDGE_CURVE('',#1587,#1586,#125,.F.);
#2013=EDGE_CURVE('',#1587,#1588,#952,.T.);
#2014=EDGE_CURVE('',#1588,#1584,#126,.T.);
#2015=EDGE_CURVE('',#1589,#1589,#1312,.T.);
#2016=EDGE_CURVE('',#1589,#1590,#1313,.T.);
#2017=EDGE_CURVE('',#1591,#1590,#1314,.T.);
#2018=EDGE_CURVE('',#1590,#1591,#1315,.T.);
#2019=EDGE_CURVE('',#1581,#1587,#127,.F.);
#2020=EDGE_CURVE('',#1582,#1588,#128,.T.);
#2021=EDGE_CURVE('',#1592,#1592,#1316,.T.);
#2022=EDGE_CURVE('',#1592,#1593,#953,.T.);
#2023=EDGE_CURVE('',#1593,#1593,#1317,.T.);
#2024=EDGE_CURVE('',#1591,#1594,#954,.T.);
#2025=EDGE_CURVE('',#1594,#1594,#1318,.T.);
#2026=EDGE_CURVE('',#1595,#1531,#955,.T.);
#2027=EDGE_CURVE('',#1596,#1595,#956,.T.);
#2028=EDGE_CURVE('',#1534,#1596,#957,.T.);
#2029=EDGE_CURVE('',#1586,#1475,#958,.T.);
#2030=EDGE_CURVE('',#1476,#1585,#959,.T.);
#2031=EDGE_CURVE('',#1595,#1527,#205,.T.);
#2032=EDGE_CURVE('',#1596,#1528,#206,.T.);
#2485=ORIENTED_EDGE('',*,*,#1846,.F.);
#2486=ORIENTED_EDGE('',*,*,#1847,.T.);
#2487=ORIENTED_EDGE('',*,*,#1848,.T.);
#2488=ORIENTED_EDGE('',*,*,#1849,.F.);
#2489=ORIENTED_EDGE('',*,*,#1850,.F.);
#2490=ORIENTED_EDGE('',*,*,#1851,.T.);
#2491=ORIENTED_EDGE('',*,*,#1846,.T.);
#2492=ORIENTED_EDGE('',*,*,#1852,.F.);
#2493=ORIENTED_EDGE('',*,*,#1853,.F.);
#2494=ORIENTED_EDGE('',*,*,#1854,.T.);
#2495=ORIENTED_EDGE('',*,*,#1850,.T.);
#2496=ORIENTED_EDGE('',*,*,#1855,.F.);
#2497=ORIENTED_EDGE('',*,*,#1856,.F.);
#2498=ORIENTED_EDGE('',*,*,#1857,.T.);
#2499=ORIENTED_EDGE('',*,*,#1853,.T.);
#2500=ORIENTED_EDGE('',*,*,#1858,.F.);
#2501=ORIENTED_EDGE('',*,*,#1859,.F.);
#2502=ORIENTED_EDGE('',*,*,#1860,.T.);
#2503=ORIENTED_EDGE('',*,*,#1856,.T.);
#2504=ORIENTED_EDGE('',*,*,#1861,.F.);
#2505=ORIENTED_EDGE('',*,*,#1862,.F.);
#2506=ORIENTED_EDGE('',*,*,#1863,.T.);
#2507=ORIENTED_EDGE('',*,*,#1859,.T.);
#2508=ORIENTED_EDGE('',*,*,#1864,.F.);
#2509=ORIENTED_EDGE('',*,*,#1865,.F.);
#2510=ORIENTED_EDGE('',*,*,#1866,.T.);
#2511=ORIENTED_EDGE('',*,*,#1862,.T.);
#2512=ORIENTED_EDGE('',*,*,#1867,.F.);
#2513=ORIENTED_EDGE('',*,*,#1868,.F.);
#2514=ORIENTED_EDGE('',*,*,#1869,.T.);
#2515=ORIENTED_EDGE('',*,*,#1865,.T.);
#2516=ORIENTED_EDGE('',*,*,#1870,.F.);
#2517=ORIENTED_EDGE('',*,*,#1871,.F.);
#2518=ORIENTED_EDGE('',*,*,#1872,.T.);
#2519=ORIENTED_EDGE('',*,*,#1868,.T.);
#2520=ORIENTED_EDGE('',*,*,#1873,.F.);
#2521=ORIENTED_EDGE('',*,*,#1874,.F.);
#2522=ORIENTED_EDGE('',*,*,#1875,.T.);
#2523=ORIENTED_EDGE('',*,*,#1871,.T.);
#2524=ORIENTED_EDGE('',*,*,#1876,.F.);
#2525=ORIENTED_EDGE('',*,*,#1877,.F.);
#2526=ORIENTED_EDGE('',*,*,#1878,.T.);
#2527=ORIENTED_EDGE('',*,*,#1874,.T.);
#2528=ORIENTED_EDGE('',*,*,#1879,.F.);
#2529=ORIENTED_EDGE('',*,*,#1880,.F.);
#2530=ORIENTED_EDGE('',*,*,#1881,.T.);
#2531=ORIENTED_EDGE('',*,*,#1877,.T.);
#2532=ORIENTED_EDGE('',*,*,#1882,.F.);
#2533=ORIENTED_EDGE('',*,*,#1883,.F.);
#2534=ORIENTED_EDGE('',*,*,#1884,.T.);
#2535=ORIENTED_EDGE('',*,*,#1880,.T.);
#2536=ORIENTED_EDGE('',*,*,#1885,.F.);
#2537=ORIENTED_EDGE('',*,*,#1886,.F.);
#2538=ORIENTED_EDGE('',*,*,#1887,.T.);
#2539=ORIENTED_EDGE('',*,*,#1883,.T.);
#2540=ORIENTED_EDGE('',*,*,#1888,.F.);
#2541=ORIENTED_EDGE('',*,*,#1889,.F.);
#2542=ORIENTED_EDGE('',*,*,#1890,.T.);
#2543=ORIENTED_EDGE('',*,*,#1886,.T.);
#2544=ORIENTED_EDGE('',*,*,#1891,.F.);
#2545=ORIENTED_EDGE('',*,*,#1892,.F.);
#2546=ORIENTED_EDGE('',*,*,#1893,.T.);
#2547=ORIENTED_EDGE('',*,*,#1889,.T.);
#2548=ORIENTED_EDGE('',*,*,#1894,.F.);
#2549=ORIENTED_EDGE('',*,*,#1895,.F.);
#2550=ORIENTED_EDGE('',*,*,#1896,.T.);
#2551=ORIENTED_EDGE('',*,*,#1892,.T.);
#2552=ORIENTED_EDGE('',*,*,#1897,.F.);
#2553=ORIENTED_EDGE('',*,*,#1898,.F.);
#2554=ORIENTED_EDGE('',*,*,#1899,.T.);
#2555=ORIENTED_EDGE('',*,*,#1895,.T.);
#2556=ORIENTED_EDGE('',*,*,#1900,.F.);
#2557=ORIENTED_EDGE('',*,*,#1901,.F.);
#2558=ORIENTED_EDGE('',*,*,#1902,.T.);
#2559=ORIENTED_EDGE('',*,*,#1898,.T.);
#2560=ORIENTED_EDGE('',*,*,#1903,.F.);
#2561=ORIENTED_EDGE('',*,*,#1904,.F.);
#2562=ORIENTED_EDGE('',*,*,#1905,.T.);
#2563=ORIENTED_EDGE('',*,*,#1901,.T.);
#2564=ORIENTED_EDGE('',*,*,#1906,.F.);
#2565=ORIENTED_EDGE('',*,*,#1907,.F.);
#2566=ORIENTED_EDGE('',*,*,#1908,.T.);
#2567=ORIENTED_EDGE('',*,*,#1904,.T.);
#2568=ORIENTED_EDGE('',*,*,#1909,.F.);
#2569=ORIENTED_EDGE('',*,*,#1910,.F.);
#2570=ORIENTED_EDGE('',*,*,#1911,.T.);
#2571=ORIENTED_EDGE('',*,*,#1907,.T.);
#2572=ORIENTED_EDGE('',*,*,#1912,.F.);
#2573=ORIENTED_EDGE('',*,*,#1913,.F.);
#2574=ORIENTED_EDGE('',*,*,#1914,.T.);
#2575=ORIENTED_EDGE('',*,*,#1910,.T.);
#2576=ORIENTED_EDGE('',*,*,#1915,.F.);
#2577=ORIENTED_EDGE('',*,*,#1916,.F.);
#2578=ORIENTED_EDGE('',*,*,#1917,.T.);
#2579=ORIENTED_EDGE('',*,*,#1913,.T.);
#2580=ORIENTED_EDGE('',*,*,#1918,.F.);
#2581=ORIENTED_EDGE('',*,*,#1919,.F.);
#2582=ORIENTED_EDGE('',*,*,#1920,.T.);
#2583=ORIENTED_EDGE('',*,*,#1916,.T.);
#2584=ORIENTED_EDGE('',*,*,#1921,.F.);
#2585=ORIENTED_EDGE('',*,*,#1922,.F.);
#2586=ORIENTED_EDGE('',*,*,#1923,.T.);
#2587=ORIENTED_EDGE('',*,*,#1919,.T.);
#2588=ORIENTED_EDGE('',*,*,#1924,.F.);
#2589=ORIENTED_EDGE('',*,*,#1925,.F.);
#2590=ORIENTED_EDGE('',*,*,#1926,.T.);
#2591=ORIENTED_EDGE('',*,*,#1922,.T.);
#2592=ORIENTED_EDGE('',*,*,#1927,.F.);
#2593=ORIENTED_EDGE('',*,*,#1928,.F.);
#2594=ORIENTED_EDGE('',*,*,#1929,.F.);
#2595=ORIENTED_EDGE('',*,*,#1930,.F.);
#2596=ORIENTED_EDGE('',*,*,#1931,.F.);
#2597=ORIENTED_EDGE('',*,*,#1932,.F.);
#2598=ORIENTED_EDGE('',*,*,#1928,.T.);
#2599=ORIENTED_EDGE('',*,*,#1933,.F.);
#2600=ORIENTED_EDGE('',*,*,#1934,.T.);
#2601=ORIENTED_EDGE('',*,*,#1935,.T.);
#2602=ORIENTED_EDGE('',*,*,#1936,.F.);
#2603=ORIENTED_EDGE('',*,*,#1937,.F.);
#2604=ORIENTED_EDGE('',*,*,#1931,.T.);
#2605=ORIENTED_EDGE('',*,*,#1938,.T.);
#2606=ORIENTED_EDGE('',*,*,#1939,.F.);
#2607=ORIENTED_EDGE('',*,*,#1940,.F.);
#2608=ORIENTED_EDGE('',*,*,#1936,.T.);
#2609=ORIENTED_EDGE('',*,*,#1941,.T.);
#2610=ORIENTED_EDGE('',*,*,#1942,.F.);
#2611=ORIENTED_EDGE('',*,*,#1943,.F.);
#2612=ORIENTED_EDGE('',*,*,#1939,.T.);
#2613=ORIENTED_EDGE('',*,*,#1944,.T.);
#2614=ORIENTED_EDGE('',*,*,#1945,.F.);
#2615=ORIENTED_EDGE('',*,*,#1946,.F.);
#2616=ORIENTED_EDGE('',*,*,#1942,.T.);
#2617=ORIENTED_EDGE('',*,*,#1947,.T.);
#2618=ORIENTED_EDGE('',*,*,#1948,.F.);
#2619=ORIENTED_EDGE('',*,*,#1949,.F.);
#2620=ORIENTED_EDGE('',*,*,#1945,.T.);
#2621=ORIENTED_EDGE('',*,*,#1950,.T.);
#2622=ORIENTED_EDGE('',*,*,#1951,.F.);
#2623=ORIENTED_EDGE('',*,*,#1952,.F.);
#2624=ORIENTED_EDGE('',*,*,#1948,.T.);
#2625=ORIENTED_EDGE('',*,*,#1953,.T.);
#2626=ORIENTED_EDGE('',*,*,#1954,.F.);
#2627=ORIENTED_EDGE('',*,*,#1955,.F.);
#2628=ORIENTED_EDGE('',*,*,#1951,.T.);
#2629=ORIENTED_EDGE('',*,*,#1956,.T.);
#2630=ORIENTED_EDGE('',*,*,#1957,.F.);
#2631=ORIENTED_EDGE('',*,*,#1958,.F.);
#2632=ORIENTED_EDGE('',*,*,#1954,.T.);
#2633=ORIENTED_EDGE('',*,*,#1959,.T.);
#2634=ORIENTED_EDGE('',*,*,#1960,.F.);
#2635=ORIENTED_EDGE('',*,*,#1961,.F.);
#2636=ORIENTED_EDGE('',*,*,#1957,.T.);
#2637=ORIENTED_EDGE('',*,*,#1962,.T.);
#2638=ORIENTED_EDGE('',*,*,#1963,.F.);
#2639=ORIENTED_EDGE('',*,*,#1964,.F.);
#2640=ORIENTED_EDGE('',*,*,#1960,.T.);
#2641=ORIENTED_EDGE('',*,*,#1965,.T.);
#2642=ORIENTED_EDGE('',*,*,#1966,.F.);
#2643=ORIENTED_EDGE('',*,*,#1967,.F.);
#2644=ORIENTED_EDGE('',*,*,#1963,.T.);
#2645=ORIENTED_EDGE('',*,*,#1968,.T.);
#2646=ORIENTED_EDGE('',*,*,#1969,.F.);
#2647=ORIENTED_EDGE('',*,*,#1970,.F.);
#2648=ORIENTED_EDGE('',*,*,#1966,.T.);
#2649=ORIENTED_EDGE('',*,*,#1971,.T.);
#2650=ORIENTED_EDGE('',*,*,#1972,.F.);
#2651=ORIENTED_EDGE('',*,*,#1973,.F.);
#2652=ORIENTED_EDGE('',*,*,#1969,.T.);
#2653=ORIENTED_EDGE('',*,*,#1974,.T.);
#2654=ORIENTED_EDGE('',*,*,#1975,.F.);
#2655=ORIENTED_EDGE('',*,*,#1976,.F.);
#2656=ORIENTED_EDGE('',*,*,#1972,.T.);
#2657=ORIENTED_EDGE('',*,*,#1977,.T.);
#2658=ORIENTED_EDGE('',*,*,#1978,.F.);
#2659=ORIENTED_EDGE('',*,*,#1979,.F.);
#2660=ORIENTED_EDGE('',*,*,#1975,.T.);
#2661=ORIENTED_EDGE('',*,*,#1980,.T.);
#2662=ORIENTED_EDGE('',*,*,#1981,.F.);
#2663=ORIENTED_EDGE('',*,*,#1982,.F.);
#2664=ORIENTED_EDGE('',*,*,#1978,.T.);
#2665=ORIENTED_EDGE('',*,*,#1983,.T.);
#2666=ORIENTED_EDGE('',*,*,#1984,.F.);
#2667=ORIENTED_EDGE('',*,*,#1985,.F.);
#2668=ORIENTED_EDGE('',*,*,#1981,.T.);
#2669=ORIENTED_EDGE('',*,*,#1986,.T.);
#2670=ORIENTED_EDGE('',*,*,#1987,.F.);
#2671=ORIENTED_EDGE('',*,*,#1988,.F.);
#2672=ORIENTED_EDGE('',*,*,#1984,.T.);
#2673=ORIENTED_EDGE('',*,*,#1989,.T.);
#2674=ORIENTED_EDGE('',*,*,#1990,.F.);
#2675=ORIENTED_EDGE('',*,*,#1991,.F.);
#2676=ORIENTED_EDGE('',*,*,#1987,.T.);
#2677=ORIENTED_EDGE('',*,*,#1992,.T.);
#2678=ORIENTED_EDGE('',*,*,#1993,.F.);
#2679=ORIENTED_EDGE('',*,*,#1994,.F.);
#2680=ORIENTED_EDGE('',*,*,#1990,.T.);
#2681=ORIENTED_EDGE('',*,*,#1995,.T.);
#2682=ORIENTED_EDGE('',*,*,#1996,.F.);
#2683=ORIENTED_EDGE('',*,*,#1997,.F.);
#2684=ORIENTED_EDGE('',*,*,#1993,.T.);
#2685=ORIENTED_EDGE('',*,*,#1998,.T.);
#2686=ORIENTED_EDGE('',*,*,#1999,.F.);
#2687=ORIENTED_EDGE('',*,*,#2000,.F.);
#2688=ORIENTED_EDGE('',*,*,#1996,.T.);
#2689=ORIENTED_EDGE('',*,*,#2001,.T.);
#2690=ORIENTED_EDGE('',*,*,#2002,.F.);
#2691=ORIENTED_EDGE('',*,*,#2003,.F.);
#2692=ORIENTED_EDGE('',*,*,#1999,.T.);
#2693=ORIENTED_EDGE('',*,*,#2004,.T.);
#2694=ORIENTED_EDGE('',*,*,#2005,.F.);
#2695=ORIENTED_EDGE('',*,*,#2006,.F.);
#2696=ORIENTED_EDGE('',*,*,#2002,.T.);
#2697=ORIENTED_EDGE('',*,*,#2007,.T.);
#2698=ORIENTED_EDGE('',*,*,#2008,.T.);
#2699=ORIENTED_EDGE('',*,*,#2009,.T.);
#2700=ORIENTED_EDGE('',*,*,#2010,.T.);
#2701=ORIENTED_EDGE('',*,*,#2011,.T.);
#2702=ORIENTED_EDGE('',*,*,#2012,.F.);
#2703=ORIENTED_EDGE('',*,*,#2013,.T.);
#2704=ORIENTED_EDGE('',*,*,#2014,.T.);
#2705=ORIENTED_EDGE('',*,*,#2009,.F.);
#2706=ORIENTED_EDGE('',*,*,#2015,.T.);
#2707=ORIENTED_EDGE('',*,*,#2016,.T.);
#2708=ORIENTED_EDGE('',*,*,#2017,.F.);
#2709=ORIENTED_EDGE('',*,*,#2018,.F.);
#2710=ORIENTED_EDGE('',*,*,#2016,.F.);
#2711=ORIENTED_EDGE('',*,*,#2013,.F.);
#2712=ORIENTED_EDGE('',*,*,#2019,.F.);
#2713=ORIENTED_EDGE('',*,*,#2005,.T.);
#2714=ORIENTED_EDGE('',*,*,#2020,.T.);
#2715=ORIENTED_EDGE('',*,*,#2021,.T.);
#2716=ORIENTED_EDGE('',*,*,#2022,.T.);
#2717=ORIENTED_EDGE('',*,*,#2023,.F.);
#2718=ORIENTED_EDGE('',*,*,#2022,.F.);
#2719=ORIENTED_EDGE('',*,*,#2017,.T.);
#2720=ORIENTED_EDGE('',*,*,#2018,.T.);
#2721=ORIENTED_EDGE('',*,*,#2024,.T.);
#2722=ORIENTED_EDGE('',*,*,#2025,.F.);
#2723=ORIENTED_EDGE('',*,*,#2024,.F.);
#2724=ORIENTED_EDGE('',*,*,#2015,.F.);
#2725=ORIENTED_EDGE('',*,*,#2023,.T.);
#2726=ORIENTED_EDGE('',*,*,#2008,.F.);
#2727=ORIENTED_EDGE('',*,*,#2021,.F.);
#2728=ORIENTED_EDGE('',*,*,#2025,.T.);
#2729=ORIENTED_EDGE('',*,*,#1933,.T.);
#2730=ORIENTED_EDGE('',*,*,#1930,.T.);
#2731=ORIENTED_EDGE('',*,*,#2026,.F.);
#2732=ORIENTED_EDGE('',*,*,#2027,.F.);
#2733=ORIENTED_EDGE('',*,*,#2028,.F.);
#2734=ORIENTED_EDGE('',*,*,#1934,.F.);
#2735=ORIENTED_EDGE('',*,*,#2029,.F.);
#2736=ORIENTED_EDGE('',*,*,#2011,.F.);
#2737=ORIENTED_EDGE('',*,*,#2030,.F.);
#2738=ORIENTED_EDGE('',*,*,#1848,.F.);
#2739=ORIENTED_EDGE('',*,*,#2026,.T.);
#2740=ORIENTED_EDGE('',*,*,#1929,.T.);
#2741=ORIENTED_EDGE('',*,*,#1932,.T.);
#2742=ORIENTED_EDGE('',*,*,#1937,.T.);
#2743=ORIENTED_EDGE('',*,*,#1940,.T.);
#2744=ORIENTED_EDGE('',*,*,#1943,.T.);
#2745=ORIENTED_EDGE('',*,*,#1946,.T.);
#2746=ORIENTED_EDGE('',*,*,#1949,.T.);
#2747=ORIENTED_EDGE('',*,*,#1952,.T.);
#2748=ORIENTED_EDGE('',*,*,#1955,.T.);
#2749=ORIENTED_EDGE('',*,*,#1958,.T.);
#2750=ORIENTED_EDGE('',*,*,#1961,.T.);
#2751=ORIENTED_EDGE('',*,*,#1964,.T.);
#2752=ORIENTED_EDGE('',*,*,#1967,.T.);
#2753=ORIENTED_EDGE('',*,*,#1970,.T.);
#2754=ORIENTED_EDGE('',*,*,#1973,.T.);
#2755=ORIENTED_EDGE('',*,*,#1976,.T.);
#2756=ORIENTED_EDGE('',*,*,#1979,.T.);
#2757=ORIENTED_EDGE('',*,*,#1982,.T.);
#2758=ORIENTED_EDGE('',*,*,#1985,.T.);
#2759=ORIENTED_EDGE('',*,*,#1988,.T.);
#2760=ORIENTED_EDGE('',*,*,#1991,.T.);
#2761=ORIENTED_EDGE('',*,*,#1994,.T.);
#2762=ORIENTED_EDGE('',*,*,#1997,.T.);
#2763=ORIENTED_EDGE('',*,*,#2000,.T.);
#2764=ORIENTED_EDGE('',*,*,#2003,.T.);
#2765=ORIENTED_EDGE('',*,*,#2006,.T.);
#2766=ORIENTED_EDGE('',*,*,#2019,.T.);
#2767=ORIENTED_EDGE('',*,*,#2012,.T.);
#2768=ORIENTED_EDGE('',*,*,#2029,.T.);
#2769=ORIENTED_EDGE('',*,*,#1847,.F.);
#2770=ORIENTED_EDGE('',*,*,#1851,.F.);
#2771=ORIENTED_EDGE('',*,*,#1854,.F.);
#2772=ORIENTED_EDGE('',*,*,#1857,.F.);
#2773=ORIENTED_EDGE('',*,*,#1860,.F.);
#2774=ORIENTED_EDGE('',*,*,#1863,.F.);
#2775=ORIENTED_EDGE('',*,*,#1866,.F.);
#2776=ORIENTED_EDGE('',*,*,#1869,.F.);
#2777=ORIENTED_EDGE('',*,*,#1872,.F.);
#2778=ORIENTED_EDGE('',*,*,#1875,.F.);
#2779=ORIENTED_EDGE('',*,*,#1878,.F.);
#2780=ORIENTED_EDGE('',*,*,#1881,.F.);
#2781=ORIENTED_EDGE('',*,*,#1884,.F.);
#2782=ORIENTED_EDGE('',*,*,#1887,.F.);
#2783=ORIENTED_EDGE('',*,*,#1890,.F.);
#2784=ORIENTED_EDGE('',*,*,#1893,.F.);
#2785=ORIENTED_EDGE('',*,*,#1896,.F.);
#2786=ORIENTED_EDGE('',*,*,#1899,.F.);
#2787=ORIENTED_EDGE('',*,*,#1902,.F.);
#2788=ORIENTED_EDGE('',*,*,#1905,.F.);
#2789=ORIENTED_EDGE('',*,*,#1908,.F.);
#2790=ORIENTED_EDGE('',*,*,#1911,.F.);
#2791=ORIENTED_EDGE('',*,*,#1914,.F.);
#2792=ORIENTED_EDGE('',*,*,#1917,.F.);
#2793=ORIENTED_EDGE('',*,*,#1920,.F.);
#2794=ORIENTED_EDGE('',*,*,#1923,.F.);
#2795=ORIENTED_EDGE('',*,*,#1926,.F.);
#2796=ORIENTED_EDGE('',*,*,#2031,.F.);
#2797=ORIENTED_EDGE('',*,*,#1925,.T.);
#2798=ORIENTED_EDGE('',*,*,#2032,.F.);
#2799=ORIENTED_EDGE('',*,*,#2027,.T.);
#2800=ORIENTED_EDGE('',*,*,#2031,.T.);
#2801=ORIENTED_EDGE('',*,*,#2028,.T.);
#2802=ORIENTED_EDGE('',*,*,#2032,.T.);
#2803=ORIENTED_EDGE('',*,*,#1927,.T.);
#2804=ORIENTED_EDGE('',*,*,#1924,.T.);
#2805=ORIENTED_EDGE('',*,*,#1921,.T.);
#2806=ORIENTED_EDGE('',*,*,#1918,.T.);
#2807=ORIENTED_EDGE('',*,*,#1915,.T.);
#2808=ORIENTED_EDGE('',*,*,#1912,.T.);
#2809=ORIENTED_EDGE('',*,*,#1909,.T.);
#2810=ORIENTED_EDGE('',*,*,#1906,.T.);
#2811=ORIENTED_EDGE('',*,*,#1903,.T.);
#2812=ORIENTED_EDGE('',*,*,#1900,.T.);
#2813=ORIENTED_EDGE('',*,*,#1897,.T.);
#2814=ORIENTED_EDGE('',*,*,#1894,.T.);
#2815=ORIENTED_EDGE('',*,*,#1891,.T.);
#2816=ORIENTED_EDGE('',*,*,#1888,.T.);
#2817=ORIENTED_EDGE('',*,*,#1885,.T.);
#2818=ORIENTED_EDGE('',*,*,#1882,.T.);
#2819=ORIENTED_EDGE('',*,*,#1879,.T.);
#2820=ORIENTED_EDGE('',*,*,#1876,.T.);
#2821=ORIENTED_EDGE('',*,*,#1873,.T.);
#2822=ORIENTED_EDGE('',*,*,#1870,.T.);
#2823=ORIENTED_EDGE('',*,*,#1867,.T.);
#2824=ORIENTED_EDGE('',*,*,#1864,.T.);
#2825=ORIENTED_EDGE('',*,*,#1861,.T.);
#2826=ORIENTED_EDGE('',*,*,#1858,.T.);
#2827=ORIENTED_EDGE('',*,*,#1855,.T.);
#2828=ORIENTED_EDGE('',*,*,#1852,.T.);
#2829=ORIENTED_EDGE('',*,*,#1849,.T.);
#2830=ORIENTED_EDGE('',*,*,#2030,.T.);
#2831=ORIENTED_EDGE('',*,*,#2010,.F.);
#2832=ORIENTED_EDGE('',*,*,#2014,.F.);
#2833=ORIENTED_EDGE('',*,*,#2020,.F.);
#2834=ORIENTED_EDGE('',*,*,#2007,.F.);
#2835=ORIENTED_EDGE('',*,*,#2004,.F.);
#2836=ORIENTED_EDGE('',*,*,#2001,.F.);
#2837=ORIENTED_EDGE('',*,*,#1998,.F.);
#2838=ORIENTED_EDGE('',*,*,#1995,.F.);
#2839=ORIENTED_EDGE('',*,*,#1992,.F.);
#2840=ORIENTED_EDGE('',*,*,#1989,.F.);
#2841=ORIENTED_EDGE('',*,*,#1986,.F.);
#2842=ORIENTED_EDGE('',*,*,#1983,.F.);
#2843=ORIENTED_EDGE('',*,*,#1980,.F.);
#2844=ORIENTED_EDGE('',*,*,#1977,.F.);
#2845=ORIENTED_EDGE('',*,*,#1974,.F.);
#2846=ORIENTED_EDGE('',*,*,#1971,.F.);
#2847=ORIENTED_EDGE('',*,*,#1968,.F.);
#2848=ORIENTED_EDGE('',*,*,#1965,.F.);
#2849=ORIENTED_EDGE('',*,*,#1962,.F.);
#2850=ORIENTED_EDGE('',*,*,#1959,.F.);
#2851=ORIENTED_EDGE('',*,*,#1956,.F.);
#2852=ORIENTED_EDGE('',*,*,#1953,.F.);
#2853=ORIENTED_EDGE('',*,*,#1950,.F.);
#2854=ORIENTED_EDGE('',*,*,#1947,.F.);
#2855=ORIENTED_EDGE('',*,*,#1944,.F.);
#2856=ORIENTED_EDGE('',*,*,#1941,.F.);
#2857=ORIENTED_EDGE('',*,*,#1938,.F.);
#2858=ORIENTED_EDGE('',*,*,#1935,.F.);
#3198=CYLINDRICAL_SURFACE('',#3650,5.75643035625);
#3199=CYLINDRICAL_SURFACE('',#3651,5.75643035625);
#3200=CYLINDRICAL_SURFACE('',#3652,5.75643035625);
#3201=CYLINDRICAL_SURFACE('',#3653,5.75643035625);
#3202=CYLINDRICAL_SURFACE('',#3654,5.75643035625);
#3203=CYLINDRICAL_SURFACE('',#3655,5.75643035625);
#3204=CYLINDRICAL_SURFACE('',#3656,5.75643035625);
#3205=CYLINDRICAL_SURFACE('',#3657,5.75643035625);
#3206=CYLINDRICAL_SURFACE('',#3658,5.75643035625);
#3207=CYLINDRICAL_SURFACE('',#3659,5.75643035625);
#3208=CYLINDRICAL_SURFACE('',#3660,5.75643035625);
#3209=CYLINDRICAL_SURFACE('',#3661,5.75643035625);
#3210=CYLINDRICAL_SURFACE('',#3662,5.75643035625);
#3211=CYLINDRICAL_SURFACE('',#3663,5.75643035625);
#3212=CYLINDRICAL_SURFACE('',#3664,5.75643035625);
#3213=CYLINDRICAL_SURFACE('',#3665,5.75643035625);
#3214=CYLINDRICAL_SURFACE('',#3666,5.75643035625);
#3215=CYLINDRICAL_SURFACE('',#3667,5.75643035625);
#3216=CYLINDRICAL_SURFACE('',#3668,5.75643035625);
#3217=CYLINDRICAL_SURFACE('',#3669,5.75643035625);
#3218=CYLINDRICAL_SURFACE('',#3670,5.75643035625);
#3219=CYLINDRICAL_SURFACE('',#3671,5.75643035625);
#3220=CYLINDRICAL_SURFACE('',#3672,5.75643035625);
#3221=CYLINDRICAL_SURFACE('',#3673,5.75643035625);
#3222=CYLINDRICAL_SURFACE('',#3674,5.75643035625);
#3223=CYLINDRICAL_SURFACE('',#3675,5.75643035625);
#3224=CYLINDRICAL_SURFACE('',#3676,5.75643035625);
#3225=CYLINDRICAL_SURFACE('',#3677,6.);
#3226=CYLINDRICAL_SURFACE('',#3679,6.);
#3227=CYLINDRICAL_SURFACE('',#3681,6.);
#3228=CYLINDRICAL_SURFACE('',#3682,6.);
#3229=CYLINDRICAL_SURFACE('',#3683,6.);
#3230=CYLINDRICAL_SURFACE('',#3684,6.);
#3231=CYLINDRICAL_SURFACE('',#3685,6.);
#3232=CYLINDRICAL_SURFACE('',#3686,6.);
#3233=CYLINDRICAL_SURFACE('',#3687,6.);
#3234=CYLINDRICAL_SURFACE('',#3688,6.);
#3235=CYLINDRICAL_SURFACE('',#3689,6.);
#3236=CYLINDRICAL_SURFACE('',#3690,6.);
#3237=CYLINDRICAL_SURFACE('',#3691,6.);
#3238=CYLINDRICAL_SURFACE('',#3692,6.);
#3239=CYLINDRICAL_SURFACE('',#3693,6.);
#3240=CYLINDRICAL_SURFACE('',#3694,6.);
#3241=CYLINDRICAL_SURFACE('',#3695,6.);
#3242=CYLINDRICAL_SURFACE('',#3696,6.);
#3243=CYLINDRICAL_SURFACE('',#3697,6.);
#3244=CYLINDRICAL_SURFACE('',#3698,6.);
#3245=CYLINDRICAL_SURFACE('',#3699,6.);
#3246=CYLINDRICAL_SURFACE('',#3700,6.);
#3247=CYLINDRICAL_SURFACE('',#3701,6.);
#3248=CYLINDRICAL_SURFACE('',#3702,6.);
#3249=CYLINDRICAL_SURFACE('',#3703,6.);
#3250=CYLINDRICAL_SURFACE('',#3704,6.);
#3251=CYLINDRICAL_SURFACE('',#3705,6.);
#3252=CYLINDRICAL_SURFACE('',#3712,6.);
#3253=CYLINDRICAL_SURFACE('',#3713,9.);
#3254=CYLINDRICAL_SURFACE('',#3716,6.);
#3255=CYLINDRICAL_SURFACE('',#3724,5.75643035625);
#3325=ADVANCED_FACE('',(#415),#3198,.T.);
#3326=ADVANCED_FACE('',(#416),#3199,.T.);
#3327=ADVANCED_FACE('',(#417),#3200,.T.);
#3328=ADVANCED_FACE('',(#418),#3201,.T.);
#3329=ADVANCED_FACE('',(#419),#3202,.T.);
#3330=ADVANCED_FACE('',(#420),#3203,.T.);
#3331=ADVANCED_FACE('',(#421),#3204,.T.);
#3332=ADVANCED_FACE('',(#422),#3205,.T.);
#3333=ADVANCED_FACE('',(#423),#3206,.T.);
#3334=ADVANCED_FACE('',(#424),#3207,.T.);
#3335=ADVANCED_FACE('',(#425),#3208,.T.);
#3336=ADVANCED_FACE('',(#426),#3209,.T.);
#3337=ADVANCED_FACE('',(#427),#3210,.T.);
#3338=ADVANCED_FACE('',(#428),#3211,.T.);
#3339=ADVANCED_FACE('',(#429),#3212,.T.);
#3340=ADVANCED_FACE('',(#430),#3213,.T.);
#3341=ADVANCED_FACE('',(#431),#3214,.T.);
#3342=ADVANCED_FACE('',(#432),#3215,.T.);
#3343=ADVANCED_FACE('',(#433),#3216,.T.);
#3344=ADVANCED_FACE('',(#434),#3217,.T.);
#3345=ADVANCED_FACE('',(#435),#3218,.T.);
#3346=ADVANCED_FACE('',(#436),#3219,.T.);
#3347=ADVANCED_FACE('',(#437),#3220,.T.);
#3348=ADVANCED_FACE('',(#438),#3221,.T.);
#3349=ADVANCED_FACE('',(#439),#3222,.T.);
#3350=ADVANCED_FACE('',(#440),#3223,.T.);
#3351=ADVANCED_FACE('',(#441),#3224,.T.);
#3352=ADVANCED_FACE('',(#442),#3225,.T.);
#3353=ADVANCED_FACE('',(#443),#3226,.T.);
#3354=ADVANCED_FACE('',(#444),#3227,.T.);
#3355=ADVANCED_FACE('',(#445),#3228,.T.);
#3356=ADVANCED_FACE('',(#446),#3229,.T.);
#3357=ADVANCED_FACE('',(#447),#3230,.T.);
#3358=ADVANCED_FACE('',(#448),#3231,.T.);
#3359=ADVANCED_FACE('',(#449),#3232,.T.);
#3360=ADVANCED_FACE('',(#450),#3233,.T.);
#3361=ADVANCED_FACE('',(#451),#3234,.T.);
#3362=ADVANCED_FACE('',(#452),#3235,.T.);
#3363=ADVANCED_FACE('',(#453),#3236,.T.);
#3364=ADVANCED_FACE('',(#454),#3237,.T.);
#3365=ADVANCED_FACE('',(#455),#3238,.T.);
#3366=ADVANCED_FACE('',(#456),#3239,.T.);
#3367=ADVANCED_FACE('',(#457),#3240,.T.);
#3368=ADVANCED_FACE('',(#458),#3241,.T.);
#3369=ADVANCED_FACE('',(#459),#3242,.T.);
#3370=ADVANCED_FACE('',(#460),#3243,.T.);
#3371=ADVANCED_FACE('',(#461),#3244,.T.);
#3372=ADVANCED_FACE('',(#462),#3245,.T.);
#3373=ADVANCED_FACE('',(#463),#3246,.T.);
#3374=ADVANCED_FACE('',(#464),#3247,.T.);
#3375=ADVANCED_FACE('',(#465),#3248,.T.);
#3376=ADVANCED_FACE('',(#466),#3249,.T.);
#3377=ADVANCED_FACE('',(#467),#3250,.T.);
#3378=ADVANCED_FACE('',(#468),#3251,.T.);
#3379=ADVANCED_FACE('',(#469),#71,.T.);
#3380=ADVANCED_FACE('',(#470),#3252,.T.);
#3381=ADVANCED_FACE('',(#471),#3253,.T.);
#3382=ADVANCED_FACE('',(#472),#3254,.T.);
#3383=ADVANCED_FACE('',(#473),#324,.F.);
#3384=ADVANCED_FACE('',(#474,#265),#325,.T.);
#3385=ADVANCED_FACE('',(#475,#266),#326,.F.);
#3386=ADVANCED_FACE('',(#476),#327,.T.);
#3387=ADVANCED_FACE('',(#477),#328,.F.);
#3388=ADVANCED_FACE('',(#478),#329,.T.);
#3389=ADVANCED_FACE('',(#479),#61,.T.);
#3390=ADVANCED_FACE('',(#480),#3255,.T.);
#3391=ADVANCED_FACE('',(#481),#62,.T.);
#3467=CLOSED_SHELL('',(#3325,#3326,#3327,#3328,#3329,#3330,#3331,#3332,
#3333,#3334,#3335,#3336,#3337,#3338,#3339,#3340,#3341,#3342,#3343,#3344,
#3345,#3346,#3347,#3348,#3349,#3350,#3351,#3352,#3353,#3354,#3355,#3356,
#3357,#3358,#3359,#3360,#3361,#3362,#3363,#3364,#3365,#3366,#3367,#3368,
#3369,#3370,#3371,#3372,#3373,#3374,#3375,#3376,#3377,#3378,#3379,#3380,
#3381,#3382,#3383,#3384,#3385,#3386,#3387,#3388,#3389,#3390,#3391));
#3649=AXIS2_PLACEMENT_3D('',#4994,#4136,#4137);
#3650=AXIS2_PLACEMENT_3D('',#4995,#4138,#4139);
#3651=AXIS2_PLACEMENT_3D('',#5008,#4142,#4143);
#3652=AXIS2_PLACEMENT_3D('',#5038,#4145,#4146);
#3653=AXIS2_PLACEMENT_3D('',#5068,#4148,#4149);
#3654=AXIS2_PLACEMENT_3D('',#5098,#4151,#4152);
#3655=AXIS2_PLACEMENT_3D('',#5128,#4154,#4155);
#3656=AXIS2_PLACEMENT_3D('',#5158,#4157,#4158);
#3657=AXIS2_PLACEMENT_3D('',#5188,#4160,#4161);
#3658=AXIS2_PLACEMENT_3D('',#5218,#4163,#4164);
#3659=AXIS2_PLACEMENT_3D('',#5248,#4166,#4167);
#3660=AXIS2_PLACEMENT_3D('',#5278,#4169,#4170);
#3661=AXIS2_PLACEMENT_3D('',#5308,#4172,#4173);
#3662=AXIS2_PLACEMENT_3D('',#5338,#4175,#4176);
#3663=AXIS2_PLACEMENT_3D('',#5368,#4178,#4179);
#3664=AXIS2_PLACEMENT_3D('',#5398,#4181,#4182);
#3665=AXIS2_PLACEMENT_3D('',#5428,#4184,#4185);
#3666=AXIS2_PLACEMENT_3D('',#5458,#4187,#4188);
#3667=AXIS2_PLACEMENT_3D('',#5488,#4190,#4191);
#3668=AXIS2_PLACEMENT_3D('',#5518,#4193,#4194);
#3669=AXIS2_PLACEMENT_3D('',#5548,#4196,#4197);
#3670=AXIS2_PLACEMENT_3D('',#5578,#4199,#4200);
#3671=AXIS2_PLACEMENT_3D('',#5608,#4202,#4203);
#3672=AXIS2_PLACEMENT_3D('',#5638,#4205,#4206);
#3673=AXIS2_PLACEMENT_3D('',#5668,#4208,#4209);
#3674=AXIS2_PLACEMENT_3D('',#5698,#4211,#4212);
#3675=AXIS2_PLACEMENT_3D('',#5728,#4214,#4215);
#3676=AXIS2_PLACEMENT_3D('',#5758,#4217,#4218);
#3677=AXIS2_PLACEMENT_3D('',#5788,#4220,#4221);
#3678=AXIS2_PLACEMENT_3D('',#5805,#4223,#4224);
#3679=AXIS2_PLACEMENT_3D('',#5806,#4225,#4226);
#3680=AXIS2_PLACEMENT_3D('',#5846,#4228,#4229);
#3681=AXIS2_PLACEMENT_3D('',#5861,#4231,#4232);
#3682=AXIS2_PLACEMENT_3D('',#5937,#4234,#4235);
#3683=AXIS2_PLACEMENT_3D('',#6015,#4237,#4238);
#3684=AXIS2_PLACEMENT_3D('',#6093,#4240,#4241);
#3685=AXIS2_PLACEMENT_3D('',#6169,#4243,#4244);
#3686=AXIS2_PLACEMENT_3D('',#6245,#4246,#4247);
#3687=AXIS2_PLACEMENT_3D('',#6321,#4249,#4250);
#3688=AXIS2_PLACEMENT_3D('',#6399,#4252,#4253);
#3689=AXIS2_PLACEMENT_3D('',#6475,#4255,#4256);
#3690=AXIS2_PLACEMENT_3D('',#6553,#4258,#4259);
#3691=AXIS2_PLACEMENT_3D('',#6629,#4261,#4262);
#3692=AXIS2_PLACEMENT_3D('',#6705,#4264,#4265);
#3693=AXIS2_PLACEMENT_3D('',#6781,#4267,#4268);
#3694=AXIS2_PLACEMENT_3D('',#6857,#4270,#4271);
#3695=AXIS2_PLACEMENT_3D('',#6935,#4273,#4274);
#3696=AXIS2_PLACEMENT_3D('',#7013,#4276,#4277);
#3697=AXIS2_PLACEMENT_3D('',#7089,#4279,#4280);
#3698=AXIS2_PLACEMENT_3D('',#7165,#4282,#4283);
#3699=AXIS2_PLACEMENT_3D('',#7241,#4285,#4286);
#3700=AXIS2_PLACEMENT_3D('',#7319,#4288,#4289);
#3701=AXIS2_PLACEMENT_3D('',#7397,#4291,#4292);
#3702=AXIS2_PLACEMENT_3D('',#7473,#4294,#4295);
#3703=AXIS2_PLACEMENT_3D('',#7549,#4297,#4298);
#3704=AXIS2_PLACEMENT_3D('',#7625,#4300,#4301);
#3705=AXIS2_PLACEMENT_3D('',#7701,#4303,#4304);
#3706=AXIS2_PLACEMENT_3D('',#7703,#4305,#4306);
#3707=AXIS2_PLACEMENT_3D('',#7782,#4310,#4311);
#3708=AXIS2_PLACEMENT_3D('',#7784,#4312,#4313);
#3709=AXIS2_PLACEMENT_3D('',#7786,#4314,#4315);
#3710=AXIS2_PLACEMENT_3D('',#7788,#4316,#4317);
#3711=AXIS2_PLACEMENT_3D('',#7789,#4318,#4319);
#3712=AXIS2_PLACEMENT_3D('',#7790,#4320,#4321);
#3713=AXIS2_PLACEMENT_3D('',#7865,#4322,#4323);
#3714=AXIS2_PLACEMENT_3D('',#7867,#4324,#4325);
#3715=AXIS2_PLACEMENT_3D('',#7870,#4327,#4328);
#3716=AXIS2_PLACEMENT_3D('',#7871,#4329,#4330);
#3717=AXIS2_PLACEMENT_3D('',#7874,#4332,#4333);
#3718=AXIS2_PLACEMENT_3D('',#7875,#4334,#4335);
#3719=AXIS2_PLACEMENT_3D('',#7876,#4336,#4337);
#3720=AXIS2_PLACEMENT_3D('',#7877,#4338,#4339);
#3721=AXIS2_PLACEMENT_3D('',#7878,#4340,#4341);
#3722=AXIS2_PLACEMENT_3D('',#7879,#4342,#4343);
#3723=AXIS2_PLACEMENT_3D('',#7885,#4347,#4348);
#3724=AXIS2_PLACEMENT_3D('',#8537,#4351,#4352);
#4136=DIRECTION('axis',(0.,0.,1.));
#4137=DIRECTION('refdir',(1.,0.,0.));
#4138=DIRECTION('center_axis',(0.,-1.,0.));
#4139=DIRECTION('ref_axis',(1.,0.,4.82166445138931E-17));
#4140=DIRECTION('',(0.,1.,0.));
#4141=DIRECTION('',(0.,1.,0.));
#4142=DIRECTION('center_axis',(0.,-1.,0.));
#4143=DIRECTION('ref_axis',(1.,0.,4.82166445138931E-17));
#4144=DIRECTION('',(0.,1.,0.));
#4145=DIRECTION('center_axis',(0.,-1.,0.));
#4146=DIRECTION('ref_axis',(1.,0.,4.82166445138931E-17));
#4147=DIRECTION('',(0.,1.,0.));
#4148=DIRECTION('center_axis',(0.,-1.,0.));
#4149=DIRECTION('ref_axis',(1.,0.,4.82166445138931E-17));
#4150=DIRECTION('',(0.,1.,0.));
#4151=DIRECTION('center_axis',(0.,-1.,0.));
#4152=DIRECTION('ref_axis',(1.,0.,4.82166445138931E-17));
#4153=DIRECTION('',(0.,1.,0.));
#4154=DIRECTION('center_axis',(0.,-1.,0.));
#4155=DIRECTION('ref_axis',(1.,0.,4.82166445138931E-17));
#4156=DIRECTION('',(0.,1.,0.));
#4157=DIRECTION('center_axis',(0.,-1.,0.));
#4158=DIRECTION('ref_axis',(1.,0.,4.82166445138931E-17));
#4159=DIRECTION('',(0.,1.,0.));
#4160=DIRECTION('center_axis',(0.,-1.,0.));
#4161=DIRECTION('ref_axis',(1.,0.,4.82166445138931E-17));
#4162=DIRECTION('',(0.,1.,0.));
#4163=DIRECTION('center_axis',(0.,-1.,0.));
#4164=DIRECTION('ref_axis',(1.,0.,4.82166445138931E-17));
#4165=DIRECTION('',(0.,1.,0.));
#4166=DIRECTION('center_axis',(0.,-1.,0.));
#4167=DIRECTION('ref_axis',(1.,0.,4.82166445138931E-17));
#4168=DIRECTION('',(0.,1.,0.));
#4169=DIRECTION('center_axis',(0.,-1.,0.));
#4170=DIRECTION('ref_axis',(1.,0.,4.82166445138931E-17));
#4171=DIRECTION('',(0.,1.,0.));
#4172=DIRECTION('center_axis',(0.,-1.,0.));
#4173=DIRECTION('ref_axis',(1.,0.,4.82166445138931E-17));
#4174=DIRECTION('',(0.,1.,0.));
#4175=DIRECTION('center_axis',(0.,-1.,0.));
#4176=DIRECTION('ref_axis',(1.,0.,4.82166445138931E-17));
#4177=DIRECTION('',(0.,1.,0.));
#4178=DIRECTION('center_axis',(0.,-1.,0.));
#4179=DIRECTION('ref_axis',(1.,0.,4.82166445138931E-17));
#4180=DIRECTION('',(0.,1.,0.));
#4181=DIRECTION('center_axis',(0.,-1.,0.));
#4182=DIRECTION('ref_axis',(1.,0.,4.82166445138931E-17));
#4183=DIRECTION('',(0.,1.,0.));
#4184=DIRECTION('center_axis',(0.,-1.,0.));
#4185=DIRECTION('ref_axis',(1.,0.,4.82166445138931E-17));
#4186=DIRECTION('',(0.,1.,0.));
#4187=DIRECTION('center_axis',(0.,-1.,0.));
#4188=DIRECTION('ref_axis',(1.,0.,4.82166445138931E-17));
#4189=DIRECTION('',(0.,1.,0.));
#4190=DIRECTION('center_axis',(0.,-1.,0.));
#4191=DIRECTION('ref_axis',(1.,0.,4.82166445138931E-17));
#4192=DIRECTION('',(0.,1.,0.));
#4193=DIRECTION('center_axis',(0.,-1.,0.));
#4194=DIRECTION('ref_axis',(1.,0.,4.82166445138931E-17));
#4195=DIRECTION('',(0.,1.,0.));
#4196=DIRECTION('center_axis',(0.,-1.,0.));
#4197=DIRECTION('ref_axis',(1.,0.,4.82166445138931E-17));
#4198=DIRECTION('',(0.,1.,0.));
#4199=DIRECTION('center_axis',(0.,-1.,0.));
#4200=DIRECTION('ref_axis',(1.,0.,4.82166445138931E-17));
#4201=DIRECTION('',(0.,1.,0.));
#4202=DIRECTION('center_axis',(0.,-1.,0.));
#4203=DIRECTION('ref_axis',(1.,0.,4.82166445138931E-17));
#4204=DIRECTION('',(0.,1.,0.));
#4205=DIRECTION('center_axis',(0.,-1.,0.));
#4206=DIRECTION('ref_axis',(1.,0.,4.82166445138931E-17));
#4207=DIRECTION('',(0.,1.,0.));
#4208=DIRECTION('center_axis',(0.,-1.,0.));
#4209=DIRECTION('ref_axis',(1.,0.,4.82166445138931E-17));
#4210=DIRECTION('',(0.,1.,0.));
#4211=DIRECTION('center_axis',(0.,-1.,0.));
#4212=DIRECTION('ref_axis',(1.,0.,4.82166445138931E-17));
#4213=DIRECTION('',(0.,1.,0.));
#4214=DIRECTION('center_axis',(0.,-1.,0.));
#4215=DIRECTION('ref_axis',(1.,0.,4.82166445138931E-17));
#4216=DIRECTION('',(0.,1.,0.));
#4217=DIRECTION('center_axis',(0.,-1.,0.));
#4218=DIRECTION('ref_axis',(1.,0.,4.82166445138931E-17));
#4219=DIRECTION('',(0.,1.,0.));
#4220=DIRECTION('center_axis',(0.,1.,0.));
#4221=DIRECTION('ref_axis',(0.,0.,1.));
#4222=DIRECTION('',(0.,-1.,0.));
#4223=DIRECTION('center_axis',(-2.67523620391605E-16,-1.,0.));
#4224=DIRECTION('ref_axis',(1.,-2.67523620391605E-16,0.));
#4225=DIRECTION('center_axis',(0.,1.,0.));
#4226=DIRECTION('ref_axis',(0.,0.,1.));
#4227=DIRECTION('',(0.,-1.,0.));
#4228=DIRECTION('center_axis',(-2.67523620391605E-16,-1.,0.));
#4229=DIRECTION('ref_axis',(1.,-2.67523620391605E-16,0.));
#4230=DIRECTION('',(0.,1.,0.));
#4231=DIRECTION('center_axis',(0.,1.,0.));
#4232=DIRECTION('ref_axis',(0.,0.,1.));
#4233=DIRECTION('',(0.,-1.,0.));
#4234=DIRECTION('center_axis',(0.,1.,0.));
#4235=DIRECTION('ref_axis',(0.,0.,1.));
#4236=DIRECTION('',(0.,-1.,0.));
#4237=DIRECTION('center_axis',(0.,1.,0.));
#4238=DIRECTION('ref_axis',(0.,0.,1.));
#4239=DIRECTION('',(0.,-1.,0.));
#4240=DIRECTION('center_axis',(0.,1.,0.));
#4241=DIRECTION('ref_axis',(0.,0.,1.));
#4242=DIRECTION('',(0.,-1.,0.));
#4243=DIRECTION('center_axis',(0.,1.,0.));
#4244=DIRECTION('ref_axis',(0.,0.,1.));
#4245=DIRECTION('',(0.,-1.,0.));
#4246=DIRECTION('center_axis',(0.,1.,0.));
#4247=DIRECTION('ref_axis',(0.,0.,1.));
#4248=DIRECTION('',(0.,-1.,0.));
#4249=DIRECTION('center_axis',(0.,1.,0.));
#4250=DIRECTION('ref_axis',(0.,0.,1.));
#4251=DIRECTION('',(0.,-1.,0.));
#4252=DIRECTION('center_axis',(0.,1.,0.));
#4253=DIRECTION('ref_axis',(0.,0.,1.));
#4254=DIRECTION('',(0.,-1.,0.));
#4255=DIRECTION('center_axis',(0.,1.,0.));
#4256=DIRECTION('ref_axis',(0.,0.,1.));
#4257=DIRECTION('',(0.,-1.,0.));
#4258=DIRECTION('center_axis',(0.,1.,0.));
#4259=DIRECTION('ref_axis',(0.,0.,1.));
#4260=DIRECTION('',(0.,-1.,0.));
#4261=DIRECTION('center_axis',(0.,1.,0.));
#4262=DIRECTION('ref_axis',(0.,0.,1.));
#4263=DIRECTION('',(0.,-1.,0.));
#4264=DIRECTION('center_axis',(0.,1.,0.));
#4265=DIRECTION('ref_axis',(0.,0.,1.));
#4266=DIRECTION('',(0.,-1.,0.));
#4267=DIRECTION('center_axis',(0.,1.,0.));
#4268=DIRECTION('ref_axis',(0.,0.,1.));
#4269=DIRECTION('',(0.,-1.,0.));
#4270=DIRECTION('center_axis',(0.,1.,0.));
#4271=DIRECTION('ref_axis',(0.,0.,1.));
#4272=DIRECTION('',(0.,-1.,0.));
#4273=DIRECTION('center_axis',(0.,1.,0.));
#4274=DIRECTION('ref_axis',(0.,0.,1.));
#4275=DIRECTION('',(0.,-1.,0.));
#4276=DIRECTION('center_axis',(0.,1.,0.));
#4277=DIRECTION('ref_axis',(0.,0.,1.));
#4278=DIRECTION('',(0.,-1.,0.));
#4279=DIRECTION('center_axis',(0.,1.,0.));
#4280=DIRECTION('ref_axis',(0.,0.,1.));
#4281=DIRECTION('',(0.,-1.,0.));
#4282=DIRECTION('center_axis',(0.,1.,0.));
#4283=DIRECTION('ref_axis',(0.,0.,1.));
#4284=DIRECTION('',(0.,-1.,0.));
#4285=DIRECTION('center_axis',(0.,1.,0.));
#4286=DIRECTION('ref_axis',(0.,0.,1.));
#4287=DIRECTION('',(0.,-1.,0.));
#4288=DIRECTION('center_axis',(0.,1.,0.));
#4289=DIRECTION('ref_axis',(0.,0.,1.));
#4290=DIRECTION('',(0.,-1.,0.));
#4291=DIRECTION('center_axis',(0.,1.,0.));
#4292=DIRECTION('ref_axis',(0.,0.,1.));
#4293=DIRECTION('',(0.,-1.,0.));
#4294=DIRECTION('center_axis',(0.,1.,0.));
#4295=DIRECTION('ref_axis',(0.,0.,1.));
#4296=DIRECTION('',(0.,-1.,0.));
#4297=DIRECTION('center_axis',(0.,1.,0.));
#4298=DIRECTION('ref_axis',(0.,0.,1.));
#4299=DIRECTION('',(0.,-1.,0.));
#4300=DIRECTION('center_axis',(0.,1.,0.));
#4301=DIRECTION('ref_axis',(0.,0.,1.));
#4302=DIRECTION('',(0.,-1.,0.));
#4303=DIRECTION('center_axis',(0.,1.,0.));
#4304=DIRECTION('ref_axis',(0.,0.,1.));
#4305=DIRECTION('center_axis',(0.,-1.,0.));
#4306=DIRECTION('ref_axis',(0.,0.,-1.));
#4307=DIRECTION('',(0.,-1.,0.));
#4308=DIRECTION('',(0.,-1.,0.));
#4309=DIRECTION('',(0.,-1.,0.));
#4310=DIRECTION('center_axis',(0.,0.,1.));
#4311=DIRECTION('ref_axis',(1.,0.,0.));
#4312=DIRECTION('center_axis',(2.67523620391605E-16,1.,0.));
#4313=DIRECTION('ref_axis',(-1.,2.67523620391605E-16,0.));
#4314=DIRECTION('center_axis',(0.,0.,-1.));
#4315=DIRECTION('ref_axis',(1.,0.,0.));
#4316=DIRECTION('center_axis',(-2.67523620391605E-16,-1.,0.));
#4317=DIRECTION('ref_axis',(1.,-2.67523620391605E-16,0.));
#4318=DIRECTION('center_axis',(-2.67523620391605E-16,-1.,0.));
#4319=DIRECTION('ref_axis',(1.,-2.67523620391605E-16,0.));
#4320=DIRECTION('center_axis',(0.,1.,0.));
#4321=DIRECTION('ref_axis',(0.,0.,1.));
#4322=DIRECTION('center_axis',(0.,1.,0.));
#4323=DIRECTION('ref_axis',(0.,0.,1.));
#4324=DIRECTION('center_axis',(0.,-1.,0.));
#4325=DIRECTION('ref_axis',(0.,0.,-1.));
#4326=DIRECTION('',(0.,-1.,0.));
#4327=DIRECTION('center_axis',(0.,-1.,0.));
#4328=DIRECTION('ref_axis',(0.,0.,-1.));
#4329=DIRECTION('center_axis',(0.,1.,0.));
#4330=DIRECTION('ref_axis',(0.,0.,1.));
#4331=DIRECTION('',(0.,-1.,0.));
#4332=DIRECTION('center_axis',(0.,-1.,0.));
#4333=DIRECTION('ref_axis',(0.,0.,-1.));
#4334=DIRECTION('center_axis',(2.67523620391605E-16,1.,0.));
#4335=DIRECTION('ref_axis',(-1.,2.67523620391605E-16,0.));
#4336=DIRECTION('center_axis',(0.,-1.,0.));
#4337=DIRECTION('ref_axis',(0.,0.,-1.));
#4338=DIRECTION('center_axis',(0.,-1.,0.));
#4339=DIRECTION('ref_axis',(0.,0.,-1.));
#4340=DIRECTION('center_axis',(-2.67523620391605E-16,-1.,0.));
#4341=DIRECTION('ref_axis',(1.,-2.67523620391605E-16,0.));
#4342=DIRECTION('center_axis',(0.,0.,1.));
#4343=DIRECTION('ref_axis',(1.,0.,0.));
#4344=DIRECTION('',(0.86602540378444,-0.499999999999998,0.));
#4345=DIRECTION('',(0.,-1.,0.));
#4346=DIRECTION('',(-0.86602540378444,-0.499999999999998,0.));
#4347=DIRECTION('center_axis',(-0.866025403784434,0.,-0.500000000000008));
#4348=DIRECTION('ref_axis',(-0.500000000000008,0.,0.866025403784434));
#4349=DIRECTION('',(0.433012701892227,0.499999999999977,-0.750000000000011));
#4350=DIRECTION('',(-0.433012701892221,0.500000000000001,0.749999999999999));
#4351=DIRECTION('center_axis',(0.,-1.,0.));
#4352=DIRECTION('ref_axis',(1.,0.,4.82166445138931E-17));
#4994=CARTESIAN_POINT('',(0.,0.,0.));
#4995=CARTESIAN_POINT('Origin',(-2.22044604925031E-15,50.1968749993855,
-2.77555756156289E-16));
#4996=CARTESIAN_POINT('',(-5.75643035625,62.0656249993855,-9.82515157185911E-16));
#4997=CARTESIAN_POINT('',(-5.75643035625,62.1781249993855,-9.82515157185911E-16));
#4998=CARTESIAN_POINT('',(-5.75643035625,50.1968749993855,-1.2600709133422E-15));
#4999=CARTESIAN_POINT('',(-2.878215178125,62.1406249993855,4.9852149236284));
#5000=CARTESIAN_POINT('Ctrl Pts',(-5.75643035625,62.0656249993855,-7.04959401029622E-16));
#5001=CARTESIAN_POINT('Ctrl Pts',(-5.75643035625,62.1031249993855,3.32347661575227));
#5002=CARTESIAN_POINT('Ctrl Pts',(-2.878215178125,62.1406249993855,4.9852149236284));
#5003=CARTESIAN_POINT('',(-2.878215178125,62.2531249993855,4.9852149236284));
#5004=CARTESIAN_POINT('',(-2.878215178125,62.1406249993855,4.9852149236284));
#5005=CARTESIAN_POINT('Ctrl Pts',(-5.75643035625,62.1781249993855,-7.04959401029622E-16));
#5006=CARTESIAN_POINT('Ctrl Pts',(-5.75643035625,62.2156249993855,3.32347661575227));
#5007=CARTESIAN_POINT('Ctrl Pts',(-2.878215178125,62.2531249993855,4.9852149236284));
#5008=CARTESIAN_POINT('Origin',(-2.22044604925031E-15,50.1968749993855,
-2.77555756156289E-16));
#5009=CARTESIAN_POINT('',(-5.75643035625,61.6156249993855,-9.82515157185911E-16));
#5010=CARTESIAN_POINT('',(-5.75643035625,61.7281249993855,-9.82515157185911E-16));
#5011=CARTESIAN_POINT('',(-5.75643035625,50.1968749993855,-1.2600709133422E-15));
#5012=CARTESIAN_POINT('Ctrl Pts',(-5.75643035625,61.6156249993855,-7.04959401029622E-16));
#5013=CARTESIAN_POINT('Ctrl Pts',(-5.75643035625,61.6531249993855,3.32347661575227));
#5014=CARTESIAN_POINT('Ctrl Pts',(-2.878215178125,61.6906249993855,4.9852149236284));
#5015=CARTESIAN_POINT('Ctrl Pts',(-1.22102549985663E-15,61.7281249993855,
6.64695323150454));
#5016=CARTESIAN_POINT('Ctrl Pts',(2.878215178125,61.7656249993855,4.98521492362841));
#5017=CARTESIAN_POINT('Ctrl Pts',(5.75643035625,61.8031249993855,3.32347661575227));
#5018=CARTESIAN_POINT('Ctrl Pts',(5.75643035625,61.8406249993855,0.));
#5019=CARTESIAN_POINT('Ctrl Pts',(5.75643035625,61.8781249993855,-3.32347661575227));
#5020=CARTESIAN_POINT('Ctrl Pts',(2.878215178125,61.9156249993855,-4.9852149236284));
#5021=CARTESIAN_POINT('Ctrl Pts',(4.0700849995221E-16,61.9531249993855,
-6.64695323150454));
#5022=CARTESIAN_POINT('Ctrl Pts',(-2.878215178125,61.9906249993855,-4.9852149236284));
#5023=CARTESIAN_POINT('Ctrl Pts',(-5.75643035625,62.0281249993855,-3.32347661575227));
#5024=CARTESIAN_POINT('Ctrl Pts',(-5.75643035625,62.0656249993855,-7.04959401029622E-16));
#5025=CARTESIAN_POINT('Ctrl Pts',(-5.75643035625,61.7281249993855,-7.04959401029622E-16));
#5026=CARTESIAN_POINT('Ctrl Pts',(-5.75643035625,61.7656249993855,3.32347661575227));
#5027=CARTESIAN_POINT('Ctrl Pts',(-2.878215178125,61.8031249993855,4.9852149236284));
#5028=CARTESIAN_POINT('Ctrl Pts',(-1.22102549985663E-15,61.8406249993855,
6.64695323150454));
#5029=CARTESIAN_POINT('Ctrl Pts',(2.878215178125,61.8781249993855,4.98521492362841));
#5030=CARTESIAN_POINT('Ctrl Pts',(5.75643035625,61.9156249993855,3.32347661575227));
#5031=CARTESIAN_POINT('Ctrl Pts',(5.75643035625,61.9531249993855,0.));
#5032=CARTESIAN_POINT('Ctrl Pts',(5.75643035625,61.9906249993855,-3.32347661575227));
#5033=CARTESIAN_POINT('Ctrl Pts',(2.878215178125,62.0281249993855,-4.9852149236284));
#5034=CARTESIAN_POINT('Ctrl Pts',(4.0700849995221E-16,62.0656249993855,
-6.64695323150454));
#5035=CARTESIAN_POINT('Ctrl Pts',(-2.878215178125,62.1031249993855,-4.9852149236284));
#5036=CARTESIAN_POINT('Ctrl Pts',(-5.75643035625,62.1406249993855,-3.32347661575227));
#5037=CARTESIAN_POINT('Ctrl Pts',(-5.75643035625,62.1781249993855,-7.04959401029622E-16));
#5038=CARTESIAN_POINT('Origin',(-2.22044604925031E-15,50.1968749993855,
-2.77555756156289E-16));
#5039=CARTESIAN_POINT('',(-5.75643035625,61.1656249993855,-9.82515157185911E-16));
#5040=CARTESIAN_POINT('',(-5.75643035625,61.2781249993855,-9.82515157185911E-16));
#5041=CARTESIAN_POINT('',(-5.75643035625,50.1968749993855,-1.2600709133422E-15));
#5042=CARTESIAN_POINT('Ctrl Pts',(-5.75643035625,61.1656249993855,-7.04959401029622E-16));
#5043=CARTESIAN_POINT('Ctrl Pts',(-5.75643035625,61.2031249993855,3.32347661575227));
#5044=CARTESIAN_POINT('Ctrl Pts',(-2.878215178125,61.2406249993855,4.9852149236284));
#5045=CARTESIAN_POINT('Ctrl Pts',(-1.22102549985663E-15,61.2781249993855,
6.64695323150454));
#5046=CARTESIAN_POINT('Ctrl Pts',(2.878215178125,61.3156249993855,4.98521492362841));
#5047=CARTESIAN_POINT('Ctrl Pts',(5.75643035625,61.3531249993855,3.32347661575227));
#5048=CARTESIAN_POINT('Ctrl Pts',(5.75643035625,61.3906249993855,0.));
#5049=CARTESIAN_POINT('Ctrl Pts',(5.75643035625,61.4281249993855,-3.32347661575227));
#5050=CARTESIAN_POINT('Ctrl Pts',(2.878215178125,61.4656249993855,-4.9852149236284));
#5051=CARTESIAN_POINT('Ctrl Pts',(4.0700849995221E-16,61.5031249993855,
-6.64695323150454));
#5052=CARTESIAN_POINT('Ctrl Pts',(-2.878215178125,61.5406249993855,-4.9852149236284));
#5053=CARTESIAN_POINT('Ctrl Pts',(-5.75643035625,61.5781249993855,-3.32347661575227));
#5054=CARTESIAN_POINT('Ctrl Pts',(-5.75643035625,61.6156249993855,-7.04959401029622E-16));
#5055=CARTESIAN_POINT('Ctrl Pts',(-5.75643035625,61.2781249993855,-7.04959401029622E-16));
#5056=CARTESIAN_POINT('Ctrl Pts',(-5.75643035625,61.3156249993855,3.32347661575227));
#5057=CARTESIAN_POINT('Ctrl Pts',(-2.878215178125,61.3531249993855,4.9852149236284));
#5058=CARTESIAN_POINT('Ctrl Pts',(-1.22102549985663E-15,61.3906249993855,
6.64695323150454));
#5059=CARTESIAN_POINT('Ctrl Pts',(2.878215178125,61.4281249993855,4.98521492362841));
#5060=CARTESIAN_POINT('Ctrl Pts',(5.75643035625,61.4656249993855,3.32347661575227));
#5061=CARTESIAN_POINT('Ctrl Pts',(5.75643035625,61.5031249993855,0.));
#5062=CARTESIAN_POINT('Ctrl Pts',(5.75643035625,61.5406249993855,-3.32347661575227));
#5063=CARTESIAN_POINT('Ctrl Pts',(2.878215178125,61.5781249993855,-4.9852149236284));
#5064=CARTESIAN_POINT('Ctrl Pts',(4.0700849995221E-16,61.6156249993855,
-6.64695323150454));
#5065=CARTESIAN_POINT('Ctrl Pts',(-2.878215178125,61.6531249993855,-4.9852149236284));
#5066=CARTESIAN_POINT('Ctrl Pts',(-5.75643035625,61.6906249993855,-3.32347661575227));
#5067=CARTESIAN_POINT('Ctrl Pts',(-5.75643035625,61.7281249993855,-7.04959401029622E-16));
#5068=CARTESIAN_POINT('Origin',(-2.22044604925031E-15,50.1968749993855,
-2.77555756156289E-16));
#5069=CARTESIAN_POINT('',(-5.75643035625,60.7156249993855,-9.82515157185911E-16));
#5070=CARTESIAN_POINT('',(-5.75643035625,60.8281249993855,-9.82515157185911E-16));
#5071=CARTESIAN_POINT('',(-5.75643035625,50.1968749993855,-1.2600709133422E-15));
#5072=CARTESIAN_POINT('Ctrl Pts',(-5.75643035625,60.7156249993855,-7.04959401029622E-16));
#5073=CARTESIAN_POINT('Ctrl Pts',(-5.75643035625,60.7531249993855,3.32347661575227));
#5074=CARTESIAN_POINT('Ctrl Pts',(-2.878215178125,60.7906249993855,4.9852149236284));
#5075=CARTESIAN_POINT('Ctrl Pts',(-1.22102549985663E-15,60.8281249993855,
6.64695323150454));
#5076=CARTESIAN_POINT('Ctrl Pts',(2.878215178125,60.8656249993855,4.98521492362841));
#5077=CARTESIAN_POINT('Ctrl Pts',(5.75643035625,60.9031249993855,3.32347661575227));
#5078=CARTESIAN_POINT('Ctrl Pts',(5.75643035625,60.9406249993855,0.));
#5079=CARTESIAN_POINT('Ctrl Pts',(5.75643035625,60.9781249993855,-3.32347661575227));
#5080=CARTESIAN_POINT('Ctrl Pts',(2.878215178125,61.0156249993855,-4.9852149236284));
#5081=CARTESIAN_POINT('Ctrl Pts',(4.0700849995221E-16,61.0531249993855,
-6.64695323150454));
#5082=CARTESIAN_POINT('Ctrl Pts',(-2.878215178125,61.0906249993855,-4.9852149236284));
#5083=CARTESIAN_POINT('Ctrl Pts',(-5.75643035625,61.1281249993855,-3.32347661575227));
#5084=CARTESIAN_POINT('Ctrl Pts',(-5.75643035625,61.1656249993855,-7.04959401029622E-16));
#5085=CARTESIAN_POINT('Ctrl Pts',(-5.75643035625,60.8281249993855,-7.04959401029622E-16));
#5086=CARTESIAN_POINT('Ctrl Pts',(-5.75643035625,60.8656249993855,3.32347661575227));
#5087=CARTESIAN_POINT('Ctrl Pts',(-2.878215178125,60.9031249993855,4.9852149236284));
#5088=CARTESIAN_POINT('Ctrl Pts',(-1.22102549985663E-15,60.9406249993855,
6.64695323150454));
#5089=CARTESIAN_POINT('Ctrl Pts',(2.878215178125,60.9781249993855,4.98521492362841));
#5090=CARTESIAN_POINT('Ctrl Pts',(5.75643035625,61.0156249993855,3.32347661575227));
#5091=CARTESIAN_POINT('Ctrl Pts',(5.75643035625,61.0531249993855,0.));
#5092=CARTESIAN_POINT('Ctrl Pts',(5.75643035625,61.0906249993855,-3.32347661575227));
#5093=CARTESIAN_POINT('Ctrl Pts',(2.878215178125,61.1281249993855,-4.9852149236284));
#5094=CARTESIAN_POINT('Ctrl Pts',(4.0700849995221E-16,61.1656249993855,
-6.64695323150454));
#5095=CARTESIAN_POINT('Ctrl Pts',(-2.878215178125,61.2031249993855,-4.9852149236284));
#5096=CARTESIAN_POINT('Ctrl Pts',(-5.75643035625,61.2406249993855,-3.32347661575227));
#5097=CARTESIAN_POINT('Ctrl Pts',(-5.75643035625,61.2781249993855,-7.04959401029622E-16));
#5098=CARTESIAN_POINT('Origin',(-2.22044604925031E-15,50.1968749993855,
-2.77555756156289E-16));
#5099=CARTESIAN_POINT('',(-5.75643035625,60.2656249993855,-9.82515157185911E-16));
#5100=CARTESIAN_POINT('',(-5.75643035625,60.3781249993855,-9.82515157185911E-16));
#5101=CARTESIAN_POINT('',(-5.75643035625,50.1968749993855,-1.2600709133422E-15));
#5102=CARTESIAN_POINT('Ctrl Pts',(-5.75643035625,60.2656249993855,-7.04959401029622E-16));
#5103=CARTESIAN_POINT('Ctrl Pts',(-5.75643035625,60.3031249993855,3.32347661575227));
#5104=CARTESIAN_POINT('Ctrl Pts',(-2.878215178125,60.3406249993855,4.9852149236284));
#5105=CARTESIAN_POINT('Ctrl Pts',(-1.22102549985663E-15,60.3781249993855,
6.64695323150454));
#5106=CARTESIAN_POINT('Ctrl Pts',(2.878215178125,60.4156249993855,4.98521492362841));
#5107=CARTESIAN_POINT('Ctrl Pts',(5.75643035625,60.4531249993855,3.32347661575227));
#5108=CARTESIAN_POINT('Ctrl Pts',(5.75643035625,60.4906249993855,0.));
#5109=CARTESIAN_POINT('Ctrl Pts',(5.75643035625,60.5281249993855,-3.32347661575227));
#5110=CARTESIAN_POINT('Ctrl Pts',(2.878215178125,60.5656249993855,-4.9852149236284));
#5111=CARTESIAN_POINT('Ctrl Pts',(4.0700849995221E-16,60.6031249993855,
-6.64695323150454));
#5112=CARTESIAN_POINT('Ctrl Pts',(-2.878215178125,60.6406249993855,-4.9852149236284));
#5113=CARTESIAN_POINT('Ctrl Pts',(-5.75643035625,60.6781249993855,-3.32347661575227));
#5114=CARTESIAN_POINT('Ctrl Pts',(-5.75643035625,60.7156249993855,-7.04959401029622E-16));
#5115=CARTESIAN_POINT('Ctrl Pts',(-5.75643035625,60.3781249993855,-7.04959401029622E-16));
#5116=CARTESIAN_POINT('Ctrl Pts',(-5.75643035625,60.4156249993855,3.32347661575227));
#5117=CARTESIAN_POINT('Ctrl Pts',(-2.878215178125,60.4531249993855,4.9852149236284));
#5118=CARTESIAN_POINT('Ctrl Pts',(-1.22102549985663E-15,60.4906249993855,
6.64695323150454));
#5119=CARTESIAN_POINT('Ctrl Pts',(2.878215178125,60.5281249993855,4.98521492362841));
#5120=CARTESIAN_POINT('Ctrl Pts',(5.75643035625,60.5656249993855,3.32347661575227));
#5121=CARTESIAN_POINT('Ctrl Pts',(5.75643035625,60.6031249993855,0.));
#5122=CARTESIAN_POINT('Ctrl Pts',(5.75643035625,60.6406249993855,-3.32347661575227));
#5123=CARTESIAN_POINT('Ctrl Pts',(2.878215178125,60.6781249993855,-4.9852149236284));
#5124=CARTESIAN_POINT('Ctrl Pts',(4.0700849995221E-16,60.7156249993855,
-6.64695323150454));
#5125=CARTESIAN_POINT('Ctrl Pts',(-2.878215178125,60.7531249993855,-4.9852149236284));
#5126=CARTESIAN_POINT('Ctrl Pts',(-5.75643035625,60.7906249993855,-3.32347661575227));
#5127=CARTESIAN_POINT('Ctrl Pts',(-5.75643035625,60.8281249993855,-7.04959401029622E-16));
#5128=CARTESIAN_POINT('Origin',(-2.22044604925031E-15,50.1968749993855,
-2.77555756156289E-16));
#5129=CARTESIAN_POINT('',(-5.75643035625,59.8156249993855,-9.82515157185911E-16));
#5130=CARTESIAN_POINT('',(-5.75643035625,59.9281249993855,-9.82515157185911E-16));
#5131=CARTESIAN_POINT('',(-5.75643035625,50.1968749993855,-1.2600709133422E-15));
#5132=CARTESIAN_POINT('Ctrl Pts',(-5.75643035625,59.8156249993855,-7.04959401029622E-16));
#5133=CARTESIAN_POINT('Ctrl Pts',(-5.75643035625,59.8531249993855,3.32347661575227));
#5134=CARTESIAN_POINT('Ctrl Pts',(-2.878215178125,59.8906249993855,4.9852149236284));
#5135=CARTESIAN_POINT('Ctrl Pts',(-1.22102549985663E-15,59.9281249993855,
6.64695323150454));
#5136=CARTESIAN_POINT('Ctrl Pts',(2.878215178125,59.9656249993855,4.98521492362841));
#5137=CARTESIAN_POINT('Ctrl Pts',(5.75643035625,60.0031249993855,3.32347661575227));
#5138=CARTESIAN_POINT('Ctrl Pts',(5.75643035625,60.0406249993855,0.));
#5139=CARTESIAN_POINT('Ctrl Pts',(5.75643035625,60.0781249993855,-3.32347661575227));
#5140=CARTESIAN_POINT('Ctrl Pts',(2.878215178125,60.1156249993855,-4.9852149236284));
#5141=CARTESIAN_POINT('Ctrl Pts',(4.0700849995221E-16,60.1531249993855,
-6.64695323150454));
#5142=CARTESIAN_POINT('Ctrl Pts',(-2.878215178125,60.1906249993855,-4.9852149236284));
#5143=CARTESIAN_POINT('Ctrl Pts',(-5.75643035625,60.2281249993855,-3.32347661575227));
#5144=CARTESIAN_POINT('Ctrl Pts',(-5.75643035625,60.2656249993855,-7.04959401029622E-16));
#5145=CARTESIAN_POINT('Ctrl Pts',(-5.75643035625,59.9281249993855,-7.04959401029622E-16));
#5146=CARTESIAN_POINT('Ctrl Pts',(-5.75643035625,59.9656249993855,3.32347661575227));
#5147=CARTESIAN_POINT('Ctrl Pts',(-2.878215178125,60.0031249993855,4.9852149236284));
#5148=CARTESIAN_POINT('Ctrl Pts',(-1.22102549985663E-15,60.0406249993855,
6.64695323150454));
#5149=CARTESIAN_POINT('Ctrl Pts',(2.878215178125,60.0781249993855,4.98521492362841));
#5150=CARTESIAN_POINT('Ctrl Pts',(5.75643035625,60.1156249993855,3.32347661575227));
#5151=CARTESIAN_POINT('Ctrl Pts',(5.75643035625,60.1531249993855,0.));
#5152=CARTESIAN_POINT('Ctrl Pts',(5.75643035625,60.1906249993855,-3.32347661575227));
#5153=CARTESIAN_POINT('Ctrl Pts',(2.878215178125,60.2281249993855,-4.9852149236284));
#5154=CARTESIAN_POINT('Ctrl Pts',(4.0700849995221E-16,60.2656249993855,
-6.64695323150454));
#5155=CARTESIAN_POINT('Ctrl Pts',(-2.878215178125,60.3031249993855,-4.9852149236284));
#5156=CARTESIAN_POINT('Ctrl Pts',(-5.75643035625,60.3406249993855,-3.32347661575227));
#5157=CARTESIAN_POINT('Ctrl Pts',(-5.75643035625,60.3781249993855,-7.04959401029622E-16));
#5158=CARTESIAN_POINT('Origin',(-2.22044604925031E-15,50.1968749993855,
-2.77555756156289E-16));
#5159=CARTESIAN_POINT('',(-5.75643035625,59.3656249993855,-9.82515157185911E-16));
#5160=CARTESIAN_POINT('',(-5.75643035625,59.4781249993855,-9.82515157185911E-16));
#5161=CARTESIAN_POINT('',(-5.75643035625,50.1968749993855,-1.2600709133422E-15));
#5162=CARTESIAN_POINT('Ctrl Pts',(-5.75643035625,59.3656249993855,-7.04959401029622E-16));
#5163=CARTESIAN_POINT('Ctrl Pts',(-5.75643035625,59.4031249993855,3.32347661575227));
#5164=CARTESIAN_POINT('Ctrl Pts',(-2.878215178125,59.4406249993855,4.9852149236284));
#5165=CARTESIAN_POINT('Ctrl Pts',(-1.22102549985663E-15,59.4781249993855,
6.64695323150454));
#5166=CARTESIAN_POINT('Ctrl Pts',(2.878215178125,59.5156249993855,4.98521492362841));
#5167=CARTESIAN_POINT('Ctrl Pts',(5.75643035625,59.5531249993855,3.32347661575227));
#5168=CARTESIAN_POINT('Ctrl Pts',(5.75643035625,59.5906249993855,0.));
#5169=CARTESIAN_POINT('Ctrl Pts',(5.75643035625,59.6281249993855,-3.32347661575227));
#5170=CARTESIAN_POINT('Ctrl Pts',(2.878215178125,59.6656249993855,-4.9852149236284));
#5171=CARTESIAN_POINT('Ctrl Pts',(4.0700849995221E-16,59.7031249993855,
-6.64695323150454));
#5172=CARTESIAN_POINT('Ctrl Pts',(-2.878215178125,59.7406249993855,-4.9852149236284));
#5173=CARTESIAN_POINT('Ctrl Pts',(-5.75643035625,59.7781249993855,-3.32347661575227));
#5174=CARTESIAN_POINT('Ctrl Pts',(-5.75643035625,59.8156249993855,-7.04959401029622E-16));
#5175=CARTESIAN_POINT('Ctrl Pts',(-5.75643035625,59.4781249993855,-7.04959401029622E-16));
#5176=CARTESIAN_POINT('Ctrl Pts',(-5.75643035625,59.5156249993855,3.32347661575227));
#5177=CARTESIAN_POINT('Ctrl Pts',(-2.878215178125,59.5531249993855,4.9852149236284));
#5178=CARTESIAN_POINT('Ctrl Pts',(-1.22102549985663E-15,59.5906249993855,
6.64695323150454));
#5179=CARTESIAN_POINT('Ctrl Pts',(2.878215178125,59.6281249993855,4.98521492362841));
#5180=CARTESIAN_POINT('Ctrl Pts',(5.75643035625,59.6656249993855,3.32347661575227));
#5181=CARTESIAN_POINT('Ctrl Pts',(5.75643035625,59.7031249993855,0.));
#5182=CARTESIAN_POINT('Ctrl Pts',(5.75643035625,59.7406249993855,-3.32347661575227));
#5183=CARTESIAN_POINT('Ctrl Pts',(2.878215178125,59.7781249993855,-4.9852149236284));
#5184=CARTESIAN_POINT('Ctrl Pts',(4.0700849995221E-16,59.8156249993855,
-6.64695323150454));
#5185=CARTESIAN_POINT('Ctrl Pts',(-2.878215178125,59.8531249993855,-4.9852149236284));
#5186=CARTESIAN_POINT('Ctrl Pts',(-5.75643035625,59.8906249993855,-3.32347661575227));
#5187=CARTESIAN_POINT('Ctrl Pts',(-5.75643035625,59.9281249993855,-7.04959401029622E-16));
#5188=CARTESIAN_POINT('Origin',(-2.22044604925031E-15,50.1968749993855,
-2.77555756156289E-16));
#5189=CARTESIAN_POINT('',(-5.75643035625,58.9156249993855,-9.82515157185911E-16));
#5190=CARTESIAN_POINT('',(-5.75643035625,59.0281249993855,-9.82515157185911E-16));
#5191=CARTESIAN_POINT('',(-5.75643035625,50.1968749993855,-1.2600709133422E-15));
#5192=CARTESIAN_POINT('Ctrl Pts',(-5.75643035625,58.9156249993855,-7.04959401029622E-16));
#5193=CARTESIAN_POINT('Ctrl Pts',(-5.75643035625,58.9531249993855,3.32347661575227));
#5194=CARTESIAN_POINT('Ctrl Pts',(-2.878215178125,58.9906249993855,4.9852149236284));
#5195=CARTESIAN_POINT('Ctrl Pts',(-1.22102549985663E-15,59.0281249993855,
6.64695323150454));
#5196=CARTESIAN_POINT('Ctrl Pts',(2.878215178125,59.0656249993855,4.98521492362841));
#5197=CARTESIAN_POINT('Ctrl Pts',(5.75643035625,59.1031249993855,3.32347661575227));
#5198=CARTESIAN_POINT('Ctrl Pts',(5.75643035625,59.1406249993855,0.));
#5199=CARTESIAN_POINT('Ctrl Pts',(5.75643035625,59.1781249993855,-3.32347661575227));
#5200=CARTESIAN_POINT('Ctrl Pts',(2.878215178125,59.2156249993855,-4.9852149236284));
#5201=CARTESIAN_POINT('Ctrl Pts',(4.0700849995221E-16,59.2531249993855,
-6.64695323150454));
#5202=CARTESIAN_POINT('Ctrl Pts',(-2.878215178125,59.2906249993855,-4.9852149236284));
#5203=CARTESIAN_POINT('Ctrl Pts',(-5.75643035625,59.3281249993855,-3.32347661575227));
#5204=CARTESIAN_POINT('Ctrl Pts',(-5.75643035625,59.3656249993855,-7.04959401029622E-16));
#5205=CARTESIAN_POINT('Ctrl Pts',(-5.75643035625,59.0281249993855,-7.04959401029622E-16));
#5206=CARTESIAN_POINT('Ctrl Pts',(-5.75643035625,59.0656249993855,3.32347661575227));
#5207=CARTESIAN_POINT('Ctrl Pts',(-2.878215178125,59.1031249993855,4.9852149236284));
#5208=CARTESIAN_POINT('Ctrl Pts',(-1.22102549985663E-15,59.1406249993855,
6.64695323150454));
#5209=CARTESIAN_POINT('Ctrl Pts',(2.878215178125,59.1781249993855,4.98521492362841));
#5210=CARTESIAN_POINT('Ctrl Pts',(5.75643035625,59.2156249993855,3.32347661575227));
#5211=CARTESIAN_POINT('Ctrl Pts',(5.75643035625,59.2531249993855,0.));
#5212=CARTESIAN_POINT('Ctrl Pts',(5.75643035625,59.2906249993855,-3.32347661575227));
#5213=CARTESIAN_POINT('Ctrl Pts',(2.878215178125,59.3281249993855,-4.9852149236284));
#5214=CARTESIAN_POINT('Ctrl Pts',(4.0700849995221E-16,59.3656249993855,
-6.64695323150454));
#5215=CARTESIAN_POINT('Ctrl Pts',(-2.878215178125,59.4031249993855,-4.9852149236284));
#5216=CARTESIAN_POINT('Ctrl Pts',(-5.75643035625,59.4406249993855,-3.32347661575227));
#5217=CARTESIAN_POINT('Ctrl Pts',(-5.75643035625,59.4781249993855,-7.04959401029622E-16));
#5218=CARTESIAN_POINT('Origin',(-2.22044604925031E-15,50.1968749993855,
-2.77555756156289E-16));
#5219=CARTESIAN_POINT('',(-5.75643035625,58.4656249993855,-9.82515157185911E-16));
#5220=CARTESIAN_POINT('',(-5.75643035625,58.5781249993855,-9.82515157185911E-16));
#5221=CARTESIAN_POINT('',(-5.75643035625,50.1968749993855,-1.2600709133422E-15));
#5222=CARTESIAN_POINT('Ctrl Pts',(-5.75643035625,58.4656249993855,-7.04959401029622E-16));
#5223=CARTESIAN_POINT('Ctrl Pts',(-5.75643035625,58.5031249993855,3.32347661575227));
#5224=CARTESIAN_POINT('Ctrl Pts',(-2.878215178125,58.5406249993855,4.9852149236284));
#5225=CARTESIAN_POINT('Ctrl Pts',(-1.22102549985663E-15,58.5781249993855,
6.64695323150454));
#5226=CARTESIAN_POINT('Ctrl Pts',(2.878215178125,58.6156249993855,4.98521492362841));
#5227=CARTESIAN_POINT('Ctrl Pts',(5.75643035625,58.6531249993855,3.32347661575227));
#5228=CARTESIAN_POINT('Ctrl Pts',(5.75643035625,58.6906249993855,0.));
#5229=CARTESIAN_POINT('Ctrl Pts',(5.75643035625,58.7281249993855,-3.32347661575227));
#5230=CARTESIAN_POINT('Ctrl Pts',(2.878215178125,58.7656249993855,-4.9852149236284));
#5231=CARTESIAN_POINT('Ctrl Pts',(4.0700849995221E-16,58.8031249993855,
-6.64695323150454));
#5232=CARTESIAN_POINT('Ctrl Pts',(-2.878215178125,58.8406249993855,-4.9852149236284));
#5233=CARTESIAN_POINT('Ctrl Pts',(-5.75643035625,58.8781249993855,-3.32347661575227));
#5234=CARTESIAN_POINT('Ctrl Pts',(-5.75643035625,58.9156249993855,-7.04959401029622E-16));
#5235=CARTESIAN_POINT('Ctrl Pts',(-5.75643035625,58.5781249993855,-7.04959401029622E-16));
#5236=CARTESIAN_POINT('Ctrl Pts',(-5.75643035625,58.6156249993855,3.32347661575227));
#5237=CARTESIAN_POINT('Ctrl Pts',(-2.878215178125,58.6531249993855,4.9852149236284));
#5238=CARTESIAN_POINT('Ctrl Pts',(-1.22102549985663E-15,58.6906249993855,
6.64695323150454));
#5239=CARTESIAN_POINT('Ctrl Pts',(2.878215178125,58.7281249993855,4.98521492362841));
#5240=CARTESIAN_POINT('Ctrl Pts',(5.75643035625,58.7656249993855,3.32347661575227));
#5241=CARTESIAN_POINT('Ctrl Pts',(5.75643035625,58.8031249993855,0.));
#5242=CARTESIAN_POINT('Ctrl Pts',(5.75643035625,58.8406249993855,-3.32347661575227));
#5243=CARTESIAN_POINT('Ctrl Pts',(2.878215178125,58.8781249993855,-4.9852149236284));
#5244=CARTESIAN_POINT('Ctrl Pts',(4.0700849995221E-16,58.9156249993855,
-6.64695323150454));
#5245=CARTESIAN_POINT('Ctrl Pts',(-2.878215178125,58.9531249993855,-4.9852149236284));
#5246=CARTESIAN_POINT('Ctrl Pts',(-5.75643035625,58.9906249993855,-3.32347661575227));
#5247=CARTESIAN_POINT('Ctrl Pts',(-5.75643035625,59.0281249993855,-7.04959401029622E-16));
#5248=CARTESIAN_POINT('Origin',(-2.22044604925031E-15,50.1968749993855,
-2.77555756156289E-16));
#5249=CARTESIAN_POINT('',(-5.75643035625,58.0156249993855,-9.82515157185911E-16));
#5250=CARTESIAN_POINT('',(-5.75643035625,58.1281249993855,-9.82515157185911E-16));
#5251=CARTESIAN_POINT('',(-5.75643035625,50.1968749993855,-1.2600709133422E-15));
#5252=CARTESIAN_POINT('Ctrl Pts',(-5.75643035625,58.0156249993855,-7.04959401029622E-16));
#5253=CARTESIAN_POINT('Ctrl Pts',(-5.75643035625,58.0531249993855,3.32347661575227));
#5254=CARTESIAN_POINT('Ctrl Pts',(-2.878215178125,58.0906249993855,4.9852149236284));
#5255=CARTESIAN_POINT('Ctrl Pts',(-1.22102549985663E-15,58.1281249993855,
6.64695323150454));
#5256=CARTESIAN_POINT('Ctrl Pts',(2.878215178125,58.1656249993855,4.98521492362841));
#5257=CARTESIAN_POINT('Ctrl Pts',(5.75643035625,58.2031249993855,3.32347661575227));
#5258=CARTESIAN_POINT('Ctrl Pts',(5.75643035625,58.2406249993855,0.));
#5259=CARTESIAN_POINT('Ctrl Pts',(5.75643035625,58.2781249993855,-3.32347661575227));
#5260=CARTESIAN_POINT('Ctrl Pts',(2.878215178125,58.3156249993855,-4.9852149236284));
#5261=CARTESIAN_POINT('Ctrl Pts',(4.0700849995221E-16,58.3531249993855,
-6.64695323150454));
#5262=CARTESIAN_POINT('Ctrl Pts',(-2.878215178125,58.3906249993855,-4.9852149236284));
#5263=CARTESIAN_POINT('Ctrl Pts',(-5.75643035625,58.4281249993855,-3.32347661575227));
#5264=CARTESIAN_POINT('Ctrl Pts',(-5.75643035625,58.4656249993855,-7.04959401029622E-16));
#5265=CARTESIAN_POINT('Ctrl Pts',(-5.75643035625,58.1281249993855,-7.04959401029622E-16));
#5266=CARTESIAN_POINT('Ctrl Pts',(-5.75643035625,58.1656249993855,3.32347661575227));
#5267=CARTESIAN_POINT('Ctrl Pts',(-2.878215178125,58.2031249993855,4.9852149236284));
#5268=CARTESIAN_POINT('Ctrl Pts',(-1.22102549985663E-15,58.2406249993855,
6.64695323150454));
#5269=CARTESIAN_POINT('Ctrl Pts',(2.878215178125,58.2781249993855,4.98521492362841));
#5270=CARTESIAN_POINT('Ctrl Pts',(5.75643035625,58.3156249993855,3.32347661575227));
#5271=CARTESIAN_POINT('Ctrl Pts',(5.75643035625,58.3531249993855,0.));
#5272=CARTESIAN_POINT('Ctrl Pts',(5.75643035625,58.3906249993855,-3.32347661575227));
#5273=CARTESIAN_POINT('Ctrl Pts',(2.878215178125,58.4281249993855,-4.9852149236284));
#5274=CARTESIAN_POINT('Ctrl Pts',(4.0700849995221E-16,58.4656249993855,
-6.64695323150454));
#5275=CARTESIAN_POINT('Ctrl Pts',(-2.878215178125,58.5031249993855,-4.9852149236284));
#5276=CARTESIAN_POINT('Ctrl Pts',(-5.75643035625,58.5406249993855,-3.32347661575227));
#5277=CARTESIAN_POINT('Ctrl Pts',(-5.75643035625,58.5781249993855,-7.04959401029622E-16));
#5278=CARTESIAN_POINT('Origin',(-2.22044604925031E-15,50.1968749993855,
-2.77555756156289E-16));
#5279=CARTESIAN_POINT('',(-5.75643035625,57.5656249993855,-9.82515157185911E-16));
#5280=CARTESIAN_POINT('',(-5.75643035625,57.6781249993855,-9.82515157185911E-16));
#5281=CARTESIAN_POINT('',(-5.75643035625,50.1968749993855,-1.2600709133422E-15));
#5282=CARTESIAN_POINT('Ctrl Pts',(-5.75643035625,57.5656249993855,-7.04959401029622E-16));
#5283=CARTESIAN_POINT('Ctrl Pts',(-5.75643035625,57.6031249993855,3.32347661575227));
#5284=CARTESIAN_POINT('Ctrl Pts',(-2.878215178125,57.6406249993855,4.9852149236284));
#5285=CARTESIAN_POINT('Ctrl Pts',(-1.22102549985663E-15,57.6781249993855,
6.64695323150454));
#5286=CARTESIAN_POINT('Ctrl Pts',(2.878215178125,57.7156249993855,4.98521492362841));
#5287=CARTESIAN_POINT('Ctrl Pts',(5.75643035625,57.7531249993855,3.32347661575227));
#5288=CARTESIAN_POINT('Ctrl Pts',(5.75643035625,57.7906249993855,0.));
#5289=CARTESIAN_POINT('Ctrl Pts',(5.75643035625,57.8281249993855,-3.32347661575227));
#5290=CARTESIAN_POINT('Ctrl Pts',(2.878215178125,57.8656249993855,-4.9852149236284));
#5291=CARTESIAN_POINT('Ctrl Pts',(4.0700849995221E-16,57.9031249993855,
-6.64695323150454));
#5292=CARTESIAN_POINT('Ctrl Pts',(-2.878215178125,57.9406249993855,-4.9852149236284));
#5293=CARTESIAN_POINT('Ctrl Pts',(-5.75643035625,57.9781249993855,-3.32347661575227));
#5294=CARTESIAN_POINT('Ctrl Pts',(-5.75643035625,58.0156249993855,-7.04959401029622E-16));
#5295=CARTESIAN_POINT('Ctrl Pts',(-5.75643035625,57.6781249993855,-7.04959401029622E-16));
#5296=CARTESIAN_POINT('Ctrl Pts',(-5.75643035625,57.7156249993855,3.32347661575227));
#5297=CARTESIAN_POINT('Ctrl Pts',(-2.878215178125,57.7531249993855,4.9852149236284));
#5298=CARTESIAN_POINT('Ctrl Pts',(-1.22102549985663E-15,57.7906249993855,
6.64695323150454));
#5299=CARTESIAN_POINT('Ctrl Pts',(2.878215178125,57.8281249993855,4.98521492362841));
#5300=CARTESIAN_POINT('Ctrl Pts',(5.75643035625,57.8656249993855,3.32347661575227));
#5301=CARTESIAN_POINT('Ctrl Pts',(5.75643035625,57.9031249993855,0.));
#5302=CARTESIAN_POINT('Ctrl Pts',(5.75643035625,57.9406249993855,-3.32347661575227));
#5303=CARTESIAN_POINT('Ctrl Pts',(2.878215178125,57.9781249993855,-4.9852149236284));
#5304=CARTESIAN_POINT('Ctrl Pts',(4.0700849995221E-16,58.0156249993855,
-6.64695323150454));
#5305=CARTESIAN_POINT('Ctrl Pts',(-2.878215178125,58.0531249993855,-4.9852149236284));
#5306=CARTESIAN_POINT('Ctrl Pts',(-5.75643035625,58.0906249993855,-3.32347661575227));
#5307=CARTESIAN_POINT('Ctrl Pts',(-5.75643035625,58.1281249993855,-7.04959401029622E-16));
#5308=CARTESIAN_POINT('Origin',(-2.22044604925031E-15,50.1968749993855,
-2.77555756156289E-16));
#5309=CARTESIAN_POINT('',(-5.75643035625,57.1156249993855,-9.82515157185911E-16));
#5310=CARTESIAN_POINT('',(-5.75643035625,57.2281249993855,-9.82515157185911E-16));
#5311=CARTESIAN_POINT('',(-5.75643035625,50.1968749993855,-1.2600709133422E-15));
#5312=CARTESIAN_POINT('Ctrl Pts',(-5.75643035625,57.1156249993855,-7.04959401029622E-16));
#5313=CARTESIAN_POINT('Ctrl Pts',(-5.75643035625,57.1531249993855,3.32347661575227));
#5314=CARTESIAN_POINT('Ctrl Pts',(-2.878215178125,57.1906249993855,4.9852149236284));
#5315=CARTESIAN_POINT('Ctrl Pts',(-1.22102549985663E-15,57.2281249993855,
6.64695323150454));
#5316=CARTESIAN_POINT('Ctrl Pts',(2.878215178125,57.2656249993855,4.98521492362841));
#5317=CARTESIAN_POINT('Ctrl Pts',(5.75643035625,57.3031249993855,3.32347661575227));
#5318=CARTESIAN_POINT('Ctrl Pts',(5.75643035625,57.3406249993855,0.));
#5319=CARTESIAN_POINT('Ctrl Pts',(5.75643035625,57.3781249993855,-3.32347661575227));
#5320=CARTESIAN_POINT('Ctrl Pts',(2.878215178125,57.4156249993855,-4.9852149236284));
#5321=CARTESIAN_POINT('Ctrl Pts',(4.0700849995221E-16,57.4531249993855,
-6.64695323150454));
#5322=CARTESIAN_POINT('Ctrl Pts',(-2.878215178125,57.4906249993855,-4.9852149236284));
#5323=CARTESIAN_POINT('Ctrl Pts',(-5.75643035625,57.5281249993855,-3.32347661575227));
#5324=CARTESIAN_POINT('Ctrl Pts',(-5.75643035625,57.5656249993855,-7.04959401029622E-16));
#5325=CARTESIAN_POINT('Ctrl Pts',(-5.75643035625,57.2281249993855,-7.04959401029622E-16));
#5326=CARTESIAN_POINT('Ctrl Pts',(-5.75643035625,57.2656249993855,3.32347661575227));
#5327=CARTESIAN_POINT('Ctrl Pts',(-2.878215178125,57.3031249993855,4.9852149236284));
#5328=CARTESIAN_POINT('Ctrl Pts',(-1.22102549985663E-15,57.3406249993855,
6.64695323150454));
#5329=CARTESIAN_POINT('Ctrl Pts',(2.878215178125,57.3781249993855,4.98521492362841));
#5330=CARTESIAN_POINT('Ctrl Pts',(5.75643035625,57.4156249993855,3.32347661575227));
#5331=CARTESIAN_POINT('Ctrl Pts',(5.75643035625,57.4531249993855,0.));
#5332=CARTESIAN_POINT('Ctrl Pts',(5.75643035625,57.4906249993855,-3.32347661575227));
#5333=CARTESIAN_POINT('Ctrl Pts',(2.878215178125,57.5281249993855,-4.9852149236284));
#5334=CARTESIAN_POINT('Ctrl Pts',(4.0700849995221E-16,57.5656249993855,
-6.64695323150454));
#5335=CARTESIAN_POINT('Ctrl Pts',(-2.878215178125,57.6031249993855,-4.9852149236284));
#5336=CARTESIAN_POINT('Ctrl Pts',(-5.75643035625,57.6406249993855,-3.32347661575227));
#5337=CARTESIAN_POINT('Ctrl Pts',(-5.75643035625,57.6781249993855,-7.04959401029622E-16));
#5338=CARTESIAN_POINT('Origin',(-2.22044604925031E-15,50.1968749993855,
-2.77555756156289E-16));
#5339=CARTESIAN_POINT('',(-5.75643035625,56.6656249993855,-9.82515157185911E-16));
#5340=CARTESIAN_POINT('',(-5.75643035625,56.7781249993855,-9.82515157185911E-16));
#5341=CARTESIAN_POINT('',(-5.75643035625,50.1968749993855,-1.2600709133422E-15));
#5342=CARTESIAN_POINT('Ctrl Pts',(-5.75643035625,56.6656249993855,-7.04959401029622E-16));
#5343=CARTESIAN_POINT('Ctrl Pts',(-5.75643035625,56.7031249993855,3.32347661575227));
#5344=CARTESIAN_POINT('Ctrl Pts',(-2.878215178125,56.7406249993855,4.9852149236284));
#5345=CARTESIAN_POINT('Ctrl Pts',(-1.22102549985663E-15,56.7781249993855,
6.64695323150454));
#5346=CARTESIAN_POINT('Ctrl Pts',(2.878215178125,56.8156249993855,4.98521492362841));
#5347=CARTESIAN_POINT('Ctrl Pts',(5.75643035625,56.8531249993855,3.32347661575227));
#5348=CARTESIAN_POINT('Ctrl Pts',(5.75643035625,56.8906249993855,0.));
#5349=CARTESIAN_POINT('Ctrl Pts',(5.75643035625,56.9281249993855,-3.32347661575227));
#5350=CARTESIAN_POINT('Ctrl Pts',(2.878215178125,56.9656249993855,-4.9852149236284));
#5351=CARTESIAN_POINT('Ctrl Pts',(4.0700849995221E-16,57.0031249993855,
-6.64695323150454));
#5352=CARTESIAN_POINT('Ctrl Pts',(-2.878215178125,57.0406249993855,-4.9852149236284));
#5353=CARTESIAN_POINT('Ctrl Pts',(-5.75643035625,57.0781249993855,-3.32347661575227));
#5354=CARTESIAN_POINT('Ctrl Pts',(-5.75643035625,57.1156249993855,-7.04959401029622E-16));
#5355=CARTESIAN_POINT('Ctrl Pts',(-5.75643035625,56.7781249993855,-7.04959401029622E-16));
#5356=CARTESIAN_POINT('Ctrl Pts',(-5.75643035625,56.8156249993855,3.32347661575227));
#5357=CARTESIAN_POINT('Ctrl Pts',(-2.878215178125,56.8531249993855,4.9852149236284));
#5358=CARTESIAN_POINT('Ctrl Pts',(-1.22102549985663E-15,56.8906249993855,
6.64695323150454));
#5359=CARTESIAN_POINT('Ctrl Pts',(2.878215178125,56.9281249993855,4.98521492362841));
#5360=CARTESIAN_POINT('Ctrl Pts',(5.75643035625,56.9656249993855,3.32347661575227));
#5361=CARTESIAN_POINT('Ctrl Pts',(5.75643035625,57.0031249993855,0.));
#5362=CARTESIAN_POINT('Ctrl Pts',(5.75643035625,57.0406249993855,-3.32347661575227));
#5363=CARTESIAN_POINT('Ctrl Pts',(2.878215178125,57.0781249993855,-4.9852149236284));
#5364=CARTESIAN_POINT('Ctrl Pts',(4.0700849995221E-16,57.1156249993855,
-6.64695323150454));
#5365=CARTESIAN_POINT('Ctrl Pts',(-2.878215178125,57.1531249993855,-4.9852149236284));
#5366=CARTESIAN_POINT('Ctrl Pts',(-5.75643035625,57.1906249993855,-3.32347661575227));
#5367=CARTESIAN_POINT('Ctrl Pts',(-5.75643035625,57.2281249993855,-7.04959401029622E-16));
#5368=CARTESIAN_POINT('Origin',(-2.22044604925031E-15,50.1968749993855,
-2.77555756156289E-16));
#5369=CARTESIAN_POINT('',(-5.75643035625,56.2156249993855,-9.82515157185911E-16));
#5370=CARTESIAN_POINT('',(-5.75643035625,56.3281249993855,-9.82515157185911E-16));
#5371=CARTESIAN_POINT('',(-5.75643035625,50.1968749993855,-1.2600709133422E-15));
#5372=CARTESIAN_POINT('Ctrl Pts',(-5.75643035625,56.2156249993855,-7.04959401029622E-16));
#5373=CARTESIAN_POINT('Ctrl Pts',(-5.75643035625,56.2531249993855,3.32347661575227));
#5374=CARTESIAN_POINT('Ctrl Pts',(-2.878215178125,56.2906249993855,4.9852149236284));
#5375=CARTESIAN_POINT('Ctrl Pts',(-1.22102549985663E-15,56.3281249993855,
6.64695323150454));
#5376=CARTESIAN_POINT('Ctrl Pts',(2.878215178125,56.3656249993855,4.98521492362841));
#5377=CARTESIAN_POINT('Ctrl Pts',(5.75643035625,56.4031249993855,3.32347661575227));
#5378=CARTESIAN_POINT('Ctrl Pts',(5.75643035625,56.4406249993855,0.));
#5379=CARTESIAN_POINT('Ctrl Pts',(5.75643035625,56.4781249993855,-3.32347661575227));
#5380=CARTESIAN_POINT('Ctrl Pts',(2.878215178125,56.5156249993855,-4.9852149236284));
#5381=CARTESIAN_POINT('Ctrl Pts',(4.0700849995221E-16,56.5531249993855,
-6.64695323150454));
#5382=CARTESIAN_POINT('Ctrl Pts',(-2.878215178125,56.5906249993855,-4.9852149236284));
#5383=CARTESIAN_POINT('Ctrl Pts',(-5.75643035625,56.6281249993855,-3.32347661575227));
#5384=CARTESIAN_POINT('Ctrl Pts',(-5.75643035625,56.6656249993855,-7.04959401029622E-16));
#5385=CARTESIAN_POINT('Ctrl Pts',(-5.75643035625,56.3281249993855,-7.04959401029622E-16));
#5386=CARTESIAN_POINT('Ctrl Pts',(-5.75643035625,56.3656249993855,3.32347661575227));
#5387=CARTESIAN_POINT('Ctrl Pts',(-2.878215178125,56.4031249993855,4.9852149236284));
#5388=CARTESIAN_POINT('Ctrl Pts',(-1.22102549985663E-15,56.4406249993855,
6.64695323150454));
#5389=CARTESIAN_POINT('Ctrl Pts',(2.878215178125,56.4781249993855,4.98521492362841));
#5390=CARTESIAN_POINT('Ctrl Pts',(5.75643035625,56.5156249993855,3.32347661575227));
#5391=CARTESIAN_POINT('Ctrl Pts',(5.75643035625,56.5531249993855,0.));
#5392=CARTESIAN_POINT('Ctrl Pts',(5.75643035625,56.5906249993855,-3.32347661575227));
#5393=CARTESIAN_POINT('Ctrl Pts',(2.878215178125,56.6281249993855,-4.9852149236284));
#5394=CARTESIAN_POINT('Ctrl Pts',(4.0700849995221E-16,56.6656249993855,
-6.64695323150454));
#5395=CARTESIAN_POINT('Ctrl Pts',(-2.878215178125,56.7031249993855,-4.9852149236284));
#5396=CARTESIAN_POINT('Ctrl Pts',(-5.75643035625,56.7406249993855,-3.32347661575227));
#5397=CARTESIAN_POINT('Ctrl Pts',(-5.75643035625,56.7781249993855,-7.04959401029622E-16));
#5398=CARTESIAN_POINT('Origin',(-2.22044604925031E-15,50.1968749993855,
-2.77555756156289E-16));
#5399=CARTESIAN_POINT('',(-5.75643035625,55.7656249993855,-9.82515157185911E-16));
#5400=CARTESIAN_POINT('',(-5.75643035625,55.8781249993855,-9.82515157185911E-16));
#5401=CARTESIAN_POINT('',(-5.75643035625,50.1968749993855,-1.2600709133422E-15));
#5402=CARTESIAN_POINT('Ctrl Pts',(-5.75643035625,55.7656249993855,-7.04959401029622E-16));
#5403=CARTESIAN_POINT('Ctrl Pts',(-5.75643035625,55.8031249993855,3.32347661575227));
#5404=CARTESIAN_POINT('Ctrl Pts',(-2.878215178125,55.8406249993855,4.9852149236284));
#5405=CARTESIAN_POINT('Ctrl Pts',(-1.22102549985663E-15,55.8781249993855,
6.64695323150454));
#5406=CARTESIAN_POINT('Ctrl Pts',(2.878215178125,55.9156249993855,4.98521492362841));
#5407=CARTESIAN_POINT('Ctrl Pts',(5.75643035625,55.9531249993855,3.32347661575227));
#5408=CARTESIAN_POINT('Ctrl Pts',(5.75643035625,55.9906249993855,0.));
#5409=CARTESIAN_POINT('Ctrl Pts',(5.75643035625,56.0281249993855,-3.32347661575227));
#5410=CARTESIAN_POINT('Ctrl Pts',(2.878215178125,56.0656249993855,-4.9852149236284));
#5411=CARTESIAN_POINT('Ctrl Pts',(4.0700849995221E-16,56.1031249993855,
-6.64695323150454));
#5412=CARTESIAN_POINT('Ctrl Pts',(-2.878215178125,56.1406249993855,-4.9852149236284));
#5413=CARTESIAN_POINT('Ctrl Pts',(-5.75643035625,56.1781249993855,-3.32347661575227));
#5414=CARTESIAN_POINT('Ctrl Pts',(-5.75643035625,56.2156249993855,-7.04959401029622E-16));
#5415=CARTESIAN_POINT('Ctrl Pts',(-5.75643035625,55.8781249993855,-7.04959401029622E-16));
#5416=CARTESIAN_POINT('Ctrl Pts',(-5.75643035625,55.9156249993855,3.32347661575227));
#5417=CARTESIAN_POINT('Ctrl Pts',(-2.878215178125,55.9531249993855,4.9852149236284));
#5418=CARTESIAN_POINT('Ctrl Pts',(-1.22102549985663E-15,55.9906249993855,
6.64695323150454));
#5419=CARTESIAN_POINT('Ctrl Pts',(2.878215178125,56.0281249993855,4.98521492362841));
#5420=CARTESIAN_POINT('Ctrl Pts',(5.75643035625,56.0656249993855,3.32347661575227));
#5421=CARTESIAN_POINT('Ctrl Pts',(5.75643035625,56.1031249993855,0.));
#5422=CARTESIAN_POINT('Ctrl Pts',(5.75643035625,56.1406249993855,-3.32347661575227));
#5423=CARTESIAN_POINT('Ctrl Pts',(2.878215178125,56.1781249993855,-4.9852149236284));
#5424=CARTESIAN_POINT('Ctrl Pts',(4.0700849995221E-16,56.2156249993855,
-6.64695323150454));
#5425=CARTESIAN_POINT('Ctrl Pts',(-2.878215178125,56.2531249993855,-4.9852149236284));
#5426=CARTESIAN_POINT('Ctrl Pts',(-5.75643035625,56.2906249993855,-3.32347661575227));
#5427=CARTESIAN_POINT('Ctrl Pts',(-5.75643035625,56.3281249993855,-7.04959401029622E-16));
#5428=CARTESIAN_POINT('Origin',(-2.22044604925031E-15,50.1968749993855,
-2.77555756156289E-16));
#5429=CARTESIAN_POINT('',(-5.75643035625,55.3156249993855,-9.82515157185911E-16));
#5430=CARTESIAN_POINT('',(-5.75643035625,55.4281249993855,-9.82515157185911E-16));
#5431=CARTESIAN_POINT('',(-5.75643035625,50.1968749993855,-1.2600709133422E-15));
#5432=CARTESIAN_POINT('Ctrl Pts',(-5.75643035625,55.3156249993855,-7.04959401029622E-16));
#5433=CARTESIAN_POINT('Ctrl Pts',(-5.75643035625,55.3531249993855,3.32347661575227));
#5434=CARTESIAN_POINT('Ctrl Pts',(-2.878215178125,55.3906249993855,4.9852149236284));
#5435=CARTESIAN_POINT('Ctrl Pts',(-1.22102549985663E-15,55.4281249993855,
6.64695323150454));
#5436=CARTESIAN_POINT('Ctrl Pts',(2.878215178125,55.4656249993855,4.98521492362841));
#5437=CARTESIAN_POINT('Ctrl Pts',(5.75643035625,55.5031249993855,3.32347661575227));
#5438=CARTESIAN_POINT('Ctrl Pts',(5.75643035625,55.5406249993855,0.));
#5439=CARTESIAN_POINT('Ctrl Pts',(5.75643035625,55.5781249993855,-3.32347661575227));
#5440=CARTESIAN_POINT('Ctrl Pts',(2.878215178125,55.6156249993855,-4.9852149236284));
#5441=CARTESIAN_POINT('Ctrl Pts',(4.0700849995221E-16,55.6531249993855,
-6.64695323150454));
#5442=CARTESIAN_POINT('Ctrl Pts',(-2.878215178125,55.6906249993855,-4.9852149236284));
#5443=CARTESIAN_POINT('Ctrl Pts',(-5.75643035625,55.7281249993855,-3.32347661575227));
#5444=CARTESIAN_POINT('Ctrl Pts',(-5.75643035625,55.7656249993855,-7.04959401029622E-16));
#5445=CARTESIAN_POINT('Ctrl Pts',(-5.75643035625,55.4281249993855,-7.04959401029622E-16));
#5446=CARTESIAN_POINT('Ctrl Pts',(-5.75643035625,55.4656249993855,3.32347661575227));
#5447=CARTESIAN_POINT('Ctrl Pts',(-2.878215178125,55.5031249993855,4.9852149236284));
#5448=CARTESIAN_POINT('Ctrl Pts',(-1.22102549985663E-15,55.5406249993855,
6.64695323150454));
#5449=CARTESIAN_POINT('Ctrl Pts',(2.878215178125,55.5781249993855,4.98521492362841));
#5450=CARTESIAN_POINT('Ctrl Pts',(5.75643035625,55.6156249993855,3.32347661575227));
#5451=CARTESIAN_POINT('Ctrl Pts',(5.75643035625,55.6531249993855,0.));
#5452=CARTESIAN_POINT('Ctrl Pts',(5.75643035625,55.6906249993855,-3.32347661575227));
#5453=CARTESIAN_POINT('Ctrl Pts',(2.878215178125,55.7281249993855,-4.9852149236284));
#5454=CARTESIAN_POINT('Ctrl Pts',(4.0700849995221E-16,55.7656249993855,
-6.64695323150454));
#5455=CARTESIAN_POINT('Ctrl Pts',(-2.878215178125,55.8031249993855,-4.9852149236284));
#5456=CARTESIAN_POINT('Ctrl Pts',(-5.75643035625,55.8406249993855,-3.32347661575227));
#5457=CARTESIAN_POINT('Ctrl Pts',(-5.75643035625,55.8781249993855,-7.04959401029622E-16));
#5458=CARTESIAN_POINT('Origin',(-2.22044604925031E-15,50.1968749993855,
-2.77555756156289E-16));
#5459=CARTESIAN_POINT('',(-5.75643035625,54.8656249993855,-9.82515157185911E-16));
#5460=CARTESIAN_POINT('',(-5.75643035625,54.9781249993855,-9.82515157185911E-16));
#5461=CARTESIAN_POINT('',(-5.75643035625,50.1968749993855,-1.2600709133422E-15));
#5462=CARTESIAN_POINT('Ctrl Pts',(-5.75643035625,54.8656249993855,-7.04959401029622E-16));
#5463=CARTESIAN_POINT('Ctrl Pts',(-5.75643035625,54.9031249993855,3.32347661575227));
#5464=CARTESIAN_POINT('Ctrl Pts',(-2.878215178125,54.9406249993855,4.9852149236284));
#5465=CARTESIAN_POINT('Ctrl Pts',(-1.22102549985663E-15,54.9781249993855,
6.64695323150454));
#5466=CARTESIAN_POINT('Ctrl Pts',(2.878215178125,55.0156249993855,4.98521492362841));
#5467=CARTESIAN_POINT('Ctrl Pts',(5.75643035625,55.0531249993855,3.32347661575227));
#5468=CARTESIAN_POINT('Ctrl Pts',(5.75643035625,55.0906249993855,0.));
#5469=CARTESIAN_POINT('Ctrl Pts',(5.75643035625,55.1281249993855,-3.32347661575227));
#5470=CARTESIAN_POINT('Ctrl Pts',(2.878215178125,55.1656249993855,-4.9852149236284));
#5471=CARTESIAN_POINT('Ctrl Pts',(4.0700849995221E-16,55.2031249993855,
-6.64695323150454));
#5472=CARTESIAN_POINT('Ctrl Pts',(-2.878215178125,55.2406249993855,-4.9852149236284));
#5473=CARTESIAN_POINT('Ctrl Pts',(-5.75643035625,55.2781249993855,-3.32347661575227));
#5474=CARTESIAN_POINT('Ctrl Pts',(-5.75643035625,55.3156249993855,-7.04959401029622E-16));
#5475=CARTESIAN_POINT('Ctrl Pts',(-5.75643035625,54.9781249993855,-7.04959401029622E-16));
#5476=CARTESIAN_POINT('Ctrl Pts',(-5.75643035625,55.0156249993855,3.32347661575227));
#5477=CARTESIAN_POINT('Ctrl Pts',(-2.878215178125,55.0531249993855,4.9852149236284));
#5478=CARTESIAN_POINT('Ctrl Pts',(-1.22102549985663E-15,55.0906249993855,
6.64695323150454));
#5479=CARTESIAN_POINT('Ctrl Pts',(2.878215178125,55.1281249993855,4.98521492362841));
#5480=CARTESIAN_POINT('Ctrl Pts',(5.75643035625,55.1656249993855,3.32347661575227));
#5481=CARTESIAN_POINT('Ctrl Pts',(5.75643035625,55.2031249993855,0.));
#5482=CARTESIAN_POINT('Ctrl Pts',(5.75643035625,55.2406249993855,-3.32347661575227));
#5483=CARTESIAN_POINT('Ctrl Pts',(2.878215178125,55.2781249993855,-4.9852149236284));
#5484=CARTESIAN_POINT('Ctrl Pts',(4.0700849995221E-16,55.3156249993855,
-6.64695323150454));
#5485=CARTESIAN_POINT('Ctrl Pts',(-2.878215178125,55.3531249993855,-4.9852149236284));
#5486=CARTESIAN_POINT('Ctrl Pts',(-5.75643035625,55.3906249993855,-3.32347661575227));
#5487=CARTESIAN_POINT('Ctrl Pts',(-5.75643035625,55.4281249993855,-7.04959401029622E-16));
#5488=CARTESIAN_POINT('Origin',(-2.22044604925031E-15,50.1968749993855,
-2.77555756156289E-16));
#5489=CARTESIAN_POINT('',(-5.75643035625,54.4156249993855,-9.82515157185911E-16));
#5490=CARTESIAN_POINT('',(-5.75643035625,54.5281249993855,-9.82515157185911E-16));
#5491=CARTESIAN_POINT('',(-5.75643035625,50.1968749993855,-1.2600709133422E-15));
#5492=CARTESIAN_POINT('Ctrl Pts',(-5.75643035625,54.4156249993855,-7.04959401029622E-16));
#5493=CARTESIAN_POINT('Ctrl Pts',(-5.75643035625,54.4531249993855,3.32347661575227));
#5494=CARTESIAN_POINT('Ctrl Pts',(-2.878215178125,54.4906249993855,4.9852149236284));
#5495=CARTESIAN_POINT('Ctrl Pts',(-1.22102549985663E-15,54.5281249993855,
6.64695323150454));
#5496=CARTESIAN_POINT('Ctrl Pts',(2.878215178125,54.5656249993855,4.98521492362841));
#5497=CARTESIAN_POINT('Ctrl Pts',(5.75643035625,54.6031249993855,3.32347661575227));
#5498=CARTESIAN_POINT('Ctrl Pts',(5.75643035625,54.6406249993855,0.));
#5499=CARTESIAN_POINT('Ctrl Pts',(5.75643035625,54.6781249993855,-3.32347661575227));
#5500=CARTESIAN_POINT('Ctrl Pts',(2.878215178125,54.7156249993855,-4.9852149236284));
#5501=CARTESIAN_POINT('Ctrl Pts',(4.0700849995221E-16,54.7531249993855,
-6.64695323150454));
#5502=CARTESIAN_POINT('Ctrl Pts',(-2.878215178125,54.7906249993855,-4.9852149236284));
#5503=CARTESIAN_POINT('Ctrl Pts',(-5.75643035625,54.8281249993855,-3.32347661575227));
#5504=CARTESIAN_POINT('Ctrl Pts',(-5.75643035625,54.8656249993855,-7.04959401029622E-16));
#5505=CARTESIAN_POINT('Ctrl Pts',(-5.75643035625,54.5281249993855,-7.04959401029622E-16));
#5506=CARTESIAN_POINT('Ctrl Pts',(-5.75643035625,54.5656249993855,3.32347661575227));
#5507=CARTESIAN_POINT('Ctrl Pts',(-2.878215178125,54.6031249993855,4.9852149236284));
#5508=CARTESIAN_POINT('Ctrl Pts',(-1.22102549985663E-15,54.6406249993855,
6.64695323150454));
#5509=CARTESIAN_POINT('Ctrl Pts',(2.878215178125,54.6781249993855,4.98521492362841));
#5510=CARTESIAN_POINT('Ctrl Pts',(5.75643035625,54.7156249993855,3.32347661575227));
#5511=CARTESIAN_POINT('Ctrl Pts',(5.75643035625,54.7531249993855,0.));
#5512=CARTESIAN_POINT('Ctrl Pts',(5.75643035625,54.7906249993855,-3.32347661575227));
#5513=CARTESIAN_POINT('Ctrl Pts',(2.878215178125,54.8281249993855,-4.9852149236284));
#5514=CARTESIAN_POINT('Ctrl Pts',(4.0700849995221E-16,54.8656249993855,
-6.64695323150454));
#5515=CARTESIAN_POINT('Ctrl Pts',(-2.878215178125,54.9031249993855,-4.9852149236284));
#5516=CARTESIAN_POINT('Ctrl Pts',(-5.75643035625,54.9406249993855,-3.32347661575227));
#5517=CARTESIAN_POINT('Ctrl Pts',(-5.75643035625,54.9781249993855,-7.04959401029622E-16));
#5518=CARTESIAN_POINT('Origin',(-2.22044604925031E-15,50.1968749993855,
-2.77555756156289E-16));
#5519=CARTESIAN_POINT('',(-5.75643035625,53.9656249993855,-9.82515157185911E-16));
#5520=CARTESIAN_POINT('',(-5.75643035625,54.0781249993855,-9.82515157185911E-16));
#5521=CARTESIAN_POINT('',(-5.75643035625,50.1968749993855,-1.2600709133422E-15));
#5522=CARTESIAN_POINT('Ctrl Pts',(-5.75643035625,53.9656249993855,-7.04959401029622E-16));
#5523=CARTESIAN_POINT('Ctrl Pts',(-5.75643035625,54.0031249993855,3.32347661575227));
#5524=CARTESIAN_POINT('Ctrl Pts',(-2.878215178125,54.0406249993855,4.9852149236284));
#5525=CARTESIAN_POINT('Ctrl Pts',(-1.22102549985663E-15,54.0781249993855,
6.64695323150454));
#5526=CARTESIAN_POINT('Ctrl Pts',(2.878215178125,54.1156249993855,4.98521492362841));
#5527=CARTESIAN_POINT('Ctrl Pts',(5.75643035625,54.1531249993855,3.32347661575227));
#5528=CARTESIAN_POINT('Ctrl Pts',(5.75643035625,54.1906249993855,0.));
#5529=CARTESIAN_POINT('Ctrl Pts',(5.75643035625,54.2281249993855,-3.32347661575227));
#5530=CARTESIAN_POINT('Ctrl Pts',(2.878215178125,54.2656249993855,-4.9852149236284));
#5531=CARTESIAN_POINT('Ctrl Pts',(4.0700849995221E-16,54.3031249993855,
-6.64695323150454));
#5532=CARTESIAN_POINT('Ctrl Pts',(-2.878215178125,54.3406249993855,-4.9852149236284));
#5533=CARTESIAN_POINT('Ctrl Pts',(-5.75643035625,54.3781249993855,-3.32347661575227));
#5534=CARTESIAN_POINT('Ctrl Pts',(-5.75643035625,54.4156249993855,-7.04959401029622E-16));
#5535=CARTESIAN_POINT('Ctrl Pts',(-5.75643035625,54.0781249993855,-7.04959401029622E-16));
#5536=CARTESIAN_POINT('Ctrl Pts',(-5.75643035625,54.1156249993855,3.32347661575227));
#5537=CARTESIAN_POINT('Ctrl Pts',(-2.878215178125,54.1531249993855,4.9852149236284));
#5538=CARTESIAN_POINT('Ctrl Pts',(-1.22102549985663E-15,54.1906249993855,
6.64695323150454));
#5539=CARTESIAN_POINT('Ctrl Pts',(2.878215178125,54.2281249993855,4.98521492362841));
#5540=CARTESIAN_POINT('Ctrl Pts',(5.75643035625,54.2656249993855,3.32347661575227));
#5541=CARTESIAN_POINT('Ctrl Pts',(5.75643035625,54.3031249993855,0.));
#5542=CARTESIAN_POINT('Ctrl Pts',(5.75643035625,54.3406249993855,-3.32347661575227));
#5543=CARTESIAN_POINT('Ctrl Pts',(2.878215178125,54.3781249993855,-4.9852149236284));
#5544=CARTESIAN_POINT('Ctrl Pts',(4.0700849995221E-16,54.4156249993855,
-6.64695323150454));
#5545=CARTESIAN_POINT('Ctrl Pts',(-2.878215178125,54.4531249993855,-4.9852149236284));
#5546=CARTESIAN_POINT('Ctrl Pts',(-5.75643035625,54.4906249993855,-3.32347661575227));
#5547=CARTESIAN_POINT('Ctrl Pts',(-5.75643035625,54.5281249993855,-7.04959401029622E-16));
#5548=CARTESIAN_POINT('Origin',(-2.22044604925031E-15,50.1968749993855,
-2.77555756156289E-16));
#5549=CARTESIAN_POINT('',(-5.75643035625,53.5156249993855,-9.82515157185911E-16));
#5550=CARTESIAN_POINT('',(-5.75643035625,53.6281249993855,-9.82515157185911E-16));
#5551=CARTESIAN_POINT('',(-5.75643035625,50.1968749993855,-1.2600709133422E-15));
#5552=CARTESIAN_POINT('Ctrl Pts',(-5.75643035625,53.5156249993855,-7.04959401029622E-16));
#5553=CARTESIAN_POINT('Ctrl Pts',(-5.75643035625,53.5531249993855,3.32347661575227));
#5554=CARTESIAN_POINT('Ctrl Pts',(-2.878215178125,53.5906249993855,4.9852149236284));
#5555=CARTESIAN_POINT('Ctrl Pts',(-1.22102549985663E-15,53.6281249993855,
6.64695323150454));
#5556=CARTESIAN_POINT('Ctrl Pts',(2.878215178125,53.6656249993855,4.98521492362841));
#5557=CARTESIAN_POINT('Ctrl Pts',(5.75643035625,53.7031249993855,3.32347661575227));
#5558=CARTESIAN_POINT('Ctrl Pts',(5.75643035625,53.7406249993855,0.));
#5559=CARTESIAN_POINT('Ctrl Pts',(5.75643035625,53.7781249993855,-3.32347661575227));
#5560=CARTESIAN_POINT('Ctrl Pts',(2.878215178125,53.8156249993855,-4.9852149236284));
#5561=CARTESIAN_POINT('Ctrl Pts',(4.0700849995221E-16,53.8531249993855,
-6.64695323150454));
#5562=CARTESIAN_POINT('Ctrl Pts',(-2.878215178125,53.8906249993855,-4.9852149236284));
#5563=CARTESIAN_POINT('Ctrl Pts',(-5.75643035625,53.9281249993855,-3.32347661575227));
#5564=CARTESIAN_POINT('Ctrl Pts',(-5.75643035625,53.9656249993855,-7.04959401029622E-16));
#5565=CARTESIAN_POINT('Ctrl Pts',(-5.75643035625,53.6281249993855,-7.04959401029622E-16));
#5566=CARTESIAN_POINT('Ctrl Pts',(-5.75643035625,53.6656249993855,3.32347661575227));
#5567=CARTESIAN_POINT('Ctrl Pts',(-2.878215178125,53.7031249993855,4.9852149236284));
#5568=CARTESIAN_POINT('Ctrl Pts',(-1.22102549985663E-15,53.7406249993855,
6.64695323150454));
#5569=CARTESIAN_POINT('Ctrl Pts',(2.878215178125,53.7781249993855,4.98521492362841));
#5570=CARTESIAN_POINT('Ctrl Pts',(5.75643035625,53.8156249993855,3.32347661575227));
#5571=CARTESIAN_POINT('Ctrl Pts',(5.75643035625,53.8531249993855,0.));
#5572=CARTESIAN_POINT('Ctrl Pts',(5.75643035625,53.8906249993855,-3.32347661575227));
#5573=CARTESIAN_POINT('Ctrl Pts',(2.878215178125,53.9281249993855,-4.9852149236284));
#5574=CARTESIAN_POINT('Ctrl Pts',(4.0700849995221E-16,53.9656249993855,
-6.64695323150454));
#5575=CARTESIAN_POINT('Ctrl Pts',(-2.878215178125,54.0031249993855,-4.9852149236284));
#5576=CARTESIAN_POINT('Ctrl Pts',(-5.75643035625,54.0406249993855,-3.32347661575227));
#5577=CARTESIAN_POINT('Ctrl Pts',(-5.75643035625,54.0781249993855,-7.04959401029622E-16));
#5578=CARTESIAN_POINT('Origin',(-2.22044604925031E-15,50.1968749993855,
-2.77555756156289E-16));
#5579=CARTESIAN_POINT('',(-5.75643035625,53.0656249993855,-9.82515157185911E-16));
#5580=CARTESIAN_POINT('',(-5.75643035625,53.1781249993855,-9.82515157185911E-16));
#5581=CARTESIAN_POINT('',(-5.75643035625,50.1968749993855,-1.2600709133422E-15));
#5582=CARTESIAN_POINT('Ctrl Pts',(-5.75643035625,53.0656249993855,-7.04959401029622E-16));
#5583=CARTESIAN_POINT('Ctrl Pts',(-5.75643035625,53.1031249993855,3.32347661575227));
#5584=CARTESIAN_POINT('Ctrl Pts',(-2.878215178125,53.1406249993855,4.9852149236284));
#5585=CARTESIAN_POINT('Ctrl Pts',(-1.22102549985663E-15,53.1781249993855,
6.64695323150454));
#5586=CARTESIAN_POINT('Ctrl Pts',(2.878215178125,53.2156249993855,4.98521492362841));
#5587=CARTESIAN_POINT('Ctrl Pts',(5.75643035625,53.2531249993855,3.32347661575227));
#5588=CARTESIAN_POINT('Ctrl Pts',(5.75643035625,53.2906249993855,0.));
#5589=CARTESIAN_POINT('Ctrl Pts',(5.75643035625,53.3281249993855,-3.32347661575227));
#5590=CARTESIAN_POINT('Ctrl Pts',(2.878215178125,53.3656249993855,-4.9852149236284));
#5591=CARTESIAN_POINT('Ctrl Pts',(4.0700849995221E-16,53.4031249993855,
-6.64695323150454));
#5592=CARTESIAN_POINT('Ctrl Pts',(-2.878215178125,53.4406249993855,-4.9852149236284));
#5593=CARTESIAN_POINT('Ctrl Pts',(-5.75643035625,53.4781249993855,-3.32347661575227));
#5594=CARTESIAN_POINT('Ctrl Pts',(-5.75643035625,53.5156249993855,-7.04959401029622E-16));
#5595=CARTESIAN_POINT('Ctrl Pts',(-5.75643035625,53.1781249993855,-7.04959401029622E-16));
#5596=CARTESIAN_POINT('Ctrl Pts',(-5.75643035625,53.2156249993855,3.32347661575227));
#5597=CARTESIAN_POINT('Ctrl Pts',(-2.878215178125,53.2531249993855,4.9852149236284));
#5598=CARTESIAN_POINT('Ctrl Pts',(-1.22102549985663E-15,53.2906249993855,
6.64695323150454));
#5599=CARTESIAN_POINT('Ctrl Pts',(2.878215178125,53.3281249993855,4.98521492362841));
#5600=CARTESIAN_POINT('Ctrl Pts',(5.75643035625,53.3656249993855,3.32347661575227));
#5601=CARTESIAN_POINT('Ctrl Pts',(5.75643035625,53.4031249993855,0.));
#5602=CARTESIAN_POINT('Ctrl Pts',(5.75643035625,53.4406249993855,-3.32347661575227));
#5603=CARTESIAN_POINT('Ctrl Pts',(2.878215178125,53.4781249993855,-4.9852149236284));
#5604=CARTESIAN_POINT('Ctrl Pts',(4.0700849995221E-16,53.5156249993855,
-6.64695323150454));
#5605=CARTESIAN_POINT('Ctrl Pts',(-2.878215178125,53.5531249993855,-4.9852149236284));
#5606=CARTESIAN_POINT('Ctrl Pts',(-5.75643035625,53.5906249993855,-3.32347661575227));
#5607=CARTESIAN_POINT('Ctrl Pts',(-5.75643035625,53.6281249993855,-7.04959401029622E-16));
#5608=CARTESIAN_POINT('Origin',(-2.22044604925031E-15,50.1968749993855,
-2.77555756156289E-16));
#5609=CARTESIAN_POINT('',(-5.75643035625,52.6156249993855,-9.82515157185911E-16));
#5610=CARTESIAN_POINT('',(-5.75643035625,52.7281249993855,-9.82515157185911E-16));
#5611=CARTESIAN_POINT('',(-5.75643035625,50.1968749993855,-1.2600709133422E-15));
#5612=CARTESIAN_POINT('Ctrl Pts',(-5.75643035625,52.6156249993855,-7.04959401029622E-16));
#5613=CARTESIAN_POINT('Ctrl Pts',(-5.75643035625,52.6531249993855,3.32347661575227));
#5614=CARTESIAN_POINT('Ctrl Pts',(-2.878215178125,52.6906249993855,4.9852149236284));
#5615=CARTESIAN_POINT('Ctrl Pts',(-1.22102549985663E-15,52.7281249993855,
6.64695323150454));
#5616=CARTESIAN_POINT('Ctrl Pts',(2.878215178125,52.7656249993855,4.98521492362841));
#5617=CARTESIAN_POINT('Ctrl Pts',(5.75643035625,52.8031249993855,3.32347661575227));
#5618=CARTESIAN_POINT('Ctrl Pts',(5.75643035625,52.8406249993855,0.));
#5619=CARTESIAN_POINT('Ctrl Pts',(5.75643035625,52.8781249993855,-3.32347661575227));
#5620=CARTESIAN_POINT('Ctrl Pts',(2.878215178125,52.9156249993855,-4.9852149236284));
#5621=CARTESIAN_POINT('Ctrl Pts',(4.0700849995221E-16,52.9531249993855,
-6.64695323150454));
#5622=CARTESIAN_POINT('Ctrl Pts',(-2.878215178125,52.9906249993855,-4.9852149236284));
#5623=CARTESIAN_POINT('Ctrl Pts',(-5.75643035625,53.0281249993855,-3.32347661575227));
#5624=CARTESIAN_POINT('Ctrl Pts',(-5.75643035625,53.0656249993855,-7.04959401029622E-16));
#5625=CARTESIAN_POINT('Ctrl Pts',(-5.75643035625,52.7281249993855,-7.04959401029622E-16));
#5626=CARTESIAN_POINT('Ctrl Pts',(-5.75643035625,52.7656249993855,3.32347661575227));
#5627=CARTESIAN_POINT('Ctrl Pts',(-2.878215178125,52.8031249993855,4.9852149236284));
#5628=CARTESIAN_POINT('Ctrl Pts',(-1.22102549985663E-15,52.8406249993855,
6.64695323150454));
#5629=CARTESIAN_POINT('Ctrl Pts',(2.878215178125,52.8781249993855,4.98521492362841));
#5630=CARTESIAN_POINT('Ctrl Pts',(5.75643035625,52.9156249993855,3.32347661575227));
#5631=CARTESIAN_POINT('Ctrl Pts',(5.75643035625,52.9531249993855,0.));
#5632=CARTESIAN_POINT('Ctrl Pts',(5.75643035625,52.9906249993855,-3.32347661575227));
#5633=CARTESIAN_POINT('Ctrl Pts',(2.878215178125,53.0281249993855,-4.9852149236284));
#5634=CARTESIAN_POINT('Ctrl Pts',(4.0700849995221E-16,53.0656249993855,
-6.64695323150454));
#5635=CARTESIAN_POINT('Ctrl Pts',(-2.878215178125,53.1031249993855,-4.9852149236284));
#5636=CARTESIAN_POINT('Ctrl Pts',(-5.75643035625,53.1406249993855,-3.32347661575227));
#5637=CARTESIAN_POINT('Ctrl Pts',(-5.75643035625,53.1781249993855,-7.04959401029622E-16));
#5638=CARTESIAN_POINT('Origin',(-2.22044604925031E-15,50.1968749993855,
-2.77555756156289E-16));
#5639=CARTESIAN_POINT('',(-5.75643035625,52.1656249993855,-9.82515157185911E-16));
#5640=CARTESIAN_POINT('',(-5.75643035625,52.2781249993855,-9.82515157185911E-16));
#5641=CARTESIAN_POINT('',(-5.75643035625,50.1968749993855,-1.2600709133422E-15));
#5642=CARTESIAN_POINT('Ctrl Pts',(-5.75643035625,52.1656249993855,-7.04959401029622E-16));
#5643=CARTESIAN_POINT('Ctrl Pts',(-5.75643035625,52.2031249993855,3.32347661575227));
#5644=CARTESIAN_POINT('Ctrl Pts',(-2.878215178125,52.2406249993855,4.9852149236284));
#5645=CARTESIAN_POINT('Ctrl Pts',(-1.22102549985663E-15,52.2781249993855,
6.64695323150454));
#5646=CARTESIAN_POINT('Ctrl Pts',(2.878215178125,52.3156249993855,4.98521492362841));
#5647=CARTESIAN_POINT('Ctrl Pts',(5.75643035625,52.3531249993855,3.32347661575227));
#5648=CARTESIAN_POINT('Ctrl Pts',(5.75643035625,52.3906249993855,0.));
#5649=CARTESIAN_POINT('Ctrl Pts',(5.75643035625,52.4281249993855,-3.32347661575227));
#5650=CARTESIAN_POINT('Ctrl Pts',(2.878215178125,52.4656249993855,-4.9852149236284));
#5651=CARTESIAN_POINT('Ctrl Pts',(4.0700849995221E-16,52.5031249993855,
-6.64695323150454));
#5652=CARTESIAN_POINT('Ctrl Pts',(-2.878215178125,52.5406249993855,-4.9852149236284));
#5653=CARTESIAN_POINT('Ctrl Pts',(-5.75643035625,52.5781249993855,-3.32347661575227));
#5654=CARTESIAN_POINT('Ctrl Pts',(-5.75643035625,52.6156249993855,-7.04959401029622E-16));
#5655=CARTESIAN_POINT('Ctrl Pts',(-5.75643035625,52.2781249993855,-7.04959401029622E-16));
#5656=CARTESIAN_POINT('Ctrl Pts',(-5.75643035625,52.3156249993855,3.32347661575227));
#5657=CARTESIAN_POINT('Ctrl Pts',(-2.878215178125,52.3531249993855,4.9852149236284));
#5658=CARTESIAN_POINT('Ctrl Pts',(-1.22102549985663E-15,52.3906249993855,
6.64695323150454));
#5659=CARTESIAN_POINT('Ctrl Pts',(2.878215178125,52.4281249993855,4.98521492362841));
#5660=CARTESIAN_POINT('Ctrl Pts',(5.75643035625,52.4656249993855,3.32347661575227));
#5661=CARTESIAN_POINT('Ctrl Pts',(5.75643035625,52.5031249993855,0.));
#5662=CARTESIAN_POINT('Ctrl Pts',(5.75643035625,52.5406249993855,-3.32347661575227));
#5663=CARTESIAN_POINT('Ctrl Pts',(2.878215178125,52.5781249993855,-4.9852149236284));
#5664=CARTESIAN_POINT('Ctrl Pts',(4.0700849995221E-16,52.6156249993855,
-6.64695323150454));
#5665=CARTESIAN_POINT('Ctrl Pts',(-2.878215178125,52.6531249993855,-4.9852149236284));
#5666=CARTESIAN_POINT('Ctrl Pts',(-5.75643035625,52.6906249993855,-3.32347661575227));
#5667=CARTESIAN_POINT('Ctrl Pts',(-5.75643035625,52.7281249993855,-7.04959401029622E-16));
#5668=CARTESIAN_POINT('Origin',(-2.22044604925031E-15,50.1968749993855,
-2.77555756156289E-16));
#5669=CARTESIAN_POINT('',(-5.75643035625,51.7156249993855,-9.82515157185911E-16));
#5670=CARTESIAN_POINT('',(-5.75643035625,51.8281249993855,-9.82515157185911E-16));
#5671=CARTESIAN_POINT('',(-5.75643035625,50.1968749993855,-1.2600709133422E-15));
#5672=CARTESIAN_POINT('Ctrl Pts',(-5.75643035625,51.7156249993855,-7.04959401029622E-16));
#5673=CARTESIAN_POINT('Ctrl Pts',(-5.75643035625,51.7531249993855,3.32347661575227));
#5674=CARTESIAN_POINT('Ctrl Pts',(-2.878215178125,51.7906249993855,4.9852149236284));
#5675=CARTESIAN_POINT('Ctrl Pts',(-1.22102549985663E-15,51.8281249993855,
6.64695323150454));
#5676=CARTESIAN_POINT('Ctrl Pts',(2.878215178125,51.8656249993855,4.98521492362841));
#5677=CARTESIAN_POINT('Ctrl Pts',(5.75643035625,51.9031249993855,3.32347661575227));
#5678=CARTESIAN_POINT('Ctrl Pts',(5.75643035625,51.9406249993855,0.));
#5679=CARTESIAN_POINT('Ctrl Pts',(5.75643035625,51.9781249993855,-3.32347661575227));
#5680=CARTESIAN_POINT('Ctrl Pts',(2.878215178125,52.0156249993855,-4.9852149236284));
#5681=CARTESIAN_POINT('Ctrl Pts',(4.0700849995221E-16,52.0531249993855,
-6.64695323150454));
#5682=CARTESIAN_POINT('Ctrl Pts',(-2.878215178125,52.0906249993855,-4.9852149236284));
#5683=CARTESIAN_POINT('Ctrl Pts',(-5.75643035625,52.1281249993855,-3.32347661575227));
#5684=CARTESIAN_POINT('Ctrl Pts',(-5.75643035625,52.1656249993855,-7.04959401029622E-16));
#5685=CARTESIAN_POINT('Ctrl Pts',(-5.75643035625,51.8281249993855,-7.04959401029622E-16));
#5686=CARTESIAN_POINT('Ctrl Pts',(-5.75643035625,51.8656249993855,3.32347661575227));
#5687=CARTESIAN_POINT('Ctrl Pts',(-2.878215178125,51.9031249993855,4.9852149236284));
#5688=CARTESIAN_POINT('Ctrl Pts',(-1.22102549985663E-15,51.9406249993855,
6.64695323150454));
#5689=CARTESIAN_POINT('Ctrl Pts',(2.878215178125,51.9781249993855,4.98521492362841));
#5690=CARTESIAN_POINT('Ctrl Pts',(5.75643035625,52.0156249993855,3.32347661575227));
#5691=CARTESIAN_POINT('Ctrl Pts',(5.75643035625,52.0531249993855,0.));
#5692=CARTESIAN_POINT('Ctrl Pts',(5.75643035625,52.0906249993855,-3.32347661575227));
#5693=CARTESIAN_POINT('Ctrl Pts',(2.878215178125,52.1281249993855,-4.9852149236284));
#5694=CARTESIAN_POINT('Ctrl Pts',(4.0700849995221E-16,52.1656249993855,
-6.64695323150454));
#5695=CARTESIAN_POINT('Ctrl Pts',(-2.878215178125,52.2031249993855,-4.9852149236284));
#5696=CARTESIAN_POINT('Ctrl Pts',(-5.75643035625,52.2406249993855,-3.32347661575227));
#5697=CARTESIAN_POINT('Ctrl Pts',(-5.75643035625,52.2781249993855,-7.04959401029622E-16));
#5698=CARTESIAN_POINT('Origin',(-2.22044604925031E-15,50.1968749993855,
-2.77555756156289E-16));
#5699=CARTESIAN_POINT('',(-5.75643035625,51.2656249993855,-9.82515157185911E-16));
#5700=CARTESIAN_POINT('',(-5.75643035625,51.3781249993855,-9.82515157185911E-16));
#5701=CARTESIAN_POINT('',(-5.75643035625,50.1968749993855,-1.2600709133422E-15));
#5702=CARTESIAN_POINT('Ctrl Pts',(-5.75643035625,51.2656249993855,-7.04959401029622E-16));
#5703=CARTESIAN_POINT('Ctrl Pts',(-5.75643035625,51.3031249993855,3.32347661575227));
#5704=CARTESIAN_POINT('Ctrl Pts',(-2.878215178125,51.3406249993855,4.9852149236284));
#5705=CARTESIAN_POINT('Ctrl Pts',(-1.22102549985663E-15,51.3781249993855,
6.64695323150454));
#5706=CARTESIAN_POINT('Ctrl Pts',(2.878215178125,51.4156249993855,4.98521492362841));
#5707=CARTESIAN_POINT('Ctrl Pts',(5.75643035625,51.4531249993855,3.32347661575227));
#5708=CARTESIAN_POINT('Ctrl Pts',(5.75643035625,51.4906249993855,0.));
#5709=CARTESIAN_POINT('Ctrl Pts',(5.75643035625,51.5281249993855,-3.32347661575227));
#5710=CARTESIAN_POINT('Ctrl Pts',(2.878215178125,51.5656249993855,-4.9852149236284));
#5711=CARTESIAN_POINT('Ctrl Pts',(4.0700849995221E-16,51.6031249993855,
-6.64695323150454));
#5712=CARTESIAN_POINT('Ctrl Pts',(-2.878215178125,51.6406249993855,-4.9852149236284));
#5713=CARTESIAN_POINT('Ctrl Pts',(-5.75643035625,51.6781249993855,-3.32347661575227));
#5714=CARTESIAN_POINT('Ctrl Pts',(-5.75643035625,51.7156249993855,-7.04959401029622E-16));
#5715=CARTESIAN_POINT('Ctrl Pts',(-5.75643035625,51.3781249993855,-7.04959401029622E-16));
#5716=CARTESIAN_POINT('Ctrl Pts',(-5.75643035625,51.4156249993855,3.32347661575227));
#5717=CARTESIAN_POINT('Ctrl Pts',(-2.878215178125,51.4531249993855,4.9852149236284));
#5718=CARTESIAN_POINT('Ctrl Pts',(-1.22102549985663E-15,51.4906249993855,
6.64695323150454));
#5719=CARTESIAN_POINT('Ctrl Pts',(2.878215178125,51.5281249993855,4.98521492362841));
#5720=CARTESIAN_POINT('Ctrl Pts',(5.75643035625,51.5656249993855,3.32347661575227));
#5721=CARTESIAN_POINT('Ctrl Pts',(5.75643035625,51.6031249993855,0.));
#5722=CARTESIAN_POINT('Ctrl Pts',(5.75643035625,51.6406249993855,-3.32347661575227));
#5723=CARTESIAN_POINT('Ctrl Pts',(2.878215178125,51.6781249993855,-4.9852149236284));
#5724=CARTESIAN_POINT('Ctrl Pts',(4.0700849995221E-16,51.7156249993855,
-6.64695323150454));
#5725=CARTESIAN_POINT('Ctrl Pts',(-2.878215178125,51.7531249993855,-4.9852149236284));
#5726=CARTESIAN_POINT('Ctrl Pts',(-5.75643035625,51.7906249993855,-3.32347661575227));
#5727=CARTESIAN_POINT('Ctrl Pts',(-5.75643035625,51.8281249993855,-7.04959401029622E-16));
#5728=CARTESIAN_POINT('Origin',(-2.22044604925031E-15,50.1968749993855,
-2.77555756156289E-16));
#5729=CARTESIAN_POINT('',(-5.75643035625,50.8156249993855,-9.82515157185911E-16));
#5730=CARTESIAN_POINT('',(-5.75643035625,50.9281249993855,-9.82515157185911E-16));
#5731=CARTESIAN_POINT('',(-5.75643035625,50.1968749993855,-1.2600709133422E-15));
#5732=CARTESIAN_POINT('Ctrl Pts',(-5.75643035625,50.8156249993855,-7.04959401029622E-16));
#5733=CARTESIAN_POINT('Ctrl Pts',(-5.75643035625,50.8531249993855,3.32347661575227));
#5734=CARTESIAN_POINT('Ctrl Pts',(-2.878215178125,50.8906249993855,4.9852149236284));
#5735=CARTESIAN_POINT('Ctrl Pts',(-1.22102549985663E-15,50.9281249993855,
6.64695323150454));
#5736=CARTESIAN_POINT('Ctrl Pts',(2.878215178125,50.9656249993855,4.98521492362841));
#5737=CARTESIAN_POINT('Ctrl Pts',(5.75643035625,51.0031249993855,3.32347661575227));
#5738=CARTESIAN_POINT('Ctrl Pts',(5.75643035625,51.0406249993855,0.));
#5739=CARTESIAN_POINT('Ctrl Pts',(5.75643035625,51.0781249993855,-3.32347661575227));
#5740=CARTESIAN_POINT('Ctrl Pts',(2.878215178125,51.1156249993855,-4.9852149236284));
#5741=CARTESIAN_POINT('Ctrl Pts',(4.0700849995221E-16,51.1531249993855,
-6.64695323150454));
#5742=CARTESIAN_POINT('Ctrl Pts',(-2.878215178125,51.1906249993855,-4.9852149236284));
#5743=CARTESIAN_POINT('Ctrl Pts',(-5.75643035625,51.2281249993855,-3.32347661575227));
#5744=CARTESIAN_POINT('Ctrl Pts',(-5.75643035625,51.2656249993855,-7.04959401029622E-16));
#5745=CARTESIAN_POINT('Ctrl Pts',(-5.75643035625,50.9281249993855,-7.04959401029622E-16));
#5746=CARTESIAN_POINT('Ctrl Pts',(-5.75643035625,50.9656249993855,3.32347661575227));
#5747=CARTESIAN_POINT('Ctrl Pts',(-2.878215178125,51.0031249993855,4.9852149236284));
#5748=CARTESIAN_POINT('Ctrl Pts',(-1.22102549985663E-15,51.0406249993855,
6.64695323150454));
#5749=CARTESIAN_POINT('Ctrl Pts',(2.878215178125,51.0781249993855,4.98521492362841));
#5750=CARTESIAN_POINT('Ctrl Pts',(5.75643035625,51.1156249993855,3.32347661575227));
#5751=CARTESIAN_POINT('Ctrl Pts',(5.75643035625,51.1531249993855,0.));
#5752=CARTESIAN_POINT('Ctrl Pts',(5.75643035625,51.1906249993855,-3.32347661575227));
#5753=CARTESIAN_POINT('Ctrl Pts',(2.878215178125,51.2281249993855,-4.9852149236284));
#5754=CARTESIAN_POINT('Ctrl Pts',(4.0700849995221E-16,51.2656249993855,
-6.64695323150454));
#5755=CARTESIAN_POINT('Ctrl Pts',(-2.878215178125,51.3031249993855,-4.9852149236284));
#5756=CARTESIAN_POINT('Ctrl Pts',(-5.75643035625,51.3406249993855,-3.32347661575227));
#5757=CARTESIAN_POINT('Ctrl Pts',(-5.75643035625,51.3781249993855,-7.04959401029622E-16));
#5758=CARTESIAN_POINT('Origin',(-2.22044604925031E-15,50.1968749993855,
-2.77555756156289E-16));
#5759=CARTESIAN_POINT('',(-5.75643035625,50.3656249993855,-9.82515157185911E-16));
#5760=CARTESIAN_POINT('',(-5.75643035625,50.4781249993855,-9.82515157185911E-16));
#5761=CARTESIAN_POINT('',(-5.75643035625,50.1968749993855,-1.2600709133422E-15));
#5762=CARTESIAN_POINT('Ctrl Pts',(-5.75643035625,50.3656249993855,-7.04959401029622E-16));
#5763=CARTESIAN_POINT('Ctrl Pts',(-5.75643035625,50.4031249993855,3.32347661575227));
#5764=CARTESIAN_POINT('Ctrl Pts',(-2.878215178125,50.4406249993855,4.9852149236284));
#5765=CARTESIAN_POINT('Ctrl Pts',(-1.22102549985663E-15,50.4781249993855,
6.64695323150454));
#5766=CARTESIAN_POINT('Ctrl Pts',(2.878215178125,50.5156249993855,4.98521492362841));
#5767=CARTESIAN_POINT('Ctrl Pts',(5.75643035625,50.5531249993855,3.32347661575227));
#5768=CARTESIAN_POINT('Ctrl Pts',(5.75643035625,50.5906249993855,0.));
#5769=CARTESIAN_POINT('Ctrl Pts',(5.75643035625,50.6281249993855,-3.32347661575227));
#5770=CARTESIAN_POINT('Ctrl Pts',(2.878215178125,50.6656249993855,-4.9852149236284));
#5771=CARTESIAN_POINT('Ctrl Pts',(4.0700849995221E-16,50.7031249993855,
-6.64695323150454));
#5772=CARTESIAN_POINT('Ctrl Pts',(-2.878215178125,50.7406249993855,-4.9852149236284));
#5773=CARTESIAN_POINT('Ctrl Pts',(-5.75643035625,50.7781249993855,-3.32347661575227));
#5774=CARTESIAN_POINT('Ctrl Pts',(-5.75643035625,50.8156249993855,-7.04959401029622E-16));
#5775=CARTESIAN_POINT('Ctrl Pts',(-5.75643035625,50.4781249993855,-7.04959401029622E-16));
#5776=CARTESIAN_POINT('Ctrl Pts',(-5.75643035625,50.5156249993855,3.32347661575227));
#5777=CARTESIAN_POINT('Ctrl Pts',(-2.878215178125,50.5531249993855,4.9852149236284));
#5778=CARTESIAN_POINT('Ctrl Pts',(-1.22102549985663E-15,50.5906249993855,
6.64695323150454));
#5779=CARTESIAN_POINT('Ctrl Pts',(2.878215178125,50.6281249993855,4.98521492362841));
#5780=CARTESIAN_POINT('Ctrl Pts',(5.75643035625,50.6656249993855,3.32347661575227));
#5781=CARTESIAN_POINT('Ctrl Pts',(5.75643035625,50.7031249993855,0.));
#5782=CARTESIAN_POINT('Ctrl Pts',(5.75643035625,50.7406249993855,-3.32347661575227));
#5783=CARTESIAN_POINT('Ctrl Pts',(2.878215178125,50.7781249993855,-4.9852149236284));
#5784=CARTESIAN_POINT('Ctrl Pts',(4.0700849995221E-16,50.8156249993855,
-6.64695323150454));
#5785=CARTESIAN_POINT('Ctrl Pts',(-2.878215178125,50.8531249993855,-4.9852149236284));
#5786=CARTESIAN_POINT('Ctrl Pts',(-5.75643035625,50.8906249993855,-3.32347661575227));
#5787=CARTESIAN_POINT('Ctrl Pts',(-5.75643035625,50.9281249993855,-7.04959401029622E-16));
#5788=CARTESIAN_POINT('Origin',(0.,50.,0.));
#5789=CARTESIAN_POINT('',(-1.07185518347685E-16,50.1125,-6.));
#5790=CARTESIAN_POINT('',(-7.34788079488412E-16,50.,-6.));
#5791=CARTESIAN_POINT('',(-7.34788079488412E-16,50.,-6.));
#5792=CARTESIAN_POINT('',(6.,50.,0.));
#5793=CARTESIAN_POINT('Ctrl Pts',(7.63278329429795E-16,50.1125,-6.));
#5794=CARTESIAN_POINT('Ctrl Pts',(0.343291227172437,50.1082088596603,-6.));
#5795=CARTESIAN_POINT('Ctrl Pts',(0.686759034749955,50.1039155120655,-5.97053821667675));
#5796=CARTESIAN_POINT('Ctrl Pts',(1.77491233708495,50.0903135957864,-5.78157134708829));
#5797=CARTESIAN_POINT('Ctrl Pts',(2.49179065334938,50.0815813989611,-5.51070121351748));
#5798=CARTESIAN_POINT('Ctrl Pts',(3.81594411981456,50.0645056281562,-4.69780943448951));
#5799=CARTESIAN_POINT('Ctrl Pts',(4.40362359624846,50.0549238334303,-4.15197805611787));
#5800=CARTESIAN_POINT('Ctrl Pts',(5.23987317830986,50.0371337154915,-2.99140627649053));
#5801=CARTESIAN_POINT('Ctrl Pts',(5.52735144341947,50.0291440981232,-2.41933269210065));
#5802=CARTESIAN_POINT('Ctrl Pts',(5.905418894506,50.0138685530285,-1.2265156251652));
#5803=CARTESIAN_POINT('Ctrl Pts',(6.,50.0066584470657,-0.615080992922631));
#5804=CARTESIAN_POINT('Ctrl Pts',(6.,50.,0.));
#5805=CARTESIAN_POINT('Origin',(0.,50.,0.));
#5806=CARTESIAN_POINT('Origin',(0.,50.,0.));
#5807=CARTESIAN_POINT('',(-1.52965876864867E-15,50.5625,-6.));
#5808=CARTESIAN_POINT('',(2.0935010245251E-14,50.506249998771,-6.));
#5809=CARTESIAN_POINT('',(-7.34788079488412E-16,50.,-6.));
#5810=CARTESIAN_POINT('Ctrl Pts',(1.11022302462516E-15,50.5625,-6.));
#5811=CARTESIAN_POINT('Ctrl Pts',(0.476472672014833,50.5565440915998,-6.));
#5812=CARTESIAN_POINT('Ctrl Pts',(0.952342916136355,50.5505957135482,-5.94324142107436));
#5813=CARTESIAN_POINT('Ctrl Pts',(2.15487129319964,50.535564108835,-5.65088635606439));
#5814=CARTESIAN_POINT('Ctrl Pts',(2.85164975918806,50.5274118357436,-5.33329821377427));
#5815=CARTESIAN_POINT('Ctrl Pts',(4.11877626853935,50.5097650355555,-4.4347324708146));
#5816=CARTESIAN_POINT('Ctrl Pts',(4.66914406878105,50.5000062126512,-3.85100602351549));
#5817=CARTESIAN_POINT('Ctrl Pts',(5.49975183061805,50.4804099614397,-2.52033349247185));
#5818=CARTESIAN_POINT('Ctrl Pts',(5.77873402031905,50.4707647501893,-1.79041748490187));
#5819=CARTESIAN_POINT('Ctrl Pts',(6.04305617758452,50.4526536893107,-0.269995813782789));
#5820=CARTESIAN_POINT('Ctrl Pts',(6.02788606094672,50.4446968849474,0.505980809288367));
#5821=CARTESIAN_POINT('Ctrl Pts',(5.69985850262359,50.4260858043139,2.03581199638024));
#5822=CARTESIAN_POINT('Ctrl Pts',(5.38000634383492,50.4161085580272,2.77280379910834));
#5823=CARTESIAN_POINT('Ctrl Pts',(4.48867993903998,50.3966646970468,4.05434319874371));
#5824=CARTESIAN_POINT('Ctrl Pts',(3.93535378351657,50.3873713829251,4.59335977946739));
#5825=CARTESIAN_POINT('Ctrl Pts',(2.63192129548323,50.369950097055,5.45013213550946));
#5826=CARTESIAN_POINT('Ctrl Pts',(1.88806980464463,50.361100872558,5.75031863985159));
#5827=CARTESIAN_POINT('Ctrl Pts',(0.335271683604976,50.341690896045,6.04191731940555));
#5828=CARTESIAN_POINT('Ctrl Pts',(-0.457848446331719,50.3317768944208,6.03386671313742));
#5829=CARTESIAN_POINT('Ctrl Pts',(-1.9694640440123,50.3128816994498,5.71810678616551));
#5830=CARTESIAN_POINT('Ctrl Pts',(-2.67595066180082,50.3044868675681,5.42354152179471));
#5831=CARTESIAN_POINT('Ctrl Pts',(-3.97145719940011,50.2871188781581,4.5671164322292));
#5832=CARTESIAN_POINT('Ctrl Pts',(-4.54056698419253,50.2774420154712,4.0017818353245));
#5833=CARTESIAN_POINT('Ctrl Pts',(-5.4156177211193,50.2578490970685,2.69707633960295));
#5834=CARTESIAN_POINT('Ctrl Pts',(-5.71889044460288,50.2481281972586,1.97419266862997));
#5835=CARTESIAN_POINT('Ctrl Pts',(-6.03066858894288,50.2298384149222,0.464660143335277));
#5836=CARTESIAN_POINT('Ctrl Pts',(-6.04074643451833,50.2219311981155,-0.30700873998632));
#5837=CARTESIAN_POINT('Ctrl Pts',(-5.76467205805915,50.2035512699327,-1.84548216186661));
#5838=CARTESIAN_POINT('Ctrl Pts',(-5.46827631697157,50.1935825943994,-2.5952248013838));
#5839=CARTESIAN_POINT('Ctrl Pts',(-4.61606755786416,50.1740325956351,-3.90915337278197));
#5840=CARTESIAN_POINT('Ctrl Pts',(-4.0784439382076,50.1646314228256,-4.46719937561014));
#5841=CARTESIAN_POINT('Ctrl Pts',(-2.80731661670282,50.1470149884145,-5.36065017826871));
#5842=CARTESIAN_POINT('Ctrl Pts',(-2.08181074478282,50.1385226343097,-5.68187235150351));
#5843=CARTESIAN_POINT('Ctrl Pts',(-0.882392025536312,50.1235299003191,-5.95130335519231));
#5844=CARTESIAN_POINT('Ctrl Pts',(-0.441341940389351,50.1180167742549,-6.));
#5845=CARTESIAN_POINT('Ctrl Pts',(9.71445146547012E-16,50.1125,-6.));
#5846=CARTESIAN_POINT('Origin',(0.,50.,0.));
#5847=CARTESIAN_POINT('',(6.,50.393749998771,0.));
#5848=CARTESIAN_POINT('',(6.,50.1968749993855,0.));
#5849=CARTESIAN_POINT('Ctrl Pts',(6.,50.393749998771,0.));
#5850=CARTESIAN_POINT('Ctrl Pts',(6.,50.3988676934681,-0.472752385765871));
#5851=CARTESIAN_POINT('Ctrl Pts',(5.94412631061322,50.4043166770945,-0.943849242317885));
#5852=CARTESIAN_POINT('Ctrl Pts',(5.71905899328923,50.4158503124434,-1.87933816182198));
#5853=CARTESIAN_POINT('Ctrl Pts',(5.54677711349615,50.4219074269274,-2.33940344059781));
#5854=CARTESIAN_POINT('Ctrl Pts',(4.95121361381124,50.437998009178,-3.48193901273638));
#5855=CARTESIAN_POINT('Ctrl Pts',(4.4440452275349,50.4479625421736,-4.10960933757635));
#5856=CARTESIAN_POINT('Ctrl Pts',(3.24080528215491,50.466278937471,-5.10691455209658));
#5857=CARTESIAN_POINT('Ctrl Pts',(2.56504807180657,50.4741868978735,-5.4775838590699));
#5858=CARTESIAN_POINT('Ctrl Pts',(1.24316375970988,50.4907104517747,-5.9029624523061));
#5859=CARTESIAN_POINT('Ctrl Pts',(0.622991567293922,50.4984626041798,-6.));
#5860=CARTESIAN_POINT('Ctrl Pts',(3.63598040564739E-14,50.506249998771,
-6.));
#5861=CARTESIAN_POINT('Origin',(0.,50.,0.));
#5862=CARTESIAN_POINT('',(5.8776104737723E-15,51.0125,-6.));
#5863=CARTESIAN_POINT('',(3.65716442452199E-15,50.956249998771,-6.));
#5864=CARTESIAN_POINT('',(-7.34788079488412E-16,50.,-6.));
#5865=CARTESIAN_POINT('Ctrl Pts',(1.58206781009085E-14,51.0125,-6.));
#5866=CARTESIAN_POINT('Ctrl Pts',(0.601653563824407,51.0049793304522,-6.));
#5867=CARTESIAN_POINT('Ctrl Pts',(1.20092291143887,50.9974884636069,-5.90949606770874));
#5868=CARTESIAN_POINT('Ctrl Pts',(2.50594358432149,50.9811757051959,-5.5047255931851));
#5869=CARTESIAN_POINT('Ctrl Pts',(3.1847068740602,50.9732585574772,-5.14192541668118));
#5870=CARTESIAN_POINT('Ctrl Pts',(4.39882179499044,50.9550207007929,-4.15815395852777));
#5871=CARTESIAN_POINT('Ctrl Pts',(4.91338690974145,50.9450623040753,-3.53532098195299));
#5872=CARTESIAN_POINT('Ctrl Pts',(5.65350068693484,50.9254580943553,-2.15166654899081));
#5873=CARTESIAN_POINT('Ctrl Pts',(5.88251857425753,50.9159965307216,-1.40986827814802));
#5874=CARTESIAN_POINT('Ctrl Pts',(6.04922997596698,50.8982658107267,0.131774603112445));
#5875=CARTESIAN_POINT('Ctrl Pts',(5.98068299604821,50.8899459720277,0.91759864356742));
#5876=CARTESIAN_POINT('Ctrl Pts',(5.5438020044826,50.8708757505391,2.42699688707256));
#5877=CARTESIAN_POINT('Ctrl Pts',(5.17645209976913,50.8609151616119,3.13502711244388));
#5878=CARTESIAN_POINT('Ctrl Pts',(4.20694003529658,50.8417559174161,4.34513422806219));
#5879=CARTESIAN_POINT('Ctrl Pts',(3.62280363610034,50.8327850454512,4.84291099325534));
#5880=CARTESIAN_POINT('Ctrl Pts',(2.27059691795816,50.8158824614744,5.61026834862654));
#5881=CARTESIAN_POINT('Ctrl Pts',(1.50889267209935,50.8063611584012,5.86122364397982));
#5882=CARTESIAN_POINT('Ctrl Pts',(-0.054498498555203,50.786818768768,6.05032206138634));
#5883=CARTESIAN_POINT('Ctrl Pts',(-0.840368151589543,50.7769953981051,5.99192403302677));
#5884=CARTESIAN_POINT('Ctrl Pts',(-2.32593591816436,50.7584258010229,5.58283012690718));
#5885=CARTESIAN_POINT('Ctrl Pts',(-3.01389064873413,50.7504258757977,5.24351291353162));
#5886=CARTESIAN_POINT('Ctrl Pts',(-4.26025821447966,50.732427877307,4.30051967936572));
#5887=CARTESIAN_POINT('Ctrl Pts',(-4.79671255812451,50.7224948600111,3.69266890552999));
#5888=CARTESIAN_POINT('Ctrl Pts',(-5.58313950087653,50.702816769394,2.32892856624056));
#5889=CARTESIAN_POINT('Ctrl Pts',(-5.83606608898751,50.6932626947642,1.59238819047398));
#5890=CARTESIAN_POINT('Ctrl Pts',(-6.04952440528675,50.675347728897,0.0607147482980532));
#5891=CARTESIAN_POINT('Ctrl Pts',(-6.00680377993718,50.667245707192,-0.720239050576822));
#5892=CARTESIAN_POINT('Ctrl Pts',(-5.62238021193402,50.6483922983037,-2.23989531159852));
#5893=CARTESIAN_POINT('Ctrl Pts',(-5.27762720706178,50.6384178537405,-2.96225179199993));
#5894=CARTESIAN_POINT('Ctrl Pts',(-4.34514342194628,50.6191112625712,-4.20734852504976));
#5895=CARTESIAN_POINT('Ctrl Pts',(-3.77550374701531,50.6099449611129,-4.72521356370631));
#5896=CARTESIAN_POINT('Ctrl Pts',(-2.44599834298937,50.5928577967403,-5.53606789283227));
#5897=CARTESIAN_POINT('Ctrl Pts',(-1.69240519125137,50.5836550648906,-5.81091707152203));
#5898=CARTESIAN_POINT('Ctrl Pts',(-0.606296241288776,50.5700787030161,-5.97704427499298));
#5899=CARTESIAN_POINT('Ctrl Pts',(-0.303026289114533,50.5662878286139,-6.));
#5900=CARTESIAN_POINT('Ctrl Pts',(4.85722573273506E-16,50.5625,-6.));
#5901=CARTESIAN_POINT('Ctrl Pts',(3.5978164891759E-14,50.506249998771,-6.));
#5902=CARTESIAN_POINT('Ctrl Pts',(-0.152003403865639,50.5081500413193,-6.));
#5903=CARTESIAN_POINT('Ctrl Pts',(-0.304174647594184,50.510052181866,-5.99422385574095));
#5904=CARTESIAN_POINT('Ctrl Pts',(-1.2482173623285,50.5218527158001,-5.92223895805082));
#5905=CARTESIAN_POINT('Ctrl Pts',(-2.02043362015721,50.531505419023,-5.70515799936607));
#5906=CARTESIAN_POINT('Ctrl Pts',(-3.40371495283626,50.5487964356815,-4.99904116312216));
#5907=CARTESIAN_POINT('Ctrl Pts',(-4.00797797076151,50.5572720195484,-4.52899800173635));
#5908=CARTESIAN_POINT('Ctrl Pts',(-5.02743121692379,50.5762120737144,-3.36797234844005));
#5909=CARTESIAN_POINT('Ctrl Pts',(-5.42507403926348,50.5861358260319,-2.6808345674558));
#5910=CARTESIAN_POINT('Ctrl Pts',(-5.93450499841088,50.605491209983,-1.18698088734165));
#5911=CARTESIAN_POINT('Ctrl Pts',(-6.03919864626748,50.6142384889631,-0.394124075355784));
#5912=CARTESIAN_POINT('Ctrl Pts',(-5.93632777073841,50.6317114764584,1.16056884240303));
#5913=CARTESIAN_POINT('Ctrl Pts',(-5.73980587496678,50.6410339113833,1.90827652312679));
#5914=CARTESIAN_POINT('Ctrl Pts',(-5.06310523712295,50.6605074794676,3.31647439179314));
#5915=CARTESIAN_POINT('Ctrl Pts',(-4.57877433964754,50.6704835153468,3.95839253781037));
#5916=CARTESIAN_POINT('Ctrl Pts',(-3.40909054731109,50.6890347370683,4.99676374218396));
#5917=CARTESIAN_POINT('Ctrl Pts',(-2.74234841966966,50.6969706435252,5.39157404784597));
#5918=CARTESIAN_POINT('Ctrl Pts',(-1.28970228179228,50.7151287202487,5.91075385984872));
#5919=CARTESIAN_POINT('Ctrl Pts',(-0.516435295961029,50.7247945575715,6.02773819372563));
#5920=CARTESIAN_POINT('Ctrl Pts',(1.05135832519143,50.7443919778359,5.96034931905182));
#5921=CARTESIAN_POINT('Ctrl Pts',(1.83043851808684,50.7541304802471,5.7689366459716));
#5922=CARTESIAN_POINT('Ctrl Pts',(3.23642006657542,50.7717052496032,5.10894082885421));
#5923=CARTESIAN_POINT('Ctrl Pts',(3.85590385180355,50.7799125840591,4.65915328260332));
#5924=CARTESIAN_POINT('Ctrl Pts',(4.911409365443,50.7986849582154,3.53443203143811));
#5925=CARTESIAN_POINT('Ctrl Pts',(5.33057380493307,50.8085687334406,2.86341268750622));
#5926=CARTESIAN_POINT('Ctrl Pts',(5.89333911364858,50.8281220796084,1.38206464221782));
#5927=CARTESIAN_POINT('Ctrl Pts',(6.02499747152435,50.8372730161237,0.583885731075924));
#5928=CARTESIAN_POINT('Ctrl Pts',(5.96852424689707,50.8545542654857,-0.979882872856363));
#5929=CARTESIAN_POINT('Ctrl Pts',(5.79544146966376,50.8637668988012,-1.7309800967731));
#5930=CARTESIAN_POINT('Ctrl Pts',(5.16480946229501,50.8831249119008,-3.15510118940353));
#5931=CARTESIAN_POINT('Ctrl Pts',(4.70262726478869,50.8931017932574,-3.80988499516316));
#5932=CARTESIAN_POINT('Ctrl Pts',(3.56553255119832,50.9118700954101,-4.88712454418799));
#5933=CARTESIAN_POINT('Ctrl Pts',(2.90721926588576,50.9199097579474,-5.30519385869809));
#5934=CARTESIAN_POINT('Ctrl Pts',(1.49047678297696,50.9376190389837,-5.8599679154867));
#5935=CARTESIAN_POINT('Ctrl Pts',(0.748406815975599,50.9468949135713,-6.));
#5936=CARTESIAN_POINT('Ctrl Pts',(8.74300631892311E-15,50.956249998771,
-6.));
#5937=CARTESIAN_POINT('Origin',(0.,50.,0.));
#5938=CARTESIAN_POINT('',(-6.44949795900495E-16,51.4625,-6.));
#5939=CARTESIAN_POINT('',(-3.06903603998188E-14,51.406249998771,-6.));
#5940=CARTESIAN_POINT('',(-7.34788079488412E-16,50.,-6.));
#5941=CARTESIAN_POINT('Ctrl Pts',(2.35922392732846E-15,51.4625,-6.));
#5942=CARTESIAN_POINT('Ctrl Pts',(0.729126527437651,51.453385918407,-6.));
#5943=CARTESIAN_POINT('Ctrl Pts',(1.45257389413295,51.4443428263233,-5.86708753239055));
#5944=CARTESIAN_POINT('Ctrl Pts',(2.85524232401819,51.4268094709497,-5.33310950763709));
#5945=CARTESIAN_POINT('Ctrl Pts',(3.51622153328107,51.4188108537407,-4.92246422249686));
#5946=CARTESIAN_POINT('Ctrl Pts',(4.66374479001418,51.4001108312203,-3.85755299791155));
#5947=CARTESIAN_POINT('Ctrl Pts',(5.13300751731751,51.3901331471364,-3.20678298515835));
#5948=CARTESIAN_POINT('Ctrl Pts',(5.77833250827751,51.3707364282851,-1.78756940637938));
#5949=CARTESIAN_POINT('Ctrl Pts',(5.95887574118884,51.3614879927408,-1.03747221033125));
#5950=CARTESIAN_POINT('Ctrl Pts',(6.03015613730497,51.3441451457851,0.5234376111266));
#5951=CARTESIAN_POINT('Ctrl Pts',(5.90716967249953,51.335131443154,1.31990283301873));
#5952=CARTESIAN_POINT('Ctrl Pts',(5.36147739674722,51.315640345333,2.80535774252139));
#5953=CARTESIAN_POINT('Ctrl Pts',(4.94913149322012,51.3057425956967,3.48160467082276));
#5954=CARTESIAN_POINT('Ctrl Pts',(3.90511006403264,51.286915968157,4.61796797412313));
#5955=CARTESIAN_POINT('Ctrl Pts',(3.29054200038651,51.2786317750047,5.0742320508147));
#5956=CARTESIAN_POINT('Ctrl Pts',(1.89181182918552,51.2611476478647,5.74909877162617));
#5957=CARTESIAN_POINT('Ctrl Pts',(1.11484561480856,51.251435570185,5.9487973907187));
#5958=CARTESIAN_POINT('Ctrl Pts',(-0.452903530529944,51.2318387058683,6.03294646757653));
#5959=CARTESIAN_POINT('Ctrl Pts',(-1.22816139551171,51.222147982556,5.92395084746659));
#5960=CARTESIAN_POINT('Ctrl Pts',(-2.68547298581604,51.2039315876772,5.41992639145892));
#5961=CARTESIAN_POINT('Ctrl Pts',(-3.35510942912662,51.1960138719864,5.03295221414885));
#5962=CARTESIAN_POINT('Ctrl Pts',(-4.53571663874673,51.177537843469,4.00783369833812));
#5963=CARTESIAN_POINT('Ctrl Pts',(-5.02748153880361,51.1675643401458,3.37044152321714));
#5964=CARTESIAN_POINT('Ctrl Pts',(-5.71971656360589,51.1480556848537,1.96797121961757));
#5965=CARTESIAN_POINT('Ctrl Pts',(-5.92417386032965,51.1386978639832,1.22157623114418));
#5966=CARTESIAN_POINT('Ctrl Pts',(-6.04267856970106,51.1211611102462,-0.329980961522083));
#5967=CARTESIAN_POINT('Ctrl Pts',(-5.94693589479211,51.1125322987399,-1.12108033315413));
#5968=CARTESIAN_POINT('Ctrl Pts',(-5.45536444033585,51.0932454615163,-2.61891312766104));
#5969=CARTESIAN_POINT('Ctrl Pts',(-5.06507198158196,51.0833107530727,-3.31130672661132));
#5970=CARTESIAN_POINT('Ctrl Pts',(-4.05781210853169,51.0643157595439,-4.48444730810267));
#5971=CARTESIAN_POINT('Ctrl Pts',(-3.45856108428655,51.0557320135535,-4.96129373331203));
#5972=CARTESIAN_POINT('Ctrl Pts',(-2.08291035391032,51.0385363794238,-5.68264072765549));
#5973=CARTESIAN_POINT('Ctrl Pts',(-1.3131598757117,51.0289144984463,-5.90817338077523));
#5974=CARTESIAN_POINT('Ctrl Pts',(-0.348046647051617,51.0168505830881,-5.99243780840527));
#5975=CARTESIAN_POINT('Ctrl Pts',(-0.17392370497713,51.0146740463122,-6.));
#5976=CARTESIAN_POINT('Ctrl Pts',(1.70696790036118E-14,51.0125,-6.));
#5977=CARTESIAN_POINT('Ctrl Pts',(8.92450088600247E-15,50.956249998771,
-6.));
#5978=CARTESIAN_POINT('Ctrl Pts',(-0.0236694939700509,50.9565458674456,
-6.));
#5979=CARTESIAN_POINT('Ctrl Pts',(-0.0473453262845365,50.9568418153495,
-5.99985993888696));
#5980=CARTESIAN_POINT('Ctrl Pts',(-0.865475177989564,50.9670684384958,-5.99017447353904));
#5981=CARTESIAN_POINT('Ctrl Pts',(-1.65020552722794,50.9768775678613,-5.82306397465396));
#5982=CARTESIAN_POINT('Ctrl Pts',(-3.07704855133587,50.9947131056627,-5.20663568267979));
#5983=CARTESIAN_POINT('Ctrl Pts',(-3.71098632648849,51.002746826765,-4.77554919943315));
#5984=CARTESIAN_POINT('Ctrl Pts',(-4.79939869161664,51.0213594783246,-3.68458126930465));
#5985=CARTESIAN_POINT('Ctrl Pts',(-5.2378834734425,51.0311967083489,-3.02901619171069));
#5986=CARTESIAN_POINT('Ctrl Pts',(-5.84386020371629,51.0507264147932,-1.57480001640781));
#5987=CARTESIAN_POINT('Ctrl Pts',(-6.00076345356614,51.0602111642092,-0.788342969138268));
#5988=CARTESIAN_POINT('Ctrl Pts',(-5.99926273157664,51.077057562383,0.766994191899727));
#5989=CARTESIAN_POINT('Ctrl Pts',(-5.85367677494241,51.0861313952624,1.52114487752692));
#5990=CARTESIAN_POINT('Ctrl Pts',(-5.27743730941944,51.105331307234,2.96206476222724));
#5991=CARTESIAN_POINT('Ctrl Pts',(-4.84159877308954,51.1152966396318,3.63099124074761));
#5992=CARTESIAN_POINT('Ctrl Pts',(-3.74344507819321,51.1343099694806,4.75334808640714));
#5993=CARTESIAN_POINT('Ctrl Pts',(-3.09486583810597,51.1425641757947,5.19899003599694));
#5994=CARTESIAN_POINT('Ctrl Pts',(-1.67246967653445,51.1603441278144,5.81339415782086));
#5995=CARTESIAN_POINT('Ctrl Pts',(-0.913518401626463,51.1698310187507,5.97981409959571));
#5996=CARTESIAN_POINT('Ctrl Pts',(0.656532155170128,51.1894566507107,6.01747330048976));
#5997=CARTESIAN_POINT('Ctrl Pts',(1.45274859455488,51.199409356203,5.87627039081847));
#5998=CARTESIAN_POINT('Ctrl Pts',(2.90675574161729,51.2175844455413,5.30390036844112));
#5999=CARTESIAN_POINT('Ctrl Pts',(3.55614425565295,51.2255153876614,4.8922826028945));
#6000=CARTESIAN_POINT('Ctrl Pts',(4.67836403780843,51.2439575069591,3.83658648965518));
#6001=CARTESIAN_POINT('Ctrl Pts',(5.13631558728198,51.2537367738425,3.19761496120145));
#6002=CARTESIAN_POINT('Ctrl Pts',(5.78886518522972,51.2733094150932,1.76632149606204));
#6003=CARTESIAN_POINT('Ctrl Pts',(5.97159814210816,51.2829059092566,0.985336259740639));
#6004=CARTESIAN_POINT('Ctrl Pts',(6.02117430454731,51.3000251205363,-0.567445928026152));
#6005=CARTESIAN_POINT('Ctrl Pts',(5.90112590328245,51.3087019176556,-1.32411411650511));
#6006=CARTESIAN_POINT('Ctrl Pts',(5.37550568819043,51.3277404092649,-2.77934766473404));
#6007=CARTESIAN_POINT('Ctrl Pts',(4.96446005702314,51.3376829976343,-3.46048733037337));
#6008=CARTESIAN_POINT('Ctrl Pts',(3.90324713248807,51.3569142092584,-4.62429899600857));
#6009=CARTESIAN_POINT('Ctrl Pts',(3.26364678912653,51.3654544139069,-5.09588808413548));
#6010=CARTESIAN_POINT('Ctrl Pts',(1.85663770964007,51.3830420274005,-5.75690279586834));
#6011=CARTESIAN_POINT('Ctrl Pts',(1.10578919839712,51.3924276337911,-5.94695282907335));
#6012=CARTESIAN_POINT('Ctrl Pts',(0.226339583391152,51.4034207539786,-5.99680138535396));
#6013=CARTESIAN_POINT('Ctrl Pts',(0.113113412960351,51.404836081109,-6.));
#6014=CARTESIAN_POINT('Ctrl Pts',(-7.18522463749593E-14,51.406249998771,
-6.));
#6015=CARTESIAN_POINT('Origin',(0.,50.,0.));
#6016=CARTESIAN_POINT('',(4.48983169299085E-15,51.9125,-6.));
#6017=CARTESIAN_POINT('',(-7.61853816932726E-15,51.856249998771,-6.));
#6018=CARTESIAN_POINT('',(-7.34788079488412E-16,50.,-6.));
#6019=CARTESIAN_POINT('Ctrl Pts',(1.57666182319377E-14,51.9125,-6.));
#6020=CARTESIAN_POINT('Ctrl Pts',(0.0924430517342845,51.9113444618533,-6.));
#6021=CARTESIAN_POINT('Ctrl Pts',(0.184967191480457,51.9101879101064,-5.99786359346722));
#6022=CARTESIAN_POINT('Ctrl Pts',(1.04490904993104,51.8994386368758,-5.95804877519037));
#6023=CARTESIAN_POINT('Ctrl Pts',(1.79840667952007,51.8900199165059,-5.77545917468654));
#6024=CARTESIAN_POINT('Ctrl Pts',(3.21034451142012,51.8723706936072,-5.12924978043591));
#6025=CARTESIAN_POINT('Ctrl Pts',(3.85280973532281,51.8639306708006,-4.66598152208977));
#6026=CARTESIAN_POINT('Ctrl Pts',(4.92589999521266,51.8447679633295,-3.51535538180445));
#6027=CARTESIAN_POINT('Ctrl Pts',(5.34489191970669,51.834816864418,-2.83801734055718));
#6028=CARTESIAN_POINT('Ctrl Pts',(5.88665914109795,51.8157260815796,-1.38727581393923));
#6029=CARTESIAN_POINT('Ctrl Pts',(6.0148587668374,51.8069285111895,-0.631449735032211));
#6030=CARTESIAN_POINT('Ctrl Pts',(5.98166780649966,51.7899022768464,0.922203612083062));
#6031=CARTESIAN_POINT('Ctrl Pts',(5.80720587787156,51.7803374787255,1.7050361738104));
#6032=CARTESIAN_POINT('Ctrl Pts',(5.16952332359099,51.7607764201622,3.14384316778836));
#6033=CARTESIAN_POINT('Ctrl Pts',(4.71775764789522,51.750977473331,3.78820406783819));
#6034=CARTESIAN_POINT('Ctrl Pts',(3.60636022497298,51.7324800640207,4.85525594567499));
#6035=CARTESIAN_POINT('Ctrl Pts',(2.96198649019483,51.7245248311274,5.27313724558066));
#6036=CARTESIAN_POINT('Ctrl Pts',(1.51407230849546,51.7064259038562,5.86088842016826));
#6037=CARTESIAN_POINT('Ctrl Pts',(0.718481536179256,51.6964810192022,6.01050736255478));
#6038=CARTESIAN_POINT('Ctrl Pts',(-0.853487612076338,51.676831404849,5.98877294558987));
#6039=CARTESIAN_POINT('Ctrl Pts',(-1.61481130609958,51.6673148586737,5.82977189026946));
#6040=CARTESIAN_POINT('Ctrl Pts',(-3.04190771790022,51.6494761535262,5.22983997346207));
#6041=CARTESIAN_POINT('Ctrl Pts',(-3.69325542961239,51.6412932439949,4.79210796388247));
#6042=CARTESIAN_POINT('Ctrl Pts',(-4.80261373614584,51.6223488062732,3.68258408586089));
#6043=CARTESIAN_POINT('Ctrl Pts',(-5.24601376188035,51.6123788015796,3.01759162709253));
#6044=CARTESIAN_POINT('Ctrl Pts',(-5.8378222397197,51.5931312744607,1.58126201695301));
#6045=CARTESIAN_POINT('Ctrl Pts',(-5.99125937980607,51.5840167139538,0.827881957130522));
#6046=CARTESIAN_POINT('Ctrl Pts',(-6.0083699018476,51.567064754705,-0.728194196054372));
#6047=CARTESIAN_POINT('Ctrl Pts',(-5.85933185788279,51.5577068077806,-1.51626187955861));
#6048=CARTESIAN_POINT('Ctrl Pts',(-5.26760096122616,51.5381929901524,-2.97723514477735));
#6049=CARTESIAN_POINT('Ctrl Pts',(-4.83513639153481,51.5283401250748,-3.63772029782657));
#6050=CARTESIAN_POINT('Ctrl Pts',(-3.7570404965506,51.5096767262397,-4.7393322772767));
#6051=CARTESIAN_POINT('Ctrl Pts',(-3.12769439993587,51.5015961799992,-5.17630593696793));
#6052=CARTESIAN_POINT('Ctrl Pts',(-1.70740286678856,51.4838425358348,-5.806547484345));
#6053=CARTESIAN_POINT('Ctrl Pts',(-0.924376327007982,51.4740547040876,-5.98136532622966));
#6054=CARTESIAN_POINT('Ctrl Pts',(-0.0867051686540407,51.4635838146081,
-5.99953035711345));
#6055=CARTESIAN_POINT('Ctrl Pts',(-0.0433425502532464,51.4630417818782,
-6.));
#6056=CARTESIAN_POINT('Ctrl Pts',(8.92450088600248E-16,51.4625,-6.));
#6057=CARTESIAN_POINT('Ctrl Pts',(-6.84174938925253E-14,51.406249998771,
-6.));
#6058=CARTESIAN_POINT('Ctrl Pts',(-0.682829483794224,51.4147853673184,-5.99999999999999));
#6059=CARTESIAN_POINT('Ctrl Pts',(-1.36154991554759,51.4232693727154,-5.88342572703261));
#6060=CARTESIAN_POINT('Ctrl Pts',(-2.72788892000143,51.440348610271,-5.3985522850297));
#6061=CARTESIAN_POINT('Ctrl Pts',(-3.39356269799421,51.4482580185231,-5.0069429255558));
#6062=CARTESIAN_POINT('Ctrl Pts',(-4.54997486002227,51.4665211913447,-3.98751815942739));
#6063=CARTESIAN_POINT('Ctrl Pts',(-5.02716012934551,51.4762312989628,-3.36603988357486));
#6064=CARTESIAN_POINT('Ctrl Pts',(-5.72633526724286,51.4958260731568,-1.95962113275784));
#6065=CARTESIAN_POINT('Ctrl Pts',(-5.93519982653713,51.5055159610265,-1.1850956430917));
#6066=CARTESIAN_POINT('Ctrl Pts',(-6.03676786753935,51.5229263324305,0.36456523978062));
#6067=CARTESIAN_POINT('Ctrl Pts',(-5.94237522903659,51.5312792187735,1.12413008956238));
#6068=CARTESIAN_POINT('Ctrl Pts',(-5.46740692741677,51.5501495145695,2.59307026996213));
#6069=CARTESIAN_POINT('Ctrl Pts',(-5.08150263678972,51.5600578002235,3.28555654622167));
#6070=CARTESIAN_POINT('Ctrl Pts',(-4.05814773950216,51.5794975557433,4.49049001396925));
#6071=CARTESIAN_POINT('Ctrl Pts',(-3.42757426035077,51.5884053205166,4.98846414670857));
#6072=CARTESIAN_POINT('Ctrl Pts',(-2.03615645946408,51.6057980430277,5.69556957119916));
#6073=CARTESIAN_POINT('Ctrl Pts',(-1.29399110079178,51.6150751100111,5.90855443995147));
#6074=CARTESIAN_POINT('Ctrl Pts',(0.260167210419777,51.6345020889012,6.04686735307427));
#6075=CARTESIAN_POINT('Ctrl Pts',(1.05837508521773,51.6444796873362,5.95920647898521));
#6076=CARTESIAN_POINT('Ctrl Pts',(2.54987339008844,51.6631234161471,5.48549489205059));
#6077=CARTESIAN_POINT('Ctrl Pts',(3.23185121945399,51.6710940591096,5.11347676787178));
#6078=CARTESIAN_POINT('Ctrl Pts',(4.42112424819284,51.6891792491168,4.12946558011599));
#6079=CARTESIAN_POINT('Ctrl Pts',(4.91630755110058,51.6988129017285,3.52544108476394));
#6080=CARTESIAN_POINT('Ctrl Pts',(5.65969707009764,51.7184079064646,2.14452822220431));
#6081=CARTESIAN_POINT('Ctrl Pts',(5.89362134311647,51.7281775430302,1.37710409603449));
#6082=CARTESIAN_POINT('Ctrl Pts',(6.04546282587192,51.7458635868776,-0.168996931216874));
#6083=CARTESIAN_POINT('Ctrl Pts',(5.97562959130781,51.7539881263655,-0.931687453613559));
#6084=CARTESIAN_POINT('Ctrl Pts',(5.54880763948184,51.7726930088022,-2.41314471042416));
#6085=CARTESIAN_POINT('Ctrl Pts',(5.18706468357243,51.7825580768145,-3.11558826504987));
#6086=CARTESIAN_POINT('Ctrl Pts',(4.20705474315048,51.8020573823026,-4.35104794574967));
#6087=CARTESIAN_POINT('Ctrl Pts',(3.59473708496763,51.8113157852089,-4.86916354403048));
#6088=CARTESIAN_POINT('Ctrl Pts',(2.23171010459133,51.8283536224636,-5.62147602523948));
#6089=CARTESIAN_POINT('Ctrl Pts',(1.49991165226443,51.8375011031177,-5.85933176219644));
#6090=CARTESIAN_POINT('Ctrl Pts',(0.496159456164859,51.8500480055689,-5.98463166999933));
#6091=CARTESIAN_POINT('Ctrl Pts',(0.247941674568198,51.8531507278389,-6.));
#6092=CARTESIAN_POINT('Ctrl Pts',(-1.17267306976032E-14,51.856249998771,
-6.));
#6093=CARTESIAN_POINT('Origin',(0.,50.,0.));
#6094=CARTESIAN_POINT('',(-9.45734505386267E-15,52.3625,-6.));
#6095=CARTESIAN_POINT('',(3.17965476092108E-14,52.306249998771,-6.));
#6096=CARTESIAN_POINT('',(-7.34788079488412E-16,50.,-6.));
#6097=CARTESIAN_POINT('Ctrl Pts',(-1.50573997714787E-14,52.3625,-6.));
#6098=CARTESIAN_POINT('Ctrl Pts',(0.218867784195469,52.3597641526975,-6.));
#6099=CARTESIAN_POINT('Ctrl Pts',(0.437994839314629,52.3570250645085,-5.98802456173197));
#6100=CARTESIAN_POINT('Ctrl Pts',(1.41543341424493,52.3448070823219,-5.88044745416016));
#6101=CARTESIAN_POINT('Ctrl Pts',(2.15159544557699,52.3356050569302,-5.65276652575058));
#6102=CARTESIAN_POINT('Ctrl Pts',(3.5326476238168,52.3183419047022,-4.9156222040165));
#6103=CARTESIAN_POINT('Ctrl Pts',(4.15722311421762,52.309149330625,-4.40005338233782));
#6104=CARTESIAN_POINT('Ctrl Pts',(5.15516415149115,52.2895779417722,-3.16828744922857));
#6105=CARTESIAN_POINT('Ctrl Pts',(5.5243713275488,52.2796984718593,-2.46882297352484));
#6106=CARTESIAN_POINT('Ctrl Pts',(5.96601865302547,52.260942102291,-0.991168972694993));
#6107=CARTESIAN_POINT('Ctrl Pts',(6.04343622383244,52.2527556742411,-0.229480366865192));
#6108=CARTESIAN_POINT('Ctrl Pts',(5.90716500607145,52.2351543708734,1.31778216686378));
#6109=CARTESIAN_POINT('Ctrl Pts',(5.6809768157088,52.2254083123868,2.08749467279664));
#6110=CARTESIAN_POINT('Ctrl Pts',(4.95118396568992,52.2058111553387,3.47645639791216));
#6111=CARTESIAN_POINT('Ctrl Pts',(4.46150970175715,52.1961528277785,4.08594091250292));
#6112=CARTESIAN_POINT('Ctrl Pts',(3.28239385516863,52.1780120002128,5.08095592961064));
#6113=CARTESIAN_POINT('Ctrl Pts',(2.60552540851252,52.1700690676063,5.45907142385025));
#6114=CARTESIAN_POINT('Ctrl Pts',(1.11966447758211,52.1514958059697,5.94810747115647));
#6115=CARTESIAN_POINT('Ctrl Pts',(0.321539219409664,52.1415192402425,6.04402472627572));
#6116=CARTESIAN_POINT('Ctrl Pts',(-1.23548602561916,52.1220564246797,5.92115850706941));
#6117=CARTESIAN_POINT('Ctrl Pts',(-1.98043099831077,52.112744612521,5.71528246658319));
#6118=CARTESIAN_POINT('Ctrl Pts',(-3.37675500006653,52.0952905624991,5.02256114425858));
#6119=CARTESIAN_POINT('Ctrl Pts',(-4.01016585633895,52.0865065480969,4.5329002576292));
#6120=CARTESIAN_POINT('Ctrl Pts',(-5.04548116745655,52.0671310648902,3.34080935998954));
#6121=CARTESIAN_POINT('Ctrl Pts',(-5.43929549024786,52.0572107945729,2.65178284716393));
#6122=CARTESIAN_POINT('Ctrl Pts',(-5.93013334981965,52.0382871396683,1.18707585699749));
#6123=CARTESIAN_POINT('Ctrl Pts',(-6.03258076592942,52.0298418558513,0.428460970690471));
#6124=CARTESIAN_POINT('Ctrl Pts',(-5.94739993750873,52.0125226070565,-1.12224352770716));
#6125=CARTESIAN_POINT('Ctrl Pts',(-5.74675091534023,52.0028609677718,-1.89890276744292));
#6126=CARTESIAN_POINT('Ctrl Pts',(-5.06217758730424,51.9832707673024,-3.31332937453221));
#6127=CARTESIAN_POINT('Ctrl Pts',(-4.59098826977479,51.9735377654933,-3.94038428954526));
#6128=CARTESIAN_POINT('Ctrl Pts',(-3.44532941940595,51.9552176218423,-4.97128022283922));
#6129=CARTESIAN_POINT('Ctrl Pts',(-2.78485079836899,51.9473106349795,-5.36922030587082));
#6130=CARTESIAN_POINT('Ctrl Pts',(-1.40463504649034,51.930057938081,-5.87584866556839));
#6131=CARTESIAN_POINT('Ctrl Pts',(-0.704673407088873,51.9213084175886,-6.));
#6132=CARTESIAN_POINT('Ctrl Pts',(1.67921232474555E-14,51.9125,-6.));
#6133=CARTESIAN_POINT('Ctrl Pts',(-1.37390099297363E-14,51.856249998771,
-6.));
#6134=CARTESIAN_POINT('Ctrl Pts',(-0.540992756444157,51.8630124082265,-5.99999999999999));
#6135=CARTESIAN_POINT('Ctrl Pts',(-1.08067101073368,51.8697583864051,-5.92682708894602));
#6136=CARTESIAN_POINT('Ctrl Pts',(-2.35171422551525,51.8856464265899,-5.57416455518408));
#6137=CARTESIAN_POINT('Ctrl Pts',(-3.05199153231469,51.8937765567516,-5.22371642671806));
#6138=CARTESIAN_POINT('Ctrl Pts',(-4.27665041483106,51.911663563064,-4.27844269669845));
#6139=CARTESIAN_POINT('Ctrl Pts',(-4.79062346986519,51.9212040079278,-3.69387663272464));
#6140=CARTESIAN_POINT('Ctrl Pts',(-5.58471546251296,51.9408720126469,-2.33549340740676));
#6141=CARTESIAN_POINT('Ctrl Pts',(-5.84660368323659,51.9508096095341,-1.56869876406795));
#6142=CARTESIAN_POINT('Ctrl Pts',(-6.04798129306953,51.9688448860489,-0.0189367011938789));
#6143=CARTESIAN_POINT('Ctrl Pts',(-6.00169394412353,51.9768266635303,0.747068330761391));
#6144=CARTESIAN_POINT('Ctrl Pts',(-5.62060806043904,51.9953697397694,2.23998430255282));
#6145=CARTESIAN_POINT('Ctrl Pts',(-5.28200909226598,52.0051843078803,2.95112506365597));
#6146=CARTESIAN_POINT('Ctrl Pts',(-4.343264457766,52.0247340310338,4.21506666426781));
#6147=CARTESIAN_POINT('Ctrl Pts',(-3.74781747966786,52.034271595978,4.75232770124426));
#6148=CARTESIAN_POINT('Ctrl Pts',(-2.4114876533685,52.0512199102857,5.54641552876093));
#6149=CARTESIAN_POINT('Ctrl Pts',(-1.68999863519737,52.0601250158311,5.80705970867361));
#6150=CARTESIAN_POINT('Ctrl Pts',(-0.15927307289999,52.0792590853598,6.0496282649839));
#6151=CARTESIAN_POINT('Ctrl Pts',(0.637312705374822,52.0892164075882,6.0180732298212));
#6152=CARTESIAN_POINT('Ctrl Pts',(2.16568132834483,52.1083210153754,5.64997174584619));
#6153=CARTESIAN_POINT('Ctrl Pts',(2.88330762224981,52.1166835593658,5.3196695424997));
#6154=CARTESIAN_POINT('Ctrl Pts',(4.14018966352825,52.1343841958284,4.4102159711343));
#6155=CARTESIAN_POINT('Ctrl Pts',(4.67069267170621,52.1438300751988,3.84392906614758));
#6156=CARTESIAN_POINT('Ctrl Pts',(5.5053081025277,52.1634206138229,2.51609807009338));
#6157=CARTESIAN_POINT('Ctrl Pts',(5.79121623205391,52.1733821090614,1.76096369244842));
#6158=CARTESIAN_POINT('Ctrl Pts',(6.04438646328482,52.1916578530666,0.218890678232439));
#6159=CARTESIAN_POINT('Ctrl Pts',(6.02320118561849,52.199569438352,-0.55097201213558));
#6160=CARTESIAN_POINT('Ctrl Pts',(5.69030954107534,52.2179373780415,-2.05553451942558));
#6161=CARTESIAN_POINT('Ctrl Pts',(5.3762506176683,52.2276889646437,-2.77502549942324));
#6162=CARTESIAN_POINT('Ctrl Pts',(4.48163229301664,52.2472735675887,-4.06766549402191));
#6163=CARTESIAN_POINT('Ctrl Pts',(3.90436395250857,52.2569104487973,-4.62459641582749));
#6164=CARTESIAN_POINT('Ctrl Pts',(2.59634506972209,52.2741521285476,-5.46212951296211));
#6165=CARTESIAN_POINT('Ctrl Pts',(1.88539609253017,52.2826825476144,-5.74640518100851));
#6166=CARTESIAN_POINT('Ctrl Pts',(0.763696519234804,52.2967037922806,-5.96355220594268));
#6167=CARTESIAN_POINT('Ctrl Pts',(0.38182666544753,52.3014771654529,-6.));
#6168=CARTESIAN_POINT('Ctrl Pts',(7.37604421985338E-14,52.306249998771,
-6.));
#6169=CARTESIAN_POINT('Origin',(0.,50.,0.));
#6170=CARTESIAN_POINT('',(-7.36700326531062E-15,52.8125,-6.));
#6171=CARTESIAN_POINT('',(3.06147672412016E-14,52.756249998771,-6.));
#6172=CARTESIAN_POINT('',(-7.34788079488412E-16,50.,-6.));
#6173=CARTESIAN_POINT('Ctrl Pts',(-1.14491749414469E-14,52.8125,-6.));
#6174=CARTESIAN_POINT('Ctrl Pts',(0.359533066415523,52.8080058366698,-6.));
#6175=CARTESIAN_POINT('Ctrl Pts',(0.719194283200083,52.80351007146,-5.96768432091232));
#6176=CARTESIAN_POINT('Ctrl Pts',(1.8215255466804,52.7897309306665,-5.76701278626887));
#6177=CARTESIAN_POINT('Ctrl Pts',(2.53589293275615,52.7810870945708,-5.49050179274652));
#6178=CARTESIAN_POINT('Ctrl Pts',(3.8532806219589,52.763941337833,-4.66723876685205));
#6179=CARTESIAN_POINT('Ctrl Pts',(4.43661013077627,52.7543359567424,-4.11671711846622));
#6180=CARTESIAN_POINT('Ctrl Pts',(5.34585807446428,52.7347604020581,-2.83335938087136));
#6181=CARTESIAN_POINT('Ctrl Pts',(5.66801918759594,52.7249869640751,-2.11652765819008));
#6182=CARTESIAN_POINT('Ctrl Pts',(6.01679524895255,52.7065607918979,-0.615756736438865));
#6183=CARTESIAN_POINT('Ctrl Pts',(6.04629083677593,52.6986352802673,0.152793435874327));
#6184=CARTESIAN_POINT('Ctrl Pts',(5.81026625134235,52.6804384052797,1.69747988554611));
#6185=CARTESIAN_POINT('Ctrl Pts',(5.53226434062804,52.6704836463375,2.4565566483534));
#6186=CARTESIAN_POINT('Ctrl Pts',(4.71095261061875,52.650865278049,3.79463933393641));
#6187=CARTESIAN_POINT('Ctrl Pts',(4.18585693462298,52.6413870859433,4.36703308622835));
#6188=CARTESIAN_POINT('Ctrl Pts',(2.93964037161027,52.6236241371035,5.2884005451934));
#6189=CARTESIAN_POINT('Ctrl Pts',(2.22782920664847,52.6153478650831,5.6254289134476));
#6190=CARTESIAN_POINT('Ctrl Pts',(0.705184014040115,52.5963148001755,6.01061589201909));
#6191=CARTESIAN_POINT('Ctrl Pts',(-0.0919183126728877,52.5863510210915,
6.0511433036594));
#6192=CARTESIAN_POINT('Ctrl Pts',(-1.62680507903547,52.567164936512,5.82517162440524));
#6193=CARTESIAN_POINT('Ctrl Pts',(-2.35175733075434,52.558121280367,5.57210108808757));
#6194=CARTESIAN_POINT('Ctrl Pts',(-3.69702974916344,52.5412677989699,4.79193655757096));
#6195=CARTESIAN_POINT('Ctrl Pts',(-4.29812828883109,52.5317641831702,4.26107453881697));
#6196=CARTESIAN_POINT('Ctrl Pts',(-5.25074960954657,52.5122302217109,3.00660064967072));
#6197=CARTESIAN_POINT('Ctrl Pts',(-5.59713037946457,52.5023976972256,2.29829397508418));
#6198=CARTESIAN_POINT('Ctrl Pts',(-5.99355862748471,52.4837998524007,0.809176616231353));
#6199=CARTESIAN_POINT('Ctrl Pts',(-6.04777158221044,52.4757783631922,0.0443211759275311));
#6200=CARTESIAN_POINT('Ctrl Pts',(-5.86375666606749,52.4579190949642,-1.49920629374432));
#6201=CARTESIAN_POINT('Ctrl Pts',(-5.61392726074293,52.4481039489542,-2.26165156988438));
#6202=CARTESIAN_POINT('Ctrl Pts',(-4.84273245148255,52.4285196980954,-3.62551764000003));
#6203=CARTESIAN_POINT('Ctrl Pts',(-4.33635602695557,52.4189398292719,-4.21811145002904));
#6204=CARTESIAN_POINT('Ctrl Pts',(-3.12614981265986,52.4009710618933,-5.17928219571708));
#6205=CARTESIAN_POINT('Ctrl Pts',(-2.43344099399138,52.3929180124248,-5.53860495466283));
#6206=CARTESIAN_POINT('Ctrl Pts',(-1.14120183459968,52.3767650229324,-5.91834520388219));
#6207=CARTESIAN_POINT('Ctrl Pts',(-0.571484748699384,52.3696435593587,-6.));
#6208=CARTESIAN_POINT('Ctrl Pts',(-1.346145417358E-14,52.3625,-6.));
#6209=CARTESIAN_POINT('Ctrl Pts',(7.28583859910259E-14,52.306249998771,
-6.));
#6210=CARTESIAN_POINT('Ctrl Pts',(-0.401217509922084,52.311265217645,-6.));
#6211=CARTESIAN_POINT('Ctrl Pts',(-0.802387333529942,52.3162798404401,-5.95975596723063));
#6212=CARTESIAN_POINT('Ctrl Pts',(-1.97205889691975,52.3309007349825,-5.72153419859104));
#6213=CARTESIAN_POINT('Ctrl Pts',(-2.70793242061734,52.3395856471272,-5.41221345393983));
#6214=CARTESIAN_POINT('Ctrl Pts',(-3.99745874815731,52.357091658676,-4.53958574945196));
#6215=CARTESIAN_POINT('Ctrl Pts',(-4.54410268846408,52.3664324944465,-3.99232132808627));
#6216=CARTESIAN_POINT('Ctrl Pts',(-5.41872646934361,52.3859244514314,-2.69669574545852));
#6217=CARTESIAN_POINT('Ctrl Pts',(-5.72853914181933,52.3958993209595,-1.9541271981608));
#6218=CARTESIAN_POINT('Ctrl Pts',(-6.03420119206698,52.4144117900263,-0.420492625292152));
#6219=CARTESIAN_POINT('Ctrl Pts',(-6.03849055947503,52.4223372120036,0.353595098947635));
#6220=CARTESIAN_POINT('Ctrl Pts',(-5.75381166082129,52.4405254457877,1.86939272759775));
#6221=CARTESIAN_POINT('Ctrl Pts',(-5.46440411634469,52.4502042499875,2.59639283751682));
#6222=CARTESIAN_POINT('Ctrl Pts',(-4.61465836409539,52.4698016634787,3.91612341143982));
#6223=CARTESIAN_POINT('Ctrl Pts',(-4.05618452379599,52.4795266716281,4.49204616107717));
#6224=CARTESIAN_POINT('Ctrl Pts',(-2.77683975502757,52.497054749469,5.37259058801151));
#6225=CARTESIAN_POINT('Ctrl Pts',(-2.07594967199261,52.5053006278711,5.68031825937686));
#6226=CARTESIAN_POINT('Ctrl Pts',(-0.571917507210461,52.5241010299309,6.02393082527088));
#6227=CARTESIAN_POINT('Ctrl Pts',(0.219371708102146,52.5339921451223,6.04704111370116));
#6228=CARTESIAN_POINT('Ctrl Pts',(1.78108360664636,52.5535135438541,5.78505138986634));
#6229=CARTESIAN_POINT('Ctrl Pts',(2.53515315850362,52.562592820824,5.4965487088559));
#6230=CARTESIAN_POINT('Ctrl Pts',(3.8560955030445,52.5799058428859,4.65988665539933));
#6231=CARTESIAN_POINT('Ctrl Pts',(4.41766562552434,52.5891370029495,4.13137127715813));
#6232=CARTESIAN_POINT('Ctrl Pts',(5.32972038187516,52.608515162003,2.86786868089532));
#6233=CARTESIAN_POINT('Ctrl Pts',(5.66208377876122,52.6184925812019,2.13808427191512));
#6234=CARTESIAN_POINT('Ctrl Pts',(6.01827497941694,52.6372258350133,0.613227496568188));
#6235=CARTESIAN_POINT('Ctrl Pts',(6.04718023195906,52.645243444225,-0.165198101203844));
#6236=CARTESIAN_POINT('Ctrl Pts',(5.80834075949411,52.6632568393674,-1.69131023299971));
#6237=CARTESIAN_POINT('Ctrl Pts',(5.54241375424038,52.6728576602113,-2.42466304471854));
#6238=CARTESIAN_POINT('Ctrl Pts',(4.7359041402153,52.6924470131212,-3.76861141008304));
#6239=CARTESIAN_POINT('Ctrl Pts',(4.19581736148071,52.702245316489,-4.36192065691855));
#6240=CARTESIAN_POINT('Ctrl Pts',(2.94408217595834,52.7200388305593,-5.28292543273532));
#6241=CARTESIAN_POINT('Ctrl Pts',(2.25234473625959,52.7280956895677,-5.61283098815292));
#6242=CARTESIAN_POINT('Ctrl Pts',(1.0209991201595,52.743487509769,-5.93471981245366));
#6243=CARTESIAN_POINT('Ctrl Pts',(0.510986821982903,52.7498626634962,-6.));
#6244=CARTESIAN_POINT('Ctrl Pts',(7.2997163869104E-14,52.756249998771,-6.));
#6245=CARTESIAN_POINT('Origin',(0.,50.,0.));
#6246=CARTESIAN_POINT('',(2.09176630104912E-14,53.2625,-6.));
#6247=CARTESIAN_POINT('',(-1.5563571689301E-14,53.206249998771,-6.));
#6248=CARTESIAN_POINT('',(-7.34788079488412E-16,50.,-6.));
#6249=CARTESIAN_POINT('Ctrl Pts',(3.24740234702858E-14,53.2625,-6.));
#6250=CARTESIAN_POINT('Ctrl Pts',(0.491259043487322,53.2563592619564,-6.));
#6251=CARTESIAN_POINT('Ctrl Pts',(0.981766247124528,53.2502279219108,-5.93966359261672));
#6252=CARTESIAN_POINT('Ctrl Pts',(2.19668792147501,53.2350414009815,-5.63479303766205));
#6253=CARTESIAN_POINT('Ctrl Pts',(2.89129907909015,53.2269328223526,-5.31194039765924));
#6254=CARTESIAN_POINT('Ctrl Pts',(4.15186450833354,53.2092230921359,-4.40377338630185));
#6255=CARTESIAN_POINT('Ctrl Pts',(4.69785860830518,53.1994470176055,-3.81592814502068));
#6256=CARTESIAN_POINT('Ctrl Pts',(5.51819126018113,53.179852975433,-2.47952733875372));
#6257=CARTESIAN_POINT('Ctrl Pts',(5.7915971879248,53.1702264099798,-1.7481142998087));
#6258=CARTESIAN_POINT('Ctrl Pts',(6.0450345184174,53.1521569235255,-0.225248751831639));
#6259=CARTESIAN_POINT('Ctrl Pts',(6.02401353226849,53.1441770784285,0.551762673190608));
#6260=CARTESIAN_POINT('Ctrl Pts',(5.68397847418228,53.1255136325642,2.07949861987119));
#6261=CARTESIAN_POINT('Ctrl Pts',(5.35877402192933,53.1155359284412,2.81344256764828));
#6262=CARTESIAN_POINT('Ctrl Pts',(4.45856813278751,53.0961193811304,4.08733226587911));
#6263=CARTESIAN_POINT('Ctrl Pts',(3.90170372579822,53.0868522527771,4.62188709850326));
#6264=CARTESIAN_POINT('Ctrl Pts',(2.59080580140653,53.0694769081903,5.47010540888669));
#6265=CARTESIAN_POINT('Ctrl Pts',(1.8426212209098,53.0605327652614,5.76533605389533));
#6266=CARTESIAN_POINT('Ctrl Pts',(0.286002065858915,53.0410750258232,6.0443673733577));
#6267=CARTESIAN_POINT('Ctrl Pts',(-0.506373489856741,53.0311703313768,6.02990557948782));
#6268=CARTESIAN_POINT('Ctrl Pts',(-2.0147821178542,53.0123152235268,5.70229239415533));
#6269=CARTESIAN_POINT('Ctrl Pts',(-2.71887969344214,53.0039869282711,5.40214419572939));
#6270=CARTESIAN_POINT('Ctrl Pts',(-4.00755213287817,52.9865508222372,4.53548109357146));
#6271=CARTESIAN_POINT('Ctrl Pts',(-4.57217721013319,52.976853122684,3.96563242230801));
#6272=CARTESIAN_POINT('Ctrl Pts',(-5.43653040942714,52.9572574539994,2.65449664019689));
#6273=CARTESIAN_POINT('Ctrl Pts',(-5.73393036442243,52.9475540224996,1.92983597811397));
#6274=CARTESIAN_POINT('Ctrl Pts',(-6.03422559788778,52.92930710304,0.417633294090379));
#6275=CARTESIAN_POINT('Ctrl Pts',(-6.03823131639805,52.9213954490686,-0.355047012897759));
#6276=CARTESIAN_POINT('Ctrl Pts',(-5.7496456227951,52.9029591903323,-1.89150061609016));
#6277=CARTESIAN_POINT('Ctrl Pts',(-5.44755803633235,52.8929874716582,-2.63823818045737));
#6278=CARTESIAN_POINT('Ctrl Pts',(-4.58582734675404,52.8734612376909,-3.94447396481805));
#6279=CARTESIAN_POINT('Ctrl Pts',(-4.04436465632552,52.8640852249845,-4.49797928833948));
#6280=CARTESIAN_POINT('Ctrl Pts',(-2.76545682823853,52.8465152547828,-5.38264583361932));
#6281=CARTESIAN_POINT('Ctrl Pts',(-2.03559289492947,52.8379449111866,-5.69885985218059));
#6282=CARTESIAN_POINT('Ctrl Pts',(-0.848661435065352,52.8231082679383,-5.95496633313774));
#6283=CARTESIAN_POINT('Ctrl Pts',(-0.424420007751195,52.8178052500969,-6.));
#6284=CARTESIAN_POINT('Ctrl Pts',(-1.56819002228303E-14,52.8125,-6.));
#6285=CARTESIAN_POINT('Ctrl Pts',(7.72992780895265E-14,52.756249998771,
-6.));
#6286=CARTESIAN_POINT('Ctrl Pts',(-0.267344232452943,52.7595918016766,-6.));
#6287=CARTESIAN_POINT('Ctrl Pts',(-0.534955221209766,52.7629369390361,-5.98213223044391));
#6288=CARTESIAN_POINT('Ctrl Pts',(-1.58812837821419,52.7761016034986,-5.84025745575398));
#6289=CARTESIAN_POINT('Ctrl Pts',(-2.34637786610327,52.7855204317038,-5.57899834959854));
#6290=CARTESIAN_POINT('Ctrl Pts',(-3.68892829615446,52.8024212061836,-4.79289353052493));
#6291=CARTESIAN_POINT('Ctrl Pts',(-4.26690007172733,52.8115160543365,-4.28643960604275));
#6292=CARTESIAN_POINT('Ctrl Pts',(-5.22063299391897,52.8307406542347,-3.06118509720213));
#6293=CARTESIAN_POINT('Ctrl Pts',(-5.57833851506736,52.8407085219569,-2.34691429810463));
#6294=CARTESIAN_POINT('Ctrl Pts',(-5.99267030213188,52.8596865961856,-0.833009464551543));
#6295=CARTESIAN_POINT('Ctrl Pts',(-6.05008800103878,52.8679032121247,-0.049304478823019));
#6296=CARTESIAN_POINT('Ctrl Pts',(-5.86334588471578,52.8857133464227,1.48810964304889));
#6297=CARTESIAN_POINT('Ctrl Pts',(-5.62409129279005,52.8952155505298,2.22775195585791));
#6298=CARTESIAN_POINT('Ctrl Pts',(-4.8641123352457,52.9148537207022,3.60307435380763));
#6299=CARTESIAN_POINT('Ctrl Pts',(-4.34013798093304,52.924802550029,4.2195911056831));
#6300=CARTESIAN_POINT('Ctrl Pts',(-3.11217506016,52.9429386857438,5.18597083674231));
#6301=CARTESIAN_POINT('Ctrl Pts',(-2.42951782408877,52.9508810259699,5.53871589289677));
#6302=CARTESIAN_POINT('Ctrl Pts',(-0.951878889039818,52.969351512658,5.97503535140572));
#6303=CARTESIAN_POINT('Ctrl Pts',(-0.168721490538011,52.9791409801393,6.04802840329404));
#6304=CARTESIAN_POINT('Ctrl Pts',(1.39663754809634,52.9987079681222,5.88899170824065));
#6305=CARTESIAN_POINT('Ctrl Pts',(2.16306991931943,53.0082883727625,5.65260725548448));
#6306=CARTESIAN_POINT('Ctrl Pts',(3.52880528145598,53.0253600647892,4.91166095187723));
#6307=CARTESIAN_POINT('Ctrl Pts',(4.12161405681198,53.0340975560578,4.42596998738146));
#6308=CARTESIAN_POINT('Ctrl Pts',(5.11296433136239,53.0531628596175,3.23714903247618));
#6309=CARTESIAN_POINT('Ctrl Pts',(5.49361928798084,53.0631099451367,2.5380478737987));
#6310=CARTESIAN_POINT('Ctrl Pts',(5.96202876101701,53.0823062579866,1.03520478653231));
#6311=CARTESIAN_POINT('Ctrl Pts',(6.0462161597879,53.0907942131497,0.246360867567393));
#6312=CARTESIAN_POINT('Ctrl Pts',(5.90735816387129,53.1084133504039,-1.30105561296681));
#6313=CARTESIAN_POINT('Ctrl Pts',(5.69254643262476,53.1178159762678,-2.04561137388686));
#6314=CARTESIAN_POINT('Ctrl Pts',(4.98008915095325,53.1373673273797,-3.44035042292738));
#6315=CARTESIAN_POINT('Ctrl Pts',(4.4786734245861,53.1473358060219,-4.07170653072655));
#6316=CARTESIAN_POINT('Ctrl Pts',(3.28388714913542,53.1657124321822,-5.07945636264507));
#6317=CARTESIAN_POINT('Ctrl Pts',(2.61043683240265,53.1736195383659,-5.45622691503375));
#6318=CARTESIAN_POINT('Ctrl Pts',(1.27568996261008,53.1903038742384,-5.89777164064974));
#6319=CARTESIAN_POINT('Ctrl Pts',(0.639437262180362,53.1982570329937,-6.00000000000001));
#6320=CARTESIAN_POINT('Ctrl Pts',(-4.08006961549745E-14,53.206249998771,
-6.));
#6321=CARTESIAN_POINT('Origin',(0.,50.,0.));
#6322=CARTESIAN_POINT('',(-5.50217552863555E-15,53.7125,-6.));
#6323=CARTESIAN_POINT('',(2.29472894773841E-14,53.656249998771,-6.));
#6324=CARTESIAN_POINT('',(-7.34788079488412E-16,50.,-6.));
#6325=CARTESIAN_POINT('Ctrl Pts',(-2.47024622979097E-14,53.7125,-6.));
#6326=CARTESIAN_POINT('Ctrl Pts',(0.618074665760965,53.704774066678,-6.));
#6327=CARTESIAN_POINT('Ctrl Pts',(1.23343403762461,53.6970820745296,-5.90448815830154));
#6328=CARTESIAN_POINT('Ctrl Pts',(2.55144973118435,53.6806068783601,-5.48389513563829));
#6329=CARTESIAN_POINT('Ctrl Pts',(3.22789828178359,53.6726976087109,-5.11504376016517));
#6330=CARTESIAN_POINT('Ctrl Pts',(4.43365342683385,53.6543992725919,-4.12085893228748));
#6331=CARTESIAN_POINT('Ctrl Pts',(4.94253298882412,53.6444360521858,-3.49429780703739));
#6332=CARTESIAN_POINT('Ctrl Pts',(5.67067377046189,53.6248539348408,-2.10577156805253));
#6333=CARTESIAN_POINT('Ctrl Pts',(5.89353510406379,53.6154175520843,-1.36274491905413));
#6334=CARTESIAN_POINT('Ctrl Pts',(6.04818455072785,53.597734988601,0.181413427204201));
#6335=CARTESIAN_POINT('Ctrl Pts',(5.97288847797361,53.5893458516483,0.968535222468236));
#6336=CARTESIAN_POINT('Ctrl Pts',(5.52237838947031,53.5702207243553,2.47513668414208));
#6337=CARTESIAN_POINT('Ctrl Pts',(5.14925095887713,53.5602654979815,3.17933588192937));
#6338=CARTESIAN_POINT('Ctrl Pts',(4.17027238796539,53.5411466073777,4.38024980235338));
#6339=CARTESIAN_POINT('Ctrl Pts',(3.58240017105194,53.532280002138,4.87279497735445));
#6340=CARTESIAN_POINT('Ctrl Pts',(2.22434107147549,53.5153042633933,5.62877258078118));
#6341=CARTESIAN_POINT('Ctrl Pts',(1.46056358190155,53.5057570447737,5.87345782879563));
#6342=CARTESIAN_POINT('Ctrl Pts',(-0.103746845680585,53.4862031644289,6.04959757139315));
#6343=CARTESIAN_POINT('Ctrl Pts',(-0.888479643857466,53.4763940044517,5.9848979741683));
#6344=CARTESIAN_POINT('Ctrl Pts',(-2.37064544174391,53.4578669319781,5.56406189814694));
#6345=CARTESIAN_POINT('Ctrl Pts',(-3.05631021084422,53.44989513097,5.21897575207413));
#6346=CARTESIAN_POINT('Ctrl Pts',(-4.29478343013108,53.4318374710426,4.26591342741277));
#6347=CARTESIAN_POINT('Ctrl Pts',(-4.82588893847439,53.4218972343699,3.65430760460912));
#6348=CARTESIAN_POINT('Ctrl Pts',(-5.60096633355719,53.4022355275788,2.28552807393122));
#6349=CARTESIAN_POINT('Ctrl Pts',(-5.84801981564352,53.3927033962653,1.54762389555455));
#6350=CARTESIAN_POINT('Ctrl Pts',(-6.05000568544818,53.3748332940483,0.0134711597906734));
#6351=CARTESIAN_POINT('Ctrl Pts',(-6.00099388817791,53.3666852976059,-0.768653128073082));
#6352=CARTESIAN_POINT('Ctrl Pts',(-5.6037508550172,53.3477781178544,-2.28587520700342));
#6353=CARTESIAN_POINT('Ctrl Pts',(-5.2534239545714,53.3378060616091,-3.0047929739411));
#6354=CARTESIAN_POINT('Ctrl Pts',(-4.31178217448903,53.3185338396968,-4.24142744016629));
#6355=CARTESIAN_POINT('Ctrl Pts',(-3.73854364388895,53.3093978219124,-4.7544171925566));
#6356=CARTESIAN_POINT('Ctrl Pts',(-2.40339227005806,53.2923899449371,-5.55468756347263));
#6357=CARTESIAN_POINT('Ctrl Pts',(-1.64777511202965,53.2830971889003,-5.82372103007885));
#6358=CARTESIAN_POINT('Ctrl Pts',(-0.575720817653312,53.2696965102206,-5.97930315353356));
#6359=CARTESIAN_POINT('Ctrl Pts',(-0.287731450645414,53.2660966431331,-6.));
#6360=CARTESIAN_POINT('Ctrl Pts',(3.35148575558719E-14,53.2625,-6.));
#6361=CARTESIAN_POINT('Ctrl Pts',(-4.25007251614318E-14,53.206249998771,
-6.));
#6362=CARTESIAN_POINT('Ctrl Pts',(-0.135125960113356,53.2079390732724,-6.));
#6363=CARTESIAN_POINT('Ctrl Pts',(-0.270394130633584,53.2096299254039,-5.99543532220098));
#6364=CARTESIAN_POINT('Ctrl Pts',(-1.19811557297958,53.2212264434332,-5.93258149174789));
#6365=CARTESIAN_POINT('Ctrl Pts',(-1.9721655079933,53.2309020676209,-5.72202636460942));
#6366=CARTESIAN_POINT('Ctrl Pts',(-3.36128493091421,53.2482660604074,-5.02765194059061));
#6367=CARTESIAN_POINT('Ctrl Pts',(-3.96941649553547,53.2566649403245,-4.5628141001609));
#6368=CARTESIAN_POINT('Ctrl Pts',(-4.99817162713518,53.2755624759913,-3.41108658364329));
#6369=CARTESIAN_POINT('Ctrl Pts',(-5.40139887038662,53.2854770039046,-2.72802508353873));
#6370=CARTESIAN_POINT('Ctrl Pts',(-5.92451595308842,53.3048841619358,-1.23729040588996));
#6371=CARTESIAN_POINT('Ctrl Pts',(-6.03609454420458,53.3137279541916,-0.443077411548285));
#6372=CARTESIAN_POINT('Ctrl Pts',(-5.945170224019,53.3311519300301,1.11398535022657));
#6373=CARTESIAN_POINT('Ctrl Pts',(-5.7547002884681,53.3404467684839,1.86263787900088));
#6374=CARTESIAN_POINT('Ctrl Pts',(-5.08986823307635,53.359892202276,3.27508914235736));
#6375=CARTESIAN_POINT('Ctrl Pts',(-4.61122888937136,53.3698694038797,3.92040099349111));
#6376=CARTESIAN_POINT('Ctrl Pts',(-3.44991154057133,53.3884773944313,4.96884664619351));
#6377=CARTESIAN_POINT('Ctrl Pts',(-2.78536159854707,53.3964329787891,5.36964488468559));
#6378=CARTESIAN_POINT('Ctrl Pts',(-1.33628151113567,53.4145464798818,5.90031898118643));
#6379=CARTESIAN_POINT('Ctrl Pts',(-0.564577998719876,53.4241927737871,6.0233423886157));
#6380=CARTESIAN_POINT('Ctrl Pts',(1.00312974829782,53.4437891206248,5.96865836317032));
#6381=CARTESIAN_POINT('Ctrl Pts',(1.78375291069941,53.4535469101548,5.78354509277361));
#6382=CARTESIAN_POINT('Ctrl Pts',(3.19519965664455,53.4711899944791,5.13484739601032));
#6383=CARTESIAN_POINT('Ctrl Pts',(3.81842392657344,53.4793449766578,4.68994756343085));
#6384=CARTESIAN_POINT('Ctrl Pts',(4.88256744925791,53.4980760320153,3.57403033625501));
#6385=CARTESIAN_POINT('Ctrl Pts',(5.30683580462029,53.5079485253874,2.90699991247375));
#6386=CARTESIAN_POINT('Ctrl Pts',(5.8792561253982,53.5274379477346,1.43713122060551));
#6387=CARTESIAN_POINT('Ctrl Pts',(6.01766909512581,53.5366354886232,0.647009039018205));
#6388=CARTESIAN_POINT('Ctrl Pts',(5.97949354956766,53.5537273034523,-0.909824522287626));
#6389=CARTESIAN_POINT('Ctrl Pts',(5.81547375410483,53.562895375946,-1.66203790876649));
#6390=CARTESIAN_POINT('Ctrl Pts',(5.20272810110748,53.5822039590112,-3.09191954192257));
#6391=CARTESIAN_POINT('Ctrl Pts',(4.74918591129041,53.5921785242975,-3.75147770904066));
#6392=CARTESIAN_POINT('Ctrl Pts',(3.62483532752884,53.6110287442997,-4.8436423316542));
#6393=CARTESIAN_POINT('Ctrl Pts',(2.96974381172352,53.6191282011245,-5.27076083695245));
#6394=CARTESIAN_POINT('Ctrl Pts',(1.53633499263769,53.6370458113631,-5.85107641045857));
#6395=CARTESIAN_POINT('Ctrl Pts',(0.771906526198351,53.6466011671936,-5.99996400996191));
#6396=CARTESIAN_POINT('Ctrl Pts',(0.000186533161219277,53.6562476671065,
-5.99999999782549));
#6397=CARTESIAN_POINT('Ctrl Pts',(9.32665259702794E-5,53.6562488329394,
-6.));
#6398=CARTESIAN_POINT('Ctrl Pts',(3.03433030124084E-14,53.656249998771,
-6.));
#6399=CARTESIAN_POINT('Origin',(0.,50.,0.));
#6400=CARTESIAN_POINT('',(1.71880075371411E-14,54.1625,-6.));
#6401=CARTESIAN_POINT('',(2.22534000869934E-14,54.106249998771,-6.));
#6402=CARTESIAN_POINT('',(-7.34788079488412E-16,50.,-6.));
#6403=CARTESIAN_POINT('Ctrl Pts',(3.40005801291454E-14,54.1625,-6.));
#6404=CARTESIAN_POINT('Ctrl Pts',(0.744020055647716,54.1531997493044,-6.));
#6405=CARTESIAN_POINT('Ctrl Pts',(1.48185695652323,54.1439767880434,-5.86160406932495));
#6406=CARTESIAN_POINT('Ctrl Pts',(2.89541452330477,54.1263073184586,-5.31158997658908));
#6407=CARTESIAN_POINT('Ctrl Pts',(3.55433416718244,54.1182776625721,-4.89521447158238));
#6408=CARTESIAN_POINT('Ctrl Pts',(4.69381032287955,54.0995248539421,-3.82078107911201));
#6409=CARTESIAN_POINT('Ctrl Pts',(5.15760866923583,54.0895477018416,-3.16690534707895));
#6410=CARTESIAN_POINT('Ctrl Pts',(5.79159158877462,54.0701807100565,-1.74388948905437));
#6411=CARTESIAN_POINT('Ctrl Pts',(5.96637457395195,54.0609598476221,-0.993013707211756));
#6412=CARTESIAN_POINT('Ctrl Pts',(6.0262257916751,54.0436645121126,0.570105834070089));
#6413=CARTESIAN_POINT('Ctrl Pts',(5.89655136082426,54.0345455731147,1.36789270390674));
#6414=CARTESIAN_POINT('Ctrl Pts',(5.33768512386391,54.0150063481362,2.85018741973248));
#6415=CARTESIAN_POINT('Ctrl Pts',(4.92007193606728,54.0051192842995,3.52240616815637));
#6416=CARTESIAN_POINT('Ctrl Pts',(3.86718457237685,53.9863344729565,4.64978790699034));
#6417=CARTESIAN_POINT('Ctrl Pts',(3.24882717012052,53.9781103396264,5.10105410207349));
#6418=CARTESIAN_POINT('Ctrl Pts',(1.84450031310309,53.9605562539137,5.7644551725158));
#6419=CARTESIAN_POINT('Ctrl Pts',(1.06589585930534,53.9508236982412,5.9577658430625));
#6420=CARTESIAN_POINT('Ctrl Pts',(-0.501903416108012,53.9312262072986,6.02898893194592));
#6421=CARTESIAN_POINT('Ctrl Pts',(-1.27563304331206,53.9215545869585,5.91382995961615));
#6422=CARTESIAN_POINT('Ctrl Pts',(-2.72935036690895,53.9033831204136,5.39811790017014));
#6423=CARTESIAN_POINT('Ctrl Pts',(-3.39675431349287,53.895452152632,5.00510648807065));
#6424=CARTESIAN_POINT('Ctrl Pts',(-4.56894829391694,53.8769181026692,3.96977080057932));
#6425=CARTESIAN_POINT('Ctrl Pts',(-5.05498728566334,53.8669425468884,3.32888317284369));
#6426=CARTESIAN_POINT('Ctrl Pts',(-5.73525397146423,53.8474607495571,1.92198397764554));
#6427=CARTESIAN_POINT('Ctrl Pts',(-5.93359607726064,53.8381301176553,1.1745699913819));
#6428=CARTESIAN_POINT('Ctrl Pts',(-6.04005597695363,53.8206424541455,-0.379406514454436));
#6429=CARTESIAN_POINT('Ctrl Pts',(-5.93742305258649,53.8119231582694,-1.17185807748706));
#6430=CARTESIAN_POINT('Ctrl Pts',(-5.43209720404327,53.79258343215,-2.66663543577941));
#6431=CARTESIAN_POINT('Ctrl Pts',(-5.03613761430514,53.78265705298,-3.35498768979131));
#6432=CARTESIAN_POINT('Ctrl Pts',(-4.01948150856907,53.7637043156959,-4.51879988913556));
#6433=CARTESIAN_POINT('Ctrl Pts',(-3.41637409273498,53.7552046761591,-4.99040568401792));
#6434=CARTESIAN_POINT('Ctrl Pts',(-2.03484549718193,53.7379355687147,-5.70003249367143));
#6435=CARTESIAN_POINT('Ctrl Pts',(-1.26318875578654,53.7282898594473,-5.91906256818622));
#6436=CARTESIAN_POINT('Ctrl Pts',(-0.314279853539542,53.7164284981692,-5.99383377292694));
#6437=CARTESIAN_POINT('Ctrl Pts',(-0.157052268400006,53.714463153355,-6.));
#6438=CARTESIAN_POINT('Ctrl Pts',(-2.15452655716319E-14,53.7125,-6.));
#6439=CARTESIAN_POINT('Ctrl Pts',(2.62290189567693E-14,53.656249998771,
-6.));
#6440=CARTESIAN_POINT('Ctrl Pts',(-0.802599966653911,53.6662824983541,-6.));
#6441=CARTESIAN_POINT('Ctrl Pts',(-1.59710684431166,53.6762138343249,-5.83895830100868));
#6442=CARTESIAN_POINT('Ctrl Pts',(-3.03657743603123,53.6942072167214,-5.2304033645235));
#6443=CARTESIAN_POINT('Ctrl Pts',(-3.67418475545865,53.7022089655309,-4.80398729501233));
#6444=CARTESIAN_POINT('Ctrl Pts',(-4.77075168658479,53.7207810741442,-3.72147260271503));
#6445=CARTESIAN_POINT('Ctrl Pts',(-5.21396967840967,53.7306052680037,-3.06984447450466));
#6446=CARTESIAN_POINT('Ctrl Pts',(-5.83120699784716,53.7501469341951,-1.62102480927238));
#6447=CARTESIAN_POINT('Ctrl Pts',(-5.99434172267899,53.7596666800625,-0.835814232303809));
#6448=CARTESIAN_POINT('Ctrl Pts',(-6.00513609416499,53.7765649148666,0.718945700488526));
#6449=CARTESIAN_POINT('Ctrl Pts',(-5.86573676047876,53.7855421431641,1.47367493621472));
#6450=CARTESIAN_POINT('Ctrl Pts',(-5.30175469450441,53.8047037726895,2.91813525294736));
#6451=CARTESIAN_POINT('Ctrl Pts',(-4.87188929188569,53.8146646574456,3.59009946627435));
#6452=CARTESIAN_POINT('Ctrl Pts',(-3.78260524830901,53.8337315976273,4.72252951793732));
#6453=CARTESIAN_POINT('Ctrl Pts',(-3.13620136273259,53.8420474817369,5.17441978277654));
#6454=CARTESIAN_POINT('Ctrl Pts',(-1.71751515098164,53.8597810593838,5.80016811140914));
#6455=CARTESIAN_POINT('Ctrl Pts',(-0.960471520801086,53.869244104761,5.97237712439266));
#6456=CARTESIAN_POINT('Ctrl Pts',(0.607967328528821,53.8888495903777,6.02248351713028));
#6457=CARTESIAN_POINT('Ctrl Pts',(1.4046143311556,53.8988076779105,5.88786911885732));
#6458=CARTESIAN_POINT('Ctrl Pts',(2.86335348217455,53.9170419172982,5.32755957371081));
#6459=CARTESIAN_POINT('Ctrl Pts',(3.51668660829516,53.9249597054766,4.92083344100594));
#6460=CARTESIAN_POINT('Ctrl Pts',(4.64732036441513,53.9433583882882,3.87400762861805));
#6461=CARTESIAN_POINT('Ctrl Pts',(5.11004964613728,53.9531216209987,3.23927569860641));
#6462=CARTESIAN_POINT('Ctrl Pts',(5.77412389849353,53.9727017559661,1.81394375589823));
#6463=CARTESIAN_POINT('Ctrl Pts',(5.96328856213595,53.9823221920229,1.03446020983009));
#6464=CARTESIAN_POINT('Ctrl Pts',(6.02562747346526,53.9995134266739,-0.517606635486794));
#6465=CARTESIAN_POINT('Ctrl Pts',(5.91190507370029,54.0081023759522,-1.27495418323414));
#6466=CARTESIAN_POINT('Ctrl Pts',(5.39880069617624,54.0270998861552,-2.73362805348819));
#6467=CARTESIAN_POINT('Ctrl Pts',(4.99393802567096,54.0370350698962,-3.41765344286178));
#6468=CARTESIAN_POINT('Ctrl Pts',(3.94199431913957,54.0563187217668,-4.59166091647857));
#6469=CARTESIAN_POINT('Ctrl Pts',(3.30461752451987,54.0649422797145,-5.06972942274412));
#6470=CARTESIAN_POINT('Ctrl Pts',(1.90144255569312,54.0824819668248,-5.74218208593506));
#6471=CARTESIAN_POINT('Ctrl Pts',(1.152687822376,54.0918414009913,-5.9379654414117));
#6472=CARTESIAN_POINT('Ctrl Pts',(0.258259320259502,54.1030217572678,-5.99583591381765));
#6473=CARTESIAN_POINT('Ctrl Pts',(0.129060583442295,54.1046367414779,-6.));
#6474=CARTESIAN_POINT('Ctrl Pts',(3.04270497686332E-14,54.106249998771,
-6.));
#6475=CARTESIAN_POINT('Origin',(0.,50.,0.));
#6476=CARTESIAN_POINT('',(-2.78454138992168E-14,54.6125,-6.));
#6477=CARTESIAN_POINT('',(9.65930765140174E-15,54.556249998771,-6.));
#6478=CARTESIAN_POINT('',(-7.34788079488412E-16,50.,-6.));
#6479=CARTESIAN_POINT('Ctrl Pts',(-1.90125692967058E-14,54.6125,-6.));
#6480=CARTESIAN_POINT('Ctrl Pts',(0.108463475076468,54.6111442065615,-6.));
#6481=CARTESIAN_POINT('Ctrl Pts',(0.217032411991259,54.6097870948501,-5.99705895880486));
#6482=CARTESIAN_POINT('Ctrl Pts',(1.09210248833924,54.5988487188957,-5.94950343388131));
#6483=CARTESIAN_POINT('Ctrl Pts',(1.84355332705342,54.5894555834118,-5.76112885167375));
#6484=CARTESIAN_POINT('Ctrl Pts',(3.25167517207667,54.571854060349,-5.10344666315784));
#6485=CARTESIAN_POINT('Ctrl Pts',(3.89192160881287,54.5633371643405,-4.63373699445241));
#6486=CARTESIAN_POINT('Ctrl Pts',(4.95581982341022,54.5441213118971,-3.47289450208802));
#6487=CARTESIAN_POINT('Ctrl Pts',(5.36865973088282,54.5341767025107,-2.79260406881144));
#6488=CARTESIAN_POINT('Ctrl Pts',(5.89791975275551,54.5151263660822,-1.33837778648844));
#6489=CARTESIAN_POINT('Ctrl Pts',(6.01980650390735,54.5064230730006,-0.581902777788305));
#6490=CARTESIAN_POINT('Ctrl Pts',(5.97393171253709,54.4893248150252,0.971080814223057));
#6491=CARTESIAN_POINT('Ctrl Pts',(5.7930658586323,54.4797353869317,1.75249128737854));
#6492=CARTESIAN_POINT('Ctrl Pts',(5.14386777267488,54.4601651694279,3.18549585271706));
#6493=CARTESIAN_POINT('Ctrl Pts',(4.68730851567618,54.4503813677914,3.82569012415617));
#6494=CARTESIAN_POINT('Ctrl Pts',(3.567531469532,54.4319267117499,4.8839546464704));
#6495=CARTESIAN_POINT('Ctrl Pts',(2.91928061049845,54.4239910076312,5.29698889009077));
#6496=CARTESIAN_POINT('Ctrl Pts',(1.46664814592476,54.405833101824,5.87284350350165));
#6497=CARTESIAN_POINT('Ctrl Pts',(0.670565922328707,54.3958820740291,6.01595179329487));
#6498=CARTESIAN_POINT('Ctrl Pts',(-0.899932770857932,54.3762508403642,5.98189549108154));
#6499=CARTESIAN_POINT('Ctrl Pts',(-1.65942748180796,54.3667571564773,5.81715281562034));
#6500=CARTESIAN_POINT('Ctrl Pts',(-3.08289154815884,54.348963855648,5.20602692283899));
#6501=CARTESIAN_POINT('Ctrl Pts',(-3.73209849904746,54.3407265244756,4.76218271375655));
#6502=CARTESIAN_POINT('Ctrl Pts',(-4.83280106975809,54.321728751943,3.64273458553758));
#6503=CARTESIAN_POINT('Ctrl Pts',(-5.27035822490241,54.3117622631446,2.97469352834565));
#6504=CARTESIAN_POINT('Ctrl Pts',(-5.85013328313548,54.2925513733541,1.53480083158262));
#6505=CARTESIAN_POINT('Ctrl Pts',(-5.99750082653629,54.2834682218936,0.780817931910112));
#6506=CARTESIAN_POINT('Ctrl Pts',(-6.002542372019,54.2665977363468,-0.774700029943063));
#6507=CARTESIAN_POINT('Ctrl Pts',(-5.84742264239086,54.2571423451884,-1.56152891151443));
#6508=CARTESIAN_POINT('Ctrl Pts',(-5.2446726922113,54.237616080659,-3.01729011869803));
#6509=CARTESIAN_POINT('Ctrl Pts',(-4.80754953397616,54.2277752224983,-3.67397648292641));
#6510=CARTESIAN_POINT('Ctrl Pts',(-3.72147580711357,54.2091510136092,-4.76736224684963));
#6511=CARTESIAN_POINT('Ctrl Pts',(-3.08858384949118,54.2011072981186,-5.19978535068864));
#6512=CARTESIAN_POINT('Ctrl Pts',(-1.66322673748714,54.1832903342185,-5.81935749367896));
#6513=CARTESIAN_POINT('Ctrl Pts',(-0.878877032028892,54.1734859629003,-5.98822219076233));
#6514=CARTESIAN_POINT('Ctrl Pts',(-0.0562965174381724,54.1632037064679,
-5.99980198137835));
#6515=CARTESIAN_POINT('Ctrl Pts',(-0.0281438351033594,54.1628517979388,
-6.));
#6516=CARTESIAN_POINT('Ctrl Pts',(3.00272269393625E-14,54.1625,-6.));
#6517=CARTESIAN_POINT('Ctrl Pts',(3.12250225675825E-14,54.106249998771,
-6.));
#6518=CARTESIAN_POINT('Ctrl Pts',(-0.665995216701814,54.1145749389797,-6.));
#6519=CARTESIAN_POINT('Ctrl Pts',(-1.32831154621538,54.1228538930987,-5.88910260237697));
#6520=CARTESIAN_POINT('Ctrl Pts',(-2.68380168378572,54.1397975198183,-5.42074527927475));
#6521=CARTESIAN_POINT('Ctrl Pts',(-3.35350325734009,54.1477146049907,-5.03401298858342));
#6522=CARTESIAN_POINT('Ctrl Pts',(-4.5181561134759,54.165933691407,-4.02341851709745));
#6523=CARTESIAN_POINT('Ctrl Pts',(-4.99990180303044,54.1756255441917,-3.40625951036384));
#6524=CARTESIAN_POINT('Ctrl Pts',(-5.71022474619925,54.1952223283079,-2.00609127926203));
#6525=CARTESIAN_POINT('Ctrl Pts',(-5.92538144060666,54.2049331533687,-1.2332644606244));
#6526=CARTESIAN_POINT('Ctrl Pts',(-6.03952951974,54.2224130621164,0.315556918500252));
#6527=CARTESIAN_POINT('Ctrl Pts',(-5.95130265594012,54.2307010359501,1.07587410048442));
#6528=CARTESIAN_POINT('Ctrl Pts',(-5.48845800853437,54.2495301726062,2.54801175744083));
#6529=CARTESIAN_POINT('Ctrl Pts',(-5.10861550067973,54.2594285450217,3.24308205985808));
#6530=CARTESIAN_POINT('Ctrl Pts',(-4.09445984153902,54.2789167229654,4.45779978214083));
#6531=CARTESIAN_POINT('Ctrl Pts',(-3.46606168236284,54.2879242277415,4.96215375070386));
#6532=CARTESIAN_POINT('Ctrl Pts',(-2.07840524998668,54.3052699331462,5.68021403610727));
#6533=CARTESIAN_POINT('Ctrl Pts',(-1.33839842906827,54.3145200184076,5.89858218723038));
#6534=CARTESIAN_POINT('Ctrl Pts',(0.213479934968243,54.3339184979581,6.04861227994175));
#6535=CARTESIAN_POINT('Ctrl Pts',(1.01169570619217,54.3438961950984,5.96722408995027));
#6536=CARTESIAN_POINT('Ctrl Pts',(2.50744136059901,54.3625930157785,5.50518764661662));
#6537=CARTESIAN_POINT('Ctrl Pts',(3.19332323280763,54.3705899008775,5.13780476697635));
#6538=CARTESIAN_POINT('Ctrl Pts',(4.39027354821862,54.3886326673574,4.16214498033042));
#6539=CARTESIAN_POINT('Ctrl Pts',(4.88958746882181,54.3982470520664,3.56228519082363));
#6540=CARTESIAN_POINT('Ctrl Pts',(5.64320947287391,54.4178391026293,2.1875529510982));
#6541=CARTESIAN_POINT('Ctrl Pts',(5.88297354086154,54.4276259148414,1.42191381386779));
#6542=CARTESIAN_POINT('Ctrl Pts',(6.04660168590296,54.4453757161804,-0.123271845530199));
#6543=CARTESIAN_POINT('Ctrl Pts',(5.98249839701545,54.4534586343659,-0.88674078467215));
#6544=CARTESIAN_POINT('Ctrl Pts',(5.56684849579367,54.4721244012078,-2.37103488404048));
#6545=CARTESIAN_POINT('Ctrl Pts',(5.21074344315951,54.4819779770023,-3.07567187803633));
#6546=CARTESIAN_POINT('Ctrl Pts',(4.2407625315026,54.5014910036302,-4.31818932579503));
#6547=CARTESIAN_POINT('Ctrl Pts',(3.63254647488505,54.5108431678349,-4.8410110561471));
#6548=CARTESIAN_POINT('Ctrl Pts',(2.2759967354326,54.5278000395781,-5.6036122334027));
#6549=CARTESIAN_POINT('Ctrl Pts',(1.54668082782739,54.5369164884232,-5.84708390728187));
#6550=CARTESIAN_POINT('Ctrl Pts',(0.528449925791234,54.5496443746986,-5.98256511642262));
#6551=CARTESIAN_POINT('Ctrl Pts',(0.264086110120325,54.5529489223944,-6.));
#6552=CARTESIAN_POINT('Ctrl Pts',(2.41473507855972E-14,54.556249998771,
-6.));
#6553=CARTESIAN_POINT('Origin',(0.,50.,0.));
#6554=CARTESIAN_POINT('',(-8.83284460251102E-15,55.0625,-6.));
#6555=CARTESIAN_POINT('',(1.52537908614269E-14,55.006249998771,-6.));
#6556=CARTESIAN_POINT('',(-7.34788079488412E-16,50.,-6.));
#6557=CARTESIAN_POINT('Ctrl Pts',(-3.46944695195361E-14,55.0625,-6.));
#6558=CARTESIAN_POINT('Ctrl Pts',(0.243170996938084,55.0594603625383,-6.));
#6559=CARTESIAN_POINT('Ctrl Pts',(0.486616495026908,55.0564172938121,-5.98521738970615));
#6560=CARTESIAN_POINT('Ctrl Pts',(1.48607170177765,55.0439241037278,-5.86287970427564));
#6561=CARTESIAN_POINT('Ctrl Pts',(2.21859564233351,55.0347675544708,-5.62668817545351));
#6562=CARTESIAN_POINT('Ctrl Pts',(3.583522346217,55.0177059706723,-4.87742638094908));
#6563=CARTESIAN_POINT('Ctrl Pts',(4.19704545643206,55.0084745072065,-4.36070730516347));
#6564=CARTESIAN_POINT('Ctrl Pts',(5.18000952607178,54.9889794757186,-3.12734800698956));
#6565=CARTESIAN_POINT('Ctrl Pts',(5.54341604297027,54.9791111174456,-2.42556096848081));
#6566=CARTESIAN_POINT('Ctrl Pts',(5.9735386696846,54.9603947304027,-0.944946607204173));
#6567=CARTESIAN_POINT('Ctrl Pts',(6.04506231156067,54.9522570672934,-0.182482207805695));
#6568=CARTESIAN_POINT('Ctrl Pts',(5.89669431020368,54.9345898771,1.36388260891157));
#6569=CARTESIAN_POINT('Ctrl Pts',(5.66449374094429,54.9248254128607,2.13182411687757));
#6570=CARTESIAN_POINT('Ctrl Pts',(4.92412965534831,54.9052297552454,3.51454402462014));
#6571=CARTESIAN_POINT('Ctrl Pts',(4.4301701829403,54.8955905211087,4.11979069803384));
#6572=CARTESIAN_POINT('Ctrl Pts',(3.24316152613063,54.8774928793281,5.10625946708773));
#6573=CARTESIAN_POINT('Ctrl Pts',(2.56232823027645,54.8695291028784,5.47964030494605));
#6574=CARTESIAN_POINT('Ctrl Pts',(1.07208496965756,54.8509010621207,5.9567802161547));
#6575=CARTESIAN_POINT('Ctrl Pts',(0.273888437522632,54.840923605469,6.04628594794717));
#6576=CARTESIAN_POINT('Ctrl Pts',(-1.28092368736922,54.8214884539079,5.91142217391699));
#6577=CARTESIAN_POINT('Ctrl Pts',(-2.02371620559728,54.81220354743,5.70002346906044));
#6578=CARTESIAN_POINT('Ctrl Pts',(-3.41623463724428,54.7947970670344,4.99613549809339));
#6579=CARTESIAN_POINT('Ctrl Pts',(-4.04744457912879,54.7859176942241,4.50002714754593));
#6580=CARTESIAN_POINT('Ctrl Pts',(-5.07348642469305,54.7664922480945,3.29796683495025));
#6581=CARTESIAN_POINT('Ctrl Pts',(-5.46116494334903,54.7565811802079,2.60624789808891));
#6582=CARTESIAN_POINT('Ctrl Pts',(-5.93968782386747,54.7376988813085,1.13825115557217));
#6583=CARTESIAN_POINT('Ctrl Pts',(-6.03588614738751,54.7293260283239,0.378902501922215));
#6584=CARTESIAN_POINT('Ctrl Pts',(-5.93799646795637,54.7119360578891,-1.17099752318919));
#6585=CARTESIAN_POINT('Ctrl Pts',(-5.73097417840607,54.7022524150224,-1.94600975911659));
#6586=CARTESIAN_POINT('Ctrl Pts',(-5.03506882783893,54.6826584748905,-3.35423927518282));
#6587=CARTESIAN_POINT('Ctrl Pts',(-4.55922402286184,54.6729431409721,-3.97697425342747));
#6588=CARTESIAN_POINT('Ctrl Pts',(-3.40522375135924,54.6546671349834,-4.99897700239477));
#6589=CARTESIAN_POINT('Ctrl Pts',(-2.74072116488649,54.6467590145611,-5.39200952355117));
#6590=CARTESIAN_POINT('Ctrl Pts',(-1.37124203932091,54.6296405254915,-5.88174277618126));
#6591=CARTESIAN_POINT('Ctrl Pts',(-0.687741080113753,54.6210967635014,-5.99999999999999));
#6592=CARTESIAN_POINT('Ctrl Pts',(-2.33146835171283E-14,54.6125,-6.));
#6593=CARTESIAN_POINT('Ctrl Pts',(2.4980018054066E-14,54.556249998771,-6.));
#6594=CARTESIAN_POINT('Ctrl Pts',(-0.524082563586572,54.5628010308158,-6.));
#6595=CARTESIAN_POINT('Ctrl Pts',(-1.04707144064502,54.5693383917791,-5.93133051383516));
#6596=CARTESIAN_POINT('Ctrl Pts',(-2.30620672576332,54.585077582843,-5.59336178117351));
#6597=CARTESIAN_POINT('Ctrl Pts',(-3.01071206136714,54.593257344516,-5.247846484898));
#6598=CARTESIAN_POINT('Ctrl Pts',(-4.24333742521803,54.6110988001506,-4.31137999639267));
#6599=CARTESIAN_POINT('Ctrl Pts',(-4.76145033958675,54.6206167190358,-3.73128494208711));
#6600=CARTESIAN_POINT('Ctrl Pts',(-5.56565134150618,54.6402674130825,-2.38033724741197));
#6601=CARTESIAN_POINT('Ctrl Pts',(-5.83351432249087,54.6502119037212,-1.61635531603474));
#6602=CARTESIAN_POINT('Ctrl Pts',(-6.04769396257433,54.6683072317106,-0.0684371911720527));
#6603=CARTESIAN_POINT('Ctrl Pts',(-6.00761182676598,54.6762638149825,0.69849130020703));
#6604=CARTESIAN_POINT('Ctrl Pts',(-5.63849769195529,54.6947638196598,2.19434038398171));
#6605=CARTESIAN_POINT('Ctrl Pts',(-5.30598207159103,54.7045636698139,2.90763378097386));
#6606=CARTESIAN_POINT('Ctrl Pts',(-4.37812463732207,54.7241241274613,4.17885271964518));
#6607=CARTESIAN_POINT('Ctrl Pts',(-3.7871338804005,54.7336874036299,4.72106165828979));
#6608=CARTESIAN_POINT('Ctrl Pts',(-2.45780508178541,54.7507092371596,5.52598294584271));
#6609=CARTESIAN_POINT('Ctrl Pts',(-1.73898164930581,54.7595127281547,5.7925185962507));
#6610=CARTESIAN_POINT('Ctrl Pts',(-0.211522394103572,54.7786059688447,6.04793647814097));
#6611=CARTESIAN_POINT('Ctrl Pts',(0.584595403767378,54.7885574413181,6.02333195023259));
#6612=CARTESIAN_POINT('Ctrl Pts',(2.11735082107309,54.8077168840344,5.66852444778916));
#6613=CARTESIAN_POINT('Ctrl Pts',(2.83951320933961,54.8161523731448,5.34345370764666));
#6614=CARTESIAN_POINT('Ctrl Pts',(4.10462434844559,54.8338045050574,4.4432318665157));
#6615=CARTESIAN_POINT('Ctrl Pts',(4.6392550826848,54.8432247738107,3.88169391275978));
#6616=CARTESIAN_POINT('Ctrl Pts',(5.48405859603673,54.8627923630686,2.56186498053673));
#6617=CARTESIAN_POINT('Ctrl Pts',(5.77603544192931,54.8727582598742,1.80982777855984));
#6618=CARTESIAN_POINT('Ctrl Pts',(6.04243628777694,54.8910943519024,0.269818751685842));
#6619=CARTESIAN_POINT('Ctrl Pts',(6.02766608938643,54.8990014361889,-0.501080033249619));
#6620=CARTESIAN_POINT('Ctrl Pts',(5.70698531737599,54.9173242780495,-2.00852653209502));
#6621=CARTESIAN_POINT('Ctrl Pts',(5.39916244932141,54.9270583443147,-2.72999944092045));
#6622=CARTESIAN_POINT('Ctrl Pts',(4.51584446455605,54.9466482719774,-4.02965556615108));
#6623=CARTESIAN_POINT('Ctrl Pts',(3.9432806003685,54.9563085395483,-4.59146295824019));
#6624=CARTESIAN_POINT('Ctrl Pts',(2.64248979487433,54.9736234368491,-5.4399327353421));
#6625=CARTESIAN_POINT('Ctrl Pts',(1.93413273845439,54.9820733395403,-5.7301633782239));
#6626=CARTESIAN_POINT('Ctrl Pts',(0.797703277241862,54.9962787078055,-5.96022548855814));
#6627=CARTESIAN_POINT('Ctrl Pts',(0.398870320543266,55.0012641197642,-6.));
#6628=CARTESIAN_POINT('Ctrl Pts',(3.81639164714898E-14,55.006249998771,
-6.));
#6629=CARTESIAN_POINT('Origin',(0.,50.,0.));
#6630=CARTESIAN_POINT('',(-6.36086364924407E-15,55.5125,-6.));
#6631=CARTESIAN_POINT('',(8.65316803533519E-15,55.456249998771,-6.));
#6632=CARTESIAN_POINT('',(-7.34788079488412E-16,50.,-6.));
#6633=CARTESIAN_POINT('Ctrl Pts',(-3.46250805804971E-14,55.5125,-6.));
#6634=CARTESIAN_POINT('Ctrl Pts',(0.376703946330025,55.5077912006709,-6.));
#6635=CARTESIAN_POINT('Ctrl Pts',(0.753472588888227,55.5030815926389,-5.96452369981927));
#6636=CARTESIAN_POINT('Ctrl Pts',(1.87073150335176,55.4891158562081,-5.75120440797882));
#6637=CARTESIAN_POINT('Ctrl Pts',(2.5824631340013,55.4805601853587,-5.46871532290478));
#6638=CARTESIAN_POINT('Ctrl Pts',(3.89264334169019,55.4633405323271,-4.6344648083913));
#6639=CARTESIAN_POINT('Ctrl Pts',(4.47131370817137,55.4537107987603,-4.07900361752885));
#6640=CARTESIAN_POINT('Ctrl Pts',(5.36930891312379,55.4341280670817,-2.78848612586233));
#6641=CARTESIAN_POINT('Ctrl Pts',(5.68523510906606,55.4243713528467,-2.06959954574193));
#6642=CARTESIAN_POINT('Ctrl Pts',(6.02178549004339,55.4059899565657,-0.565906344247707));
#6643=CARTESIAN_POINT('Ctrl Pts',(6.04488833118811,55.3980759709811,0.203650477614851));
#6644=CARTESIAN_POINT('Ctrl Pts',(5.79567389144728,55.3798183574028,1.74633255200975));
#6645=CARTESIAN_POINT('Ctrl Pts',(5.51158572968284,55.369858312968,2.50238366903789));
#6646=CARTESIAN_POINT('Ctrl Pts',(4.68002966528737,55.3502611620082,3.83259181253258));
#6647=CARTESIAN_POINT('Ctrl Pts',(4.15076842647487,55.3408077395651,4.40029245259052));
#6648=CARTESIAN_POINT('Ctrl Pts',(2.89634695185098,55.3230926721373,5.31249970824152));
#6649=CARTESIAN_POINT('Ctrl Pts',(2.18006863674793,55.3147508579593,5.64435900304111));
#6650=CARTESIAN_POINT('Ctrl Pts',(0.65301674366652,55.2956627092958,6.01641659700119));
#6651=CARTESIAN_POINT('Ctrl Pts',(-0.143697171846589,55.2857037853519,6.05004525969472));
#6652=CARTESIAN_POINT('Ctrl Pts',(-1.67538998151804,55.266557625231,5.81131134918754));
#6653=CARTESIAN_POINT('Ctrl Pts',(-2.39767714231781,55.2576212337002,5.55242057122521));
#6654=CARTESIAN_POINT('Ctrl Pts',(-3.73608308927647,55.2406948435203,4.76155665670778));
#6655=CARTESIAN_POINT('Ctrl Pts',(-4.33284626103593,55.2311650493507,4.22577335789718));
#6656=CARTESIAN_POINT('Ctrl Pts',(-5.27481565079531,55.2116187796453,2.96401258647136));
#6657=CARTESIAN_POINT('Ctrl Pts',(-5.61522017998204,55.2017999578695,2.25352132977259));
#6658=CARTESIAN_POINT('Ctrl Pts',(-5.99986293011047,55.1832441412076,0.761482005930106));
#6659=CARTESIAN_POINT('Ctrl Pts',(-6.04799029994773,55.1752538979774,-0.00425312209671055));
#6660=CARTESIAN_POINT('Ctrl Pts',(-5.85040814233194,55.1572365006543,-1.55455488134153));
#6661=CARTESIAN_POINT('Ctrl Pts',(-5.59029581047135,55.147301071778,-2.32217456232466));
#6662=CARTESIAN_POINT('Ctrl Pts',(-4.79921218024328,55.1276281671419,-3.68274730144777));
#6663=CARTESIAN_POINT('Ctrl Pts',(-4.28647314765261,55.1180811516861,-4.26863279389512));
#6664=CARTESIAN_POINT('Ctrl Pts',(-3.06417633838736,55.1001807055688,-5.21651178354219));
#6665=CARTESIAN_POINT('Ctrl Pts',(-2.36514495870567,55.0920643119838,-5.56841679012325));
#6666=CARTESIAN_POINT('Ctrl Pts',(-1.09060147835293,55.0761325184794,-5.92546814491037));
#6667=CARTESIAN_POINT('Ctrl Pts',(-0.545992672507869,55.0693249084063,-5.99999999999999));
#6668=CARTESIAN_POINT('Ctrl Pts',(-2.55351295663786E-14,55.0625,-6.));
#6669=CARTESIAN_POINT('Ctrl Pts',(2.67147415300428E-14,55.006249998771,
-6.));
#6670=CARTESIAN_POINT('Ctrl Pts',(-0.383498096873053,55.0110437249819,-6.));
#6671=CARTESIAN_POINT('Ctrl Pts',(-0.767030733126266,55.0158378829351,-5.96323238459905));
#6672=CARTESIAN_POINT('Ctrl Pts',(-1.92341860149788,55.0302927312897,-5.73836805133425));
#6673=CARTESIAN_POINT('Ctrl Pts',(-2.66390770238158,55.0390710339514,-5.43433369990439));
#6674=CARTESIAN_POINT('Ctrl Pts',(-3.96150517296733,55.05652800478,-4.57089605970513));
#6675=CARTESIAN_POINT('Ctrl Pts',(-4.51204186370488,55.0658414586601,-4.02840854953488));
#6676=CARTESIAN_POINT('Ctrl Pts',(-5.39638537330542,55.0853059424018,-2.74093252440032));
#6677=CARTESIAN_POINT('Ctrl Pts',(-5.71203585602825,55.0952824329659,-2.0015846935231));
#6678=CARTESIAN_POINT('Ctrl Pts',(-6.03067862274505,55.1138523039486,-0.470141978956567));
#6679=CARTESIAN_POINT('Ctrl Pts',(-6.04128052820748,55.1217941051577,0.305035826766368));
#6680=CARTESIAN_POINT('Ctrl Pts',(-5.76842964141191,55.1399375910254,1.82352872578303));
#6681=CARTESIAN_POINT('Ctrl Pts',(-5.48507891182408,55.1495970803031,2.55224150333299));
#6682=CARTESIAN_POINT('Ctrl Pts',(-4.64644024297387,55.1691942904959,3.87836597494945));
#6683=CARTESIAN_POINT('Ctrl Pts',(-4.09266447021715,55.1789391921554,4.45883883889243));
#6684=CARTESIAN_POINT('Ctrl Pts',(-2.82041073021032,55.1965364144534,5.34986456454548));
#6685=CARTESIAN_POINT('Ctrl Pts',(-2.12191903657733,55.2047260108138,5.66332403510793));
#6686=CARTESIAN_POINT('Ctrl Pts',(-0.621212253847653,55.2234848455979,6.01896338011437));
#6687=CARTESIAN_POINT('Ctrl Pts',(0.169198820019541,55.2333649840212,6.04856958122179));
#6688=CARTESIAN_POINT('Ctrl Pts',(1.73468835005995,55.2529336031467,5.79944910313727));
#6689=CARTESIAN_POINT('Ctrl Pts',(2.4932084072145,55.2621197300586,5.51603414832992));
#6690=CARTESIAN_POINT('Ctrl Pts',(3.82167666488108,55.2793856676905,4.68806665616739));
#6691=CARTESIAN_POINT('Ctrl Pts',(4.38673093219715,55.2885893283747,4.16410313374755));
#6692=CARTESIAN_POINT('Ctrl Pts',(5.30758874303518,55.3079374972146,2.90845336063413));
#6693=CARTESIAN_POINT('Ctrl Pts',(5.64528357279742,55.3179140263612,2.18182927535854));
#6694=CARTESIAN_POINT('Ctrl Pts',(6.01358028789105,55.3366990892299,0.659175706319895));
#6695=CARTESIAN_POINT('Ctrl Pts',(6.04840302459413,55.3447500396245,-0.120325316236857));
#6696=CARTESIAN_POINT('Ctrl Pts',(5.82046622292647,55.3627212936052,-1.64883927418895));
#6697=CARTESIAN_POINT('Ctrl Pts',(5.56012447741785,55.3723023405631,-2.38359010377172));
#6698=CARTESIAN_POINT('Ctrl Pts',(4.76396909667191,55.3918869071758,-3.73307434931714));
#6699=CARTESIAN_POINT('Ctrl Pts',(4.22832460066992,55.4017011341472,-4.3304193087725));
#6700=CARTESIAN_POINT('Ctrl Pts',(2.98320792615936,55.4195567595843,-5.26098288599923));
#6701=CARTESIAN_POINT('Ctrl Pts',(2.29359292232722,55.4275800872419,-5.59615121010581));
#6702=CARTESIAN_POINT('Ctrl Pts',(1.05013028978537,55.4431233701486,-5.93092063589006));
#6703=CARTESIAN_POINT('Ctrl Pts',(0.52564419070393,55.4496794463872,-6.));
#6704=CARTESIAN_POINT('Ctrl Pts',(3.92741394961149E-14,55.456249998771,
-6.));
#6705=CARTESIAN_POINT('Origin',(0.,50.,0.));
#6706=CARTESIAN_POINT('',(4.30578759205125E-16,55.9625,-6.));
#6707=CARTESIAN_POINT('',(-6.33484279710442E-15,55.906249998771,-6.));
#6708=CARTESIAN_POINT('',(-7.34788079488412E-16,50.,-6.));
#6709=CARTESIAN_POINT('Ctrl Pts',(-2.31759056390501E-14,55.9625,-6.));
#6710=CARTESIAN_POINT('Ctrl Pts',(0.506510355492559,55.9561686205563,-6.));
#6711=CARTESIAN_POINT('Ctrl Pts',(1.01209912649085,55.9498487609188,-5.93585868886586));
#6712=CARTESIAN_POINT('Ctrl Pts',(2.23972937663833,55.934503382792,-5.61786356684971));
#6713=CARTESIAN_POINT('Ctrl Pts',(2.93211714923827,55.9264354497199,-5.28956140569632));
#6714=CARTESIAN_POINT('Ctrl Pts',(4.18586379090878,55.9086609288615,-4.37147246239368));
#6715=CARTESIAN_POINT('Ctrl Pts',(4.72729822672339,55.8988675897434,-3.77939986348097));
#6716=CARTESIAN_POINT('Ctrl Pts',(5.53695585424453,55.8792769970504,-2.43715447829796));
#6717=CARTESIAN_POINT('Ctrl Pts',(5.80458380678377,55.8696702471273,-1.70423600408193));
#6718=CARTESIAN_POINT('Ctrl Pts',(6.04674334504191,55.8516440612997,-0.178859160276753));
#6719=CARTESIAN_POINT('Ctrl Pts',(6.01963510658597,55.8436357324319,0.599242189053428));
#6720=CARTESIAN_POINT('Ctrl Pts',(5.66712365275588,55.8249183119528,2.1247608466305));
#6721=CARTESIAN_POINT('Ctrl Pts',(5.33638643972422,55.814940737021,2.85549851929398));
#6722=CARTESIAN_POINT('Ctrl Pts',(4.42702037453283,55.7955536697512,4.12137633788628));
#6723=CARTESIAN_POINT('Ctrl Pts',(3.86651644869223,55.7863142436256,4.65127087115331));
#6724=CARTESIAN_POINT('Ctrl Pts',(2.54786180622585,55.7689869752017,5.49056975257084));
#6725=CARTESIAN_POINT('Ctrl Pts',(1.79513813675954,55.7599392267095,5.78061097099999));
#6726=CARTESIAN_POINT('Ctrl Pts',(0.23458113017717,55.7404322641272,6.04649552222604));
#6727=CARTESIAN_POINT('Ctrl Pts',(-0.556964089759994,55.730537948878,6.02535719121178));
#6728=CARTESIAN_POINT('Ctrl Pts',(-2.06199924228826,55.7117250094714,5.68539383393839));
#6729=CARTESIAN_POINT('Ctrl Pts',(-2.76361918902967,55.7034610872385,5.37939944167112));
#6730=CARTESIAN_POINT('Ctrl Pts',(-4.04510199417962,55.685953988623,4.50202738844765));
#6731=CARTESIAN_POINT('Ctrl Pts',(-4.60498874435356,55.6762351251842,3.927488006763));
#6732=CARTESIAN_POINT('Ctrl Pts',(-5.45808318515566,55.6566379085014,2.60970897944998));
#6733=CARTESIAN_POINT('Ctrl Pts',(-5.74932024339951,55.6469533803752,1.88323638612024));
#6734=CARTESIAN_POINT('Ctrl Pts',(-6.03757286035596,55.628751677179,0.36825779370989));
#6735=CARTESIAN_POINT('Ctrl Pts',(-6.03518566331545,55.620830193446,-0.405504682015357));
#6736=CARTESIAN_POINT('Ctrl Pts',(-5.7334376873049,55.6023351233639,-1.93979179733037));
#6737=CARTESIAN_POINT('Ctrl Pts',(-5.42539117238217,55.5923608738131,-2.68332276511667));
#6738=CARTESIAN_POINT('Ctrl Pts',(-4.55371198609171,55.5728608728174,-3.98139148411494));
#6739=CARTESIAN_POINT('Ctrl Pts',(-4.00824961913072,55.5635118891683,-4.53009075594725));
#6740=CARTESIAN_POINT('Ctrl Pts',(-2.72115707341145,55.545991162172,-5.40548295984068));
#6741=CARTESIAN_POINT('Ctrl Pts',(-1.98666726293254,55.5373333407866,-5.71638974522215));
#6742=CARTESIAN_POINT('Ctrl Pts',(-0.813017784230776,55.5226627223029,-5.95867972578508));
#6743=CARTESIAN_POINT('Ctrl Pts',(-0.406546568500345,55.5175818321062,-6.));
#6744=CARTESIAN_POINT('Ctrl Pts',(-2.43555176027144E-14,55.5125,-6.));
#6745=CARTESIAN_POINT('Ctrl Pts',(3.10862446895044E-14,55.456249998771,
-6.));
#6746=CARTESIAN_POINT('Ctrl Pts',(-0.252210903516962,55.4594026350649,-6.));
#6747=CARTESIAN_POINT('Ctrl Pts',(-0.504688423457114,55.4625586040642,-5.98409784058804));
#6748=CARTESIAN_POINT('Ctrl Pts',(-1.54373724533781,55.4755467143377,-5.85213938017255));
#6749=CARTESIAN_POINT('Ctrl Pts',(-2.30391117524793,55.4850488884616,-5.59666644130015));
#6750=CARTESIAN_POINT('Ctrl Pts',(-3.65187175733235,55.5018983957376,-4.82109477946861));
#6751=CARTESIAN_POINT('Ctrl Pts',(-4.23331191747355,55.5109480403995,-4.31951835605545));
#6752=CARTESIAN_POINT('Ctrl Pts',(-5.1959362139153,55.5301362886266,-3.10275530806472));
#6753=CARTESIAN_POINT('Ctrl Pts',(-5.55907359665902,55.5401003115312,-2.39197576474886));
#6754=CARTESIAN_POINT('Ctrl Pts',(-5.98607499914932,55.5591303586157,-0.880584690310904));
#6755=CARTESIAN_POINT('Ctrl Pts',(-6.04974036764568,55.5674032084568,-0.0956935454188609));
#6756=CARTESIAN_POINT('Ctrl Pts',(-5.87426437626053,55.5851687624621,1.44410692567844));
#6757=CARTESIAN_POINT('Ctrl Pts',(-5.64076913631869,55.594648290711,2.18497969585381));
#6758=CARTESIAN_POINT('Ctrl Pts',(-4.89196010651508,55.6142677812028,3.56502549961348));
#6759=CARTESIAN_POINT('Ctrl Pts',(-4.37327273364698,55.6242222315692,4.18511394105391));
#6760=CARTESIAN_POINT('Ctrl Pts',(-3.1530932458043,55.6424157760385,5.16129063278652));
#6761=CARTESIAN_POINT('Ctrl Pts',(-2.47263399832919,55.6503420737918,5.51969218998909));
#6762=CARTESIAN_POINT('Ctrl Pts',(-0.998344881824021,55.6687706877482,5.96736898710037));
#6763=CARTESIAN_POINT('Ctrl Pts',(-0.216398092781286,55.6785450226112,6.04643284268571));
#6764=CARTESIAN_POINT('Ctrl Pts',(1.34961157525821,55.6981201434617,5.8999504421065));
#6765=CARTESIAN_POINT('Ctrl Pts',(2.11793378939434,55.7077241711384,5.66967751177729));
#6766=CARTESIAN_POINT('Ctrl Pts',(3.4892697862692,55.7248658710993,4.93977576174127));
#6767=CARTESIAN_POINT('Ctrl Pts',(4.08570796533894,55.7335147004569,4.45908148989135));
#6768=CARTESIAN_POINT('Ctrl Pts',(5.08605410587349,55.752540440314,3.27910903892516));
#6769=CARTESIAN_POINT('Ctrl Pts',(5.47216468472763,55.7624807928114,2.58377965513738));
#6770=CARTESIAN_POINT('Ctrl Pts',(5.95365105266994,55.7817284375683,1.08374467820946));
#6771=CARTESIAN_POINT('Ctrl Pts',(6.04435521787812,55.7902941311579,0.293630878490182));
#6772=CARTESIAN_POINT('Ctrl Pts',(5.9169993760804,55.807866799235,-1.25613373511938));
#6773=CARTESIAN_POINT('Ctrl Pts',(5.70804226618502,55.8172442820665,-2.00174704940243));
#6774=CARTESIAN_POINT('Ctrl Pts',(5.00701244719134,55.8367719223822,-3.4008934375671));
#6775=CARTESIAN_POINT('Ctrl Pts',(4.51104662686718,55.8467434818924,-4.03568064847992));
#6776=CARTESIAN_POINT('Ctrl Pts',(3.32426749193355,55.8651764922436,-5.05326195358436));
#6777=CARTESIAN_POINT('Ctrl Pts',(2.65297920336261,55.8730877587289,-5.43579915260006));
#6778=CARTESIAN_POINT('Ctrl Pts',(1.30624861040293,55.8899218911409,-5.89276769691465));
#6779=CARTESIAN_POINT('Ctrl Pts',(0.654900599338993,55.8980637412792,-6.));
#6780=CARTESIAN_POINT('Ctrl Pts',(-1.98452365651747E-14,55.906249998771,
-6.));
#6781=CARTESIAN_POINT('Origin',(0.,50.,0.));
#6782=CARTESIAN_POINT('',(-1.96575190926063E-14,56.4125,-6.));
#6783=CARTESIAN_POINT('',(-4.32256356497133E-15,56.3562499987709,-6.));
#6784=CARTESIAN_POINT('',(-7.34788079488412E-16,50.,-6.));
#6785=CARTESIAN_POINT('Ctrl Pts',(1.59594559789866E-14,56.4125,-6.));
#6786=CARTESIAN_POINT('Ctrl Pts',(0.655375591716446,56.4043078051035,-6.));
#6787=CARTESIAN_POINT('Ctrl Pts',(1.30732882068663,56.3961583897414,-5.89261098724614));
#6788=CARTESIAN_POINT('Ctrl Pts',(2.65590763722434,56.3793011545347,-5.43455999387956));
#6789=CARTESIAN_POINT('Ctrl Pts',(3.32816065133725,56.371376638691,-5.05090428275669));
#6790=CARTESIAN_POINT('Ctrl Pts',(4.49799175700267,56.3531854412059,-4.04587574413293));
#6791=CARTESIAN_POINT('Ctrl Pts',(4.98258729451814,56.3435053739532,-3.43145079870755));
#6792=CARTESIAN_POINT('Ctrl Pts',(5.69989537662752,56.3239079934447,-2.03526034708743));
#6793=CARTESIAN_POINT('Ctrl Pts',(5.91900359014787,56.3141843310689,-1.26352907871823));
#6794=CARTESIAN_POINT('Ctrl Pts',(6.04106600107415,56.2966608626863,0.284746825533261));
#6795=CARTESIAN_POINT('Ctrl Pts',(5.95671079979978,56.288411058258,1.04554755236564));
#6796=CARTESIAN_POINT('Ctrl Pts',(5.50016128983585,56.2695539572171,2.52390294774796));
#6797=CARTESIAN_POINT('Ctrl Pts',(5.1211965582148,56.2596049286264,3.22415944935899));
#6798=CARTESIAN_POINT('Ctrl Pts',(4.13262816737534,56.2405274921602,4.41570731546272));
#6799=CARTESIAN_POINT('Ctrl Pts',(3.54093488582301,56.2317616860728,4.90294124689549));
#6800=CARTESIAN_POINT('Ctrl Pts',(2.1769282763679,56.2147116034546,5.64728331917592));
#6801=CARTESIAN_POINT('Ctrl Pts',(1.41108733546057,56.2051385916932,5.88554479318212));
#6802=CARTESIAN_POINT('Ctrl Pts',(-0.154051268862532,56.1855743591392,6.04844370577617));
#6803=CARTESIAN_POINT('Ctrl Pts',(-0.937571873767269,56.1757803515779,5.97732115913926));
#6804=CARTESIAN_POINT('Ctrl Pts',(-2.41623675328628,56.1572970405839,5.5444969437559));
#6805=CARTESIAN_POINT('Ctrl Pts',(-3.09957176867773,56.1493488123132,5.19348606835151));
#6806=CARTESIAN_POINT('Ctrl Pts',(-4.32991740497706,56.1312303713413,4.23011656908343));
#6807=CARTESIAN_POINT('Ctrl Pts',(-4.8555092940329,56.1212833886199,3.61470428341965));
#6808=CARTESIAN_POINT('Ctrl Pts',(-5.61890970623177,56.101639711652,2.24084856725757));
#6809=CARTESIAN_POINT('Ctrl Pts',(-5.85993019338523,56.0921306525639,1.50159255851692));
#6810=CARTESIAN_POINT('Ctrl Pts',(-6.05012504695993,56.0743068999117,-0.0350861342543961));
#6811=CARTESIAN_POINT('Ctrl Pts',(-5.99461604293912,56.0661065790627,-0.818430606491861));
#6812=CARTESIAN_POINT('Ctrl Pts',(-5.58416036006447,56.0471445058752,-2.33309519696156));
#6813=CARTESIAN_POINT('Ctrl Pts',(-5.22812325350618,56.0371755875623,-3.04842630508126));
#6814=CARTESIAN_POINT('Ctrl Pts',(-4.27712108424128,56.0179400054575,-4.27627190765333));
#6815=CARTESIAN_POINT('Ctrl Pts',(-3.70021645348818,56.0088357393135,-4.78421194524034));
#6816=CARTESIAN_POINT('Ctrl Pts',(-2.35933157194477,55.9919105321677,-5.57353536219895));
#6817=CARTESIAN_POINT('Ctrl Pts',(-1.60167263802065,55.9825209079752,-5.83655998386992));
#6818=CARTESIAN_POINT('Ctrl Pts',(-0.544202575513397,55.9693025321939,-5.98150876757896));
#6819=CARTESIAN_POINT('Ctrl Pts',(-0.271968436546483,55.9658996054568,-6.));
#6820=CARTESIAN_POINT('Ctrl Pts',(-3.30985239216375E-14,55.9625,-6.));
#6821=CARTESIAN_POINT('Ctrl Pts',(-2.78943534937071E-14,55.906249998771,
-6.));
#6822=CARTESIAN_POINT('Ctrl Pts',(-0.119270180566787,55.907740876028,-6.));
#6823=CARTESIAN_POINT('Ctrl Pts',(-0.238658191670233,55.9092332261669,-5.99644370777172));
#6824=CARTESIAN_POINT('Ctrl Pts',(-1.15097298881717,55.9206371611312,-5.94191079972275));
#6825=CARTESIAN_POINT('Ctrl Pts',(-1.92669402478814,55.9303336740808,-5.73750039954501));
#6826=CARTESIAN_POINT('Ctrl Pts',(-3.32126851885456,55.9477658552566,-5.05417095172651));
#6827=CARTESIAN_POINT('Ctrl Pts',(-3.93304275666383,55.9560978579313,-4.59419853981487));
#6828=CARTESIAN_POINT('Ctrl Pts',(-4.97046981399306,55.9749552855053,-3.45118278885069));
#6829=CARTESIAN_POINT('Ctrl Pts',(-5.3788842150237,55.9848605335407,-2.77197333408993));
#6830=CARTESIAN_POINT('Ctrl Pts',(-5.91480788525159,56.0043155350143,-1.28421295529728));
#6831=CARTESIAN_POINT('Ctrl Pts',(-6.03284998524064,56.0132540892278,-0.488724428843167));
#6832=CARTESIAN_POINT('Ctrl Pts',(-5.95307864390457,56.0306320858508,1.07053013027671));
#6833=CARTESIAN_POINT('Ctrl Pts',(-5.76824859512135,56.0399007335379,1.82001944980712));
#6834=CARTESIAN_POINT('Ctrl Pts',(-5.11449349917068,56.0593188805931,3.2363453578896));
#6835=CARTESIAN_POINT('Ctrl Pts',(-4.64117525801476,56.0692965738505,3.88477476699456));
#6836=CARTESIAN_POINT('Ctrl Pts',(-3.49281748541018,56.0878739702295,4.93787646592986));
#6837=CARTESIAN_POINT('Ctrl Pts',(-2.837096009414,56.0957862986533,5.34165539099934));
#6838=CARTESIAN_POINT('Ctrl Pts',(-1.37551778539592,56.1140560264535,5.8946789976836));
#6839=CARTESIAN_POINT('Ctrl Pts',(-0.578636157799252,56.1240170467985,6.02531808526819));
#6840=CARTESIAN_POINT('Ctrl Pts',(0.988783613055412,56.1436097939341,5.96770974701454));
#6841=CARTESIAN_POINT('Ctrl Pts',(1.7446548179888,56.1530581839958,5.79201578404849));
#6842=CARTESIAN_POINT('Ctrl Pts',(3.16108939615775,56.1707636162229,5.15941578064434));
#6843=CARTESIAN_POINT('Ctrl Pts',(3.80617671912254,56.1791192213777,4.70373101437893));
#6844=CARTESIAN_POINT('Ctrl Pts',(4.89006630320523,56.1982183667389,3.56521148303067));
#6845=CARTESIAN_POINT('Ctrl Pts',(5.31630477201846,56.2081762283405,2.89143252553516));
#6846=CARTESIAN_POINT('Ctrl Pts',(5.87286095503918,56.2273143187955,1.44485931946931));
#6847=CARTESIAN_POINT('Ctrl Pts',(6.00851807636355,56.2362297678481,0.689771261951205));
#6848=CARTESIAN_POINT('Ctrl Pts',(5.99025571610193,56.2531707988027,-0.864630364559025));
#6849=CARTESIAN_POINT('Ctrl Pts',(5.82334149419617,56.2627057874727,-1.64906691766854));
#6850=CARTESIAN_POINT('Ctrl Pts',(5.19927143500941,56.2822543761502,-3.09458117064177));
#6851=CARTESIAN_POINT('Ctrl Pts',(4.75319161261995,56.2920703642246,-3.74379900224259));
#6852=CARTESIAN_POINT('Ctrl Pts',(3.65167466294551,56.3106176781953,-4.82116536902607));
#6853=CARTESIAN_POINT('Ctrl Pts',(3.01182230798196,56.3186022199212,-5.24473876155051));
#6854=CARTESIAN_POINT('Ctrl Pts',(1.5780185312142,56.3365247671308,-5.84284081098096));
#6855=CARTESIAN_POINT('Ctrl Pts',(0.792860950716405,56.346339236887,-6.));
#6856=CARTESIAN_POINT('Ctrl Pts',(-3.28903571045203E-14,56.3562499987709,
-6.));
#6857=CARTESIAN_POINT('Origin',(0.,50.,0.));
#6858=CARTESIAN_POINT('',(1.97553982815868E-14,56.8625,-6.));
#6859=CARTESIAN_POINT('',(1.82982305617662E-14,56.806249998771,-6.));
#6860=CARTESIAN_POINT('',(-7.34788079488412E-16,50.,-6.));
#6861=CARTESIAN_POINT('Ctrl Pts',(5.19029264012261E-14,56.8625,-6.));
#6862=CARTESIAN_POINT('Ctrl Pts',(0.79230170443347,56.8525962286946,-6.));
#6863=CARTESIAN_POINT('Ctrl Pts',(1.57692203908962,56.8427884745114,-5.84306232652071));
#6864=CARTESIAN_POINT('Ctrl Pts',(3.01039884018676,56.8248700144976,-5.24555843097968));
#6865=CARTESIAN_POINT('Ctrl Pts',(3.65038030404161,56.8168864084426,-4.8221481831563));
#6866=CARTESIAN_POINT('Ctrl Pts',(4.7521810297415,56.7983405201061,-3.74507734898934));
#6867=CARTESIAN_POINT('Ctrl Pts',(5.19842465106967,56.788525009161,-3.09599816206786));
#6868=CARTESIAN_POINT('Ctrl Pts',(5.82288616449566,56.7689760372507,-1.65067451377228));
#6869=CARTESIAN_POINT('Ctrl Pts',(5.9900170998114,56.7594401809463,-0.866282931574435));
#6870=CARTESIAN_POINT('Ctrl Pts',(6.00870781223811,56.7424966987589,0.688097820879049));
#6871=CARTESIAN_POINT('Ctrl Pts',(5.87326509905218,56.7335847363924,1.44320666884808));
#6872=CARTESIAN_POINT('Ctrl Pts',(5.31713429155998,56.7144479987091,2.88990050189163));
#6873=CARTESIAN_POINT('Ctrl Pts',(4.89110382406863,56.7044903178273,3.56378285482827));
#6874=CARTESIAN_POINT('Ctrl Pts',(3.80752381648088,56.6853893334694,4.70265099948569));
#6875=CARTESIAN_POINT('Ctrl Pts',(3.16251190645564,56.6770313988307,5.15855339423183));
#6876=CARTESIAN_POINT('Ctrl Pts',(1.74620643543745,56.6593275804429,5.79154551234025));
#6877=CARTESIAN_POINT('Ctrl Pts',(0.990402786055763,56.6498800348257,5.96743864857926));
#6878=CARTESIAN_POINT('Ctrl Pts',(-0.576957627503505,56.6302880296562,6.02547594392505));
#6879=CARTESIAN_POINT('Ctrl Pts',(-1.37385210404051,56.6203268486995,5.89506426277027));
#6880=CARTESIAN_POINT('Ctrl Pts',(-2.83559237052781,56.6020550953684,5.34245766139812));
#6881=CARTESIAN_POINT('Ctrl Pts',(-3.4914506638857,56.5941430230773,4.93884724332227));
#6882=CARTESIAN_POINT('Ctrl Pts',(-4.62742573681593,56.5757721178423,3.89767122424419));
#6883=CARTESIAN_POINT('Ctrl Pts',(-5.09317321362636,56.566019397227,3.26565291573955));
#6884=CARTESIAN_POINT('Ctrl Pts',(-5.76454703716699,56.54643519543,1.84415970479431));
#6885=CARTESIAN_POINT('Ctrl Pts',(-5.95779467092296,56.5367998826718,1.06565921181134));
#6886=CARTESIAN_POINT('Ctrl Pts',(-6.02824627631527,56.5195630499973,-0.485935932386859));
#6887=CARTESIAN_POINT('Ctrl Pts',(-5.91853504504944,56.5110271148658,-1.24372602530261));
#6888=CARTESIAN_POINT('Ctrl Pts',(-5.4133585673446,56.4920557629773,-2.70456066906765));
#6889=CARTESIAN_POINT('Ctrl Pts',(-5.01242265950065,56.4821256339637,-3.39038624019974));
#6890=CARTESIAN_POINT('Ctrl Pts',(-3.96637907523528,56.4628090686586,-4.570840563839));
#6891=CARTESIAN_POINT('Ctrl Pts',(-3.33041263228381,56.4541301579035,-5.05302690239553));
#6892=CARTESIAN_POINT('Ctrl Pts',(-1.92967253351213,56.4366209066689,-5.73270782100113));
#6893=CARTESIAN_POINT('Ctrl Pts',(-1.18226194780873,56.4272782743476,-5.9321004182363));
#6894=CARTESIAN_POINT('Ctrl Pts',(-0.278410879134601,56.4159801359892,-5.99516091994516));
#6895=CARTESIAN_POINT('Ctrl Pts',(-0.139128323189838,56.4142391040399,-6.));
#6896=CARTESIAN_POINT('Ctrl Pts',(-3.15719672627779E-15,56.4125,-6.));
#6897=CARTESIAN_POINT('Ctrl Pts',(-2.79634361094744E-14,56.356249998771,
-6.));
#6898=CARTESIAN_POINT('Ctrl Pts',(-0.00925431949252112,56.3563656777646,
-6.));
#6899=CARTESIAN_POINT('Ctrl Pts',(-0.0185096884686758,56.3564813698768,
-5.99997858939597));
#6900=CARTESIAN_POINT('Ctrl Pts',(-0.799046772047178,56.3662380834215,-5.996366480783));
#6901=CARTESIAN_POINT('Ctrl Pts',(-1.56245757872404,56.375780718505,-5.84411035638461));
#6902=CARTESIAN_POINT('Ctrl Pts',(-2.99377584853423,56.3936721968776,-5.25727495839769));
#6903=CARTESIAN_POINT('Ctrl Pts',(-3.64762391318448,56.4017977100718,-4.82664253757592));
#6904=CARTESIAN_POINT('Ctrl Pts',(-4.76701621692779,56.4206793476575,-3.7287130186124));
#6905=CARTESIAN_POINT('Ctrl Pts',(-5.21720131349499,56.4306526218535,-3.06733589861962));
#6906=CARTESIAN_POINT('Ctrl Pts',(-5.82300969662807,56.4499413548937,-1.63528269760468));
#6907=CARTESIAN_POINT('Ctrl Pts',(-5.98351994764647,56.4590918575462,-0.882666107090339));
#6908=CARTESIAN_POINT('Ctrl Pts',(-6.01470652529258,56.4761376036864,0.673946893518462));
#6909=CARTESIAN_POINT('Ctrl Pts',(-5.87276684295458,56.4853870058037,1.46340278074942));
#6910=CARTESIAN_POINT('Ctrl Pts',(-5.2939284322367,56.5048849006054,2.93034863848238));
#6911=CARTESIAN_POINT('Ctrl Pts',(-4.86693149478656,56.5147510685449,3.59521939622588));
#6912=CARTESIAN_POINT('Ctrl Pts',(-3.79815452074611,56.5334597809641,4.70639754678297));
#6913=CARTESIAN_POINT('Ctrl Pts',(-3.17290832994337,56.5415886446467,5.14866957910816));
#6914=CARTESIAN_POINT('Ctrl Pts',(-1.7585265333779,56.5592684171037,5.79126668266434));
#6915=CARTESIAN_POINT('Ctrl Pts',(-0.977092871982791,56.5690363378712,5.97297738342711));
#6916=CARTESIAN_POINT('Ctrl Pts',(0.590525770206689,56.5886315708985,6.02081222645328));
#6917=CARTESIAN_POINT('Ctrl Pts',(1.36136697655774,56.5982670859779,5.8945391065037));
#6918=CARTESIAN_POINT('Ctrl Pts',(2.80851390396222,56.6163564225705,5.35766563810351));
#6919=CARTESIAN_POINT('Ctrl Pts',(3.47188226102197,56.6243247365624,4.95362155480435));
#6920=CARTESIAN_POINT('Ctrl Pts',(4.62865756826947,56.64296324636,3.89973430600555));
#6921=CARTESIAN_POINT('Ctrl Pts',(5.10420827628955,56.6529408032822,3.25260640731597));
#6922=CARTESIAN_POINT('Ctrl Pts',(5.76260847138282,56.6723705134876,1.83789419040876));
#6923=CARTESIAN_POINT('Ctrl Pts',(5.94980260893631,56.6816501951599,1.08875050227638));
#6924=CARTESIAN_POINT('Ctrl Pts',(6.03425140366107,56.6990475013165,-0.46958726618876));
#6925=CARTESIAN_POINT('Ctrl Pts',(5.91892429640393,56.7079457666895,-1.26453978936345));
#6926=CARTESIAN_POINT('Ctrl Pts',(5.38837502284035,56.7273807618557,-2.75355497399551));
#6927=CARTESIAN_POINT('Ctrl Pts',(4.98213291703594,56.7372899804404,-3.43438538763148));
#6928=CARTESIAN_POINT('Ctrl Pts',(3.94834137551491,56.7561642773249,-4.58105842476809));
#6929=CARTESIAN_POINT('Ctrl Pts',(3.33809854614214,56.7645237669442,-5.04307208402363));
#6930=CARTESIAN_POINT('Ctrl Pts',(1.94581237222651,56.7819273441181,-5.73104345580422));
#6931=CARTESIAN_POINT('Ctrl Pts',(1.17078731673957,56.7916151573117,-5.93803703272594));
#6932=CARTESIAN_POINT('Ctrl Pts',(0.251991343217977,56.8031001069807,-5.99603536758937));
#6933=CARTESIAN_POINT('Ctrl Pts',(0.125931641266464,56.8046758532551,-6.));
#6934=CARTESIAN_POINT('Ctrl Pts',(1.76941794549634E-15,56.806249998771,
-6.));
#6935=CARTESIAN_POINT('Origin',(0.,50.,0.));
#6936=CARTESIAN_POINT('',(3.74495777365502E-14,57.3125,-6.));
#6937=CARTESIAN_POINT('',(-3.54435027239952E-14,57.256249998771,-6.));
#6938=CARTESIAN_POINT('',(-7.34788079488412E-16,50.,-6.));
#6939=CARTESIAN_POINT('Ctrl Pts',(1.02071129326475E-13,57.3125,-6.));
#6940=CARTESIAN_POINT('Ctrl Pts',(0.125400103295474,57.3109324987088,-6.));
#6941=CARTESIAN_POINT('Ctrl Pts',(0.250927449357367,57.309363406883,-5.99606876480776));
#6942=CARTESIAN_POINT('Ctrl Pts',(1.16920671278006,57.2978849160902,-5.93834856646838));
#6943=CARTESIAN_POINT('Ctrl Pts',(1.94428762714173,57.2881964046607,-5.73156102449072));
#6944=CARTESIAN_POINT('Ctrl Pts',(3.33675657998753,57.2707905427501,-5.04395995896572));
#6945=CARTESIAN_POINT('Ctrl Pts',(3.947121550112,57.2624332788191,-4.582109327563));
#6946=CARTESIAN_POINT('Ctrl Pts',(4.98120359387457,57.2435603269992,-3.43572826371665));
#6947=CARTESIAN_POINT('Ctrl Pts',(5.38761940453579,57.2336514214288,-2.75502705365286));
#6948=CARTESIAN_POINT('Ctrl Pts',(5.91859783697493,57.2142148248932,-1.26611171583379));
#6949=CARTESIAN_POINT('Ctrl Pts',(6.03414160801522,57.2053133699899,-0.471116428454863));
#6950=CARTESIAN_POINT('Ctrl Pts',(5.95006647750491,57.1879176050029,1.08729470798663));
#6951=CARTESIAN_POINT('Ctrl Pts',(5.76306126409791,57.1786388021573,1.83646628899214));
#6952=CARTESIAN_POINT('Ctrl Pts',(5.10503217547553,57.1592100093662,3.25130801722047));
#6953=CARTESIAN_POINT('Ctrl Pts',(4.62965976686184,57.1492324378488,3.89854020536501));
#6954=CARTESIAN_POINT('Ctrl Pts',(3.47314670683594,57.1305921723927,4.95274104346126));
#6955=CARTESIAN_POINT('Ctrl Pts',(2.80984639355393,57.1226230799194,5.35697242982361));
#6956=CARTESIAN_POINT('Ctrl Pts',(1.36281102046722,57.1045351377558,5.89420296635131));
#6957=CARTESIAN_POINT('Ctrl Pts',(0.592019886103502,57.0949002485763,6.02066309919394));
#6958=CARTESIAN_POINT('Ctrl Pts',(-0.975592711237711,57.0753050911095,5.97322267694157));
#6959=CARTESIAN_POINT('Ctrl Pts',(-1.75707259140603,57.0655365926074,5.79170805839118));
#6960=CARTESIAN_POINT('Ctrl Pts',(-3.17162316846255,57.0478547103942,5.14946248351839));
#6961=CARTESIAN_POINT('Ctrl Pts',(-3.79698591448204,57.0397273059984,4.70734163143148));
#6962=CARTESIAN_POINT('Ctrl Pts',(-4.86602922517863,57.0210198816722,3.59643623934408));
#6963=CARTESIAN_POINT('Ctrl Pts',(-5.29318280569659,57.0111540831499,2.93169004482648));
#6964=CARTESIAN_POINT('Ctrl Pts',(-5.87238998366337,56.9916557125567,1.46491314322759));
#6965=CARTESIAN_POINT('Ctrl Pts',(-6.01453244277215,56.9824032869153,0.675496041203355));
#6966=CARTESIAN_POINT('Ctrl Pts',(-5.98374780588059,56.9653602002944,-0.88110334414595));
#6967=CARTESIAN_POINT('Ctrl Pts',(-5.82343943906002,56.9562107136636,-1.63374263648686));
#6968=CARTESIAN_POINT('Ctrl Pts',(-5.21803030381155,56.9369231345048,-3.06591975237485));
#6969=CARTESIAN_POINT('Ctrl Pts',(-4.76803851417126,56.9269499412634,-3.72740099990421));
#6970=CARTESIAN_POINT('Ctrl Pts',(-3.64893183786213,56.9080665015842,-4.82566189620856));
#6971=CARTESIAN_POINT('Ctrl Pts',(-2.99515524025006,56.8999394405031,-5.25649662540572));
#6972=CARTESIAN_POINT('Ctrl Pts',(-1.56395731254144,56.8820494664067,-5.84370662915294));
#6973=CARTESIAN_POINT('Ctrl Pts',(-0.800605409757413,56.872507567622,-5.99615608358869));
#6974=CARTESIAN_POINT('Ctrl Pts',(-0.0195622404979201,56.8627445280062,
-5.99997608528796));
#6975=CARTESIAN_POINT('Ctrl Pts',(-0.00978053498370382,56.8626222566873,
-6.));
#6976=CARTESIAN_POINT('Ctrl Pts',(5.85670370643913E-14,56.8625,-6.));
#6977=CARTESIAN_POINT('Ctrl Pts',(-6.93889390390723E-16,56.806249998771,
-6.));
#6978=CARTESIAN_POINT('Ctrl Pts',(-0.648402459143038,56.8143550295102,-6.));
#6979=CARTESIAN_POINT('Ctrl Pts',(-1.29340995251398,56.8224176231774,-5.89488504120407));
#6980=CARTESIAN_POINT('Ctrl Pts',(-2.63511788894843,56.8391889723828,-5.4444243204798));
#6981=CARTESIAN_POINT('Ctrl Pts',(-3.30731393856354,56.8470979035384,-5.06431401286994));
#6982=CARTESIAN_POINT('Ctrl Pts',(-4.49746487288741,56.8655072495993,-4.05086543056204));
#6983=CARTESIAN_POINT('Ctrl Pts',(-4.99572570987037,56.8754775890921,-3.41751594850567));
#6984=CARTESIAN_POINT('Ctrl Pts',(-5.70156528953609,56.8950153414053,-2.02021237064714));
#6985=CARTESIAN_POINT('Ctrl Pts',(-5.91298550005615,56.9044034627066,-1.27503838843151));
#6986=CARTESIAN_POINT('Ctrl Pts',(-6.04518225838507,56.9219957161009,0.273740534820731));
#6987=CARTESIAN_POINT('Ctrl Pts',(-5.95722502302248,56.9305281010994,1.06331834350479));
#6988=CARTESIAN_POINT('Ctrl Pts',(-5.48124632997723,56.9497541962257,2.56454250840581));
#6989=CARTESIAN_POINT('Ctrl Pts',(-5.09742898458621,56.9596974651858,3.26146530244624));
#6990=CARTESIAN_POINT('Ctrl Pts',(-4.10086736349352,56.9787399104357,4.44516592481387));
#6991=CARTESIAN_POINT('Ctrl Pts',(-3.5059602233989,56.9874254959785,4.92796363125023));
#6992=CARTESIAN_POINT('Ctrl Pts',(-2.1369822837587,57.004537720224,5.66252364490185));
#6993=CARTESIAN_POINT('Ctrl Pts',(-1.36945084820307,57.0141318631684,5.89537543174104));
#6994=CARTESIAN_POINT('Ctrl Pts',(0.196296765378441,57.0337037083382,6.04715142045329));
#6995=CARTESIAN_POINT('Ctrl Pts',(0.978759606102301,57.0434844938472,5.97064561121902));
#6996=CARTESIAN_POINT('Ctrl Pts',(2.45446398587465,57.0619307985944,5.52775699432585));
#6997=CARTESIAN_POINT('Ctrl Pts',(3.13584909447357,57.0698632821768,5.17174421812721));
#6998=CARTESIAN_POINT('Ctrl Pts',(4.35931772271835,57.0880326402888,4.19970075246771));
#6999=CARTESIAN_POINT('Ctrl Pts',(4.88023982560178,57.097984791888,3.58111488403131));
#7000=CARTESIAN_POINT('Ctrl Pts',(5.63376775666096,57.1176123046472,2.20305247385668));
#7001=CARTESIAN_POINT('Ctrl Pts',(5.86969505471758,57.12710146791,1.46269380863545));
#7002=CARTESIAN_POINT('Ctrl Pts',(6.04992953488621,57.1448858782599,-0.0761012221813032));
#7003=CARTESIAN_POINT('Ctrl Pts',(5.98890670457258,57.1531344045418,-0.860489554575097));
#7004=CARTESIAN_POINT('Ctrl Pts',(5.56726068923777,57.1721425446805,-2.37294888625735));
#7005=CARTESIAN_POINT('Ctrl Pts',(5.20641527721435,57.1821082694806,-3.08520891385342));
#7006=CARTESIAN_POINT('Ctrl Pts',(4.24754836417997,57.2013118582877,-4.30555839024504));
#7007=CARTESIAN_POINT('Ctrl Pts',(3.66757324889836,57.2103888076896,-4.80920227021172));
#7008=CARTESIAN_POINT('Ctrl Pts',(2.32190020184786,57.2272432574316,-5.58922494954457));
#7009=CARTESIAN_POINT('Ctrl Pts',(1.56254663837337,57.2367181657913,-5.84714922855423));
#7010=CARTESIAN_POINT('Ctrl Pts',(0.517503993885004,57.2497811988474,-5.98327958263317));
#7011=CARTESIAN_POINT('Ctrl Pts',(0.258618334561658,57.2530172695889,-6.));
#7012=CARTESIAN_POINT('Ctrl Pts',(-4.9960036108132E-14,57.256249998771,
-6.));
#7013=CARTESIAN_POINT('Origin',(0.,50.,0.));
#7014=CARTESIAN_POINT('',(3.55066874434562E-14,57.7625,-6.));
#7015=CARTESIAN_POINT('',(-6.07565071524461E-15,57.706249998771,-6.));
#7016=CARTESIAN_POINT('',(-7.34788079488412E-16,50.,-6.));
#7017=CARTESIAN_POINT('Ctrl Pts',(3.67761376907083E-14,57.7625,-6.));
#7018=CARTESIAN_POINT('Ctrl Pts',(0.258110612055831,57.7592736173493,-6.));
#7019=CARTESIAN_POINT('Ctrl Pts',(0.516488526706724,57.7560438934161,-5.98334517000259));
#7020=CARTESIAN_POINT('Ctrl Pts',(1.56105720933857,57.7429867848832,-5.84754679167773));
#7021=CARTESIAN_POINT('Ctrl Pts',(2.32047460153356,57.7335085743511,-5.589816681709));
#7022=CARTESIAN_POINT('Ctrl Pts',(3.66632852427493,57.7166568288435,-4.81014823747084));
#7023=CARTESIAN_POINT('Ctrl Pts',(4.24641978670145,57.7075809259861,-4.3066680907309));
#7024=CARTESIAN_POINT('Ctrl Pts',(5.20558465828751,57.6883785712772,-3.08660464190133));
#7025=CARTESIAN_POINT('Ctrl Pts',(5.56661242618428,57.6784129776166,-2.37446201166824));
#7026=CARTESIAN_POINT('Ctrl Pts',(5.9886840232526,57.6594030932603,-0.862087265793267));
#7027=CARTESIAN_POINT('Ctrl Pts',(6.04991675977275,57.6511526636423,-0.0776590515749793));
#7028=CARTESIAN_POINT('Ctrl Pts',(5.87006062165887,57.6333697511002,1.46121605357551));
#7029=CARTESIAN_POINT('Ctrl Pts',(5.63432672297646,57.6238813508433,2.20161589450978));
#7030=CARTESIAN_POINT('Ctrl Pts',(4.88117393256969,57.6042544688462,3.57983662493059));
#7031=CARTESIAN_POINT('Ctrl Pts',(4.36042942270714,57.5943021304438,4.19854228289295));
#7032=CARTESIAN_POINT('Ctrl Pts',(3.13722222214314,57.5761308460079,5.17091463006621));
#7033=CARTESIAN_POINT('Ctrl Pts',(2.45591086078362,57.5681988857598,5.52711735424255));
#7034=CARTESIAN_POINT('Ctrl Pts',(0.980318986417133,57.5497539873302,5.97038714552931));
#7035=CARTESIAN_POINT('Ctrl Pts',(0.197896924777086,57.5399737115597,6.04709666809083));
#7036=CARTESIAN_POINT('Ctrl Pts',(-1.36787220453393,57.5204015974433,5.89574204871011));
#7037=CARTESIAN_POINT('Ctrl Pts',(-2.13546691100742,57.5108066636124,5.6630954373108));
#7038=CARTESIAN_POINT('Ctrl Pts',(-3.50463273732457,57.4936920907834,4.92890615136674));
#7039=CARTESIAN_POINT('Ctrl Pts',(-4.09966171028527,57.4850094645677,4.44627606041768));
#7040=CARTESIAN_POINT('Ctrl Pts',(-5.09652503725565,57.465968347838,3.26287235145577));
#7041=CARTESIAN_POINT('Ctrl Pts',(-5.48052530547623,57.4560253069035,2.5660762320662));
#7042=CARTESIAN_POINT('Ctrl Pts',(-5.9569427420416,57.4367974913717,1.06494645160616));
#7043=CARTESIAN_POINT('Ctrl Pts',(-6.04511867915217,57.4282624831873,0.275326005877001));
#7044=CARTESIAN_POINT('Ctrl Pts',(-5.91330773664244,57.410671789239,-1.2735316127887));
#7045=CARTESIAN_POINT('Ctrl Pts',(-5.70208388348488,57.4012845128089,-2.01874091612926));
#7046=CARTESIAN_POINT('Ctrl Pts',(-4.9966276237321,57.3817475593453,-3.41619200927743));
#7047=CARTESIAN_POINT('Ctrl Pts',(-4.49854962822897,57.3717771185393,-4.04965641382376));
#7048=CARTESIAN_POINT('Ctrl Pts',(-3.30866732480217,57.3533658829282,-5.06343463942207));
#7049=CARTESIAN_POINT('Ctrl Pts',(-2.63654373742122,57.3454567967178,-5.4437383734588));
#7050=CARTESIAN_POINT('Ctrl Pts',(-1.2944343830689,57.3286804297884,-5.89471689272042));
#7051=CARTESIAN_POINT('Ctrl Pts',(-0.648920882495232,57.3206115110312,-6.));
#7052=CARTESIAN_POINT('Ctrl Pts',(1.08385522779031E-13,57.3125,-6.));
#7053=CARTESIAN_POINT('Ctrl Pts',(-4.76008121808036E-14,57.256249998771,
-6.));
#7054=CARTESIAN_POINT('Ctrl Pts',(-0.519436872236381,57.2627429596739,-5.99999999999999));
#7055=CARTESIAN_POINT('Ctrl Pts',(-1.03779532898449,57.2692224403833,-5.93254268395134));
#7056=CARTESIAN_POINT('Ctrl Pts',(-2.27613559137132,57.2847016936631,-5.60325267671887));
#7057=CARTESIAN_POINT('Ctrl Pts',(-2.96664814970964,57.2927387106259,-5.27031552020861));
#7058=CARTESIAN_POINT('Ctrl Pts',(-4.21457381419212,57.3105680471163,-4.34380218297167));
#7059=CARTESIAN_POINT('Ctrl Pts',(-4.75210513328209,57.3203755926538,-3.74816378575814));
#7060=CARTESIAN_POINT('Ctrl Pts',(-5.5526541858912,57.3399623225271,-2.40101639440333));
#7061=CARTESIAN_POINT('Ctrl Pts',(-5.81536420644968,57.3495518110932,-1.66685308668976));
#7062=CARTESIAN_POINT('Ctrl Pts',(-6.04792418952215,57.367540960483,-0.139355216686795));
#7063=CARTESIAN_POINT('Ctrl Pts',(-6.01561379010144,57.375577236203,0.639687804988226));
#7064=CARTESIAN_POINT('Ctrl Pts',(-5.65245436363216,57.3943403650438,2.16328121029141));
#7065=CARTESIAN_POINT('Ctrl Pts',(-5.31701861410011,57.4043173426411,2.89125100224821));
#7066=CARTESIAN_POINT('Ctrl Pts',(-4.39988869026892,57.4236783666517,4.15024058173161));
#7067=CARTESIAN_POINT('Ctrl Pts',(-3.83630861676176,57.432893754617,4.67613855017113));
#7068=CARTESIAN_POINT('Ctrl Pts',(-2.51103415904724,57.4501797145846,5.5077995677353));
#7069=CARTESIAN_POINT('Ctrl Pts',(-1.75440706620821,57.4593199104434,5.79337860149726));
#7070=CARTESIAN_POINT('Ctrl Pts',(-0.190516556092516,57.4788685418198,6.04797102451951));
#7071=CARTESIAN_POINT('Ctrl Pts',(0.600273930605387,57.4887534229035,6.02112312229376));
#7072=CARTESIAN_POINT('Ctrl Pts',(2.10239675516878,57.5075299582106,5.67059173961374));
#7073=CARTESIAN_POINT('Ctrl Pts',(2.80190577330558,57.5157428591829,5.3595703237078));
#7074=CARTESIAN_POINT('Ctrl Pts',(4.07717959526911,57.5333107146008,4.47300103937156));
#7075=CARTESIAN_POINT('Ctrl Pts',(4.63295849576113,57.5430472346991,3.89445893722693));
#7076=CARTESIAN_POINT('Ctrl Pts',(5.47632776170528,57.5626446916676,2.57104288095419));
#7077=CARTESIAN_POINT('Ctrl Pts',(5.76225600572969,57.5723124689847,1.84305261576839));
#7078=CARTESIAN_POINT('Ctrl Pts',(6.04013983523531,57.5904750269888,0.325703679081649));
#7079=CARTESIAN_POINT('Ctrl Pts',(6.03222718366437,57.5984092303024,-0.44900774578563));
#7080=CARTESIAN_POINT('Ctrl Pts',(5.71911276192995,57.6169547111498,-1.98138918762898));
#7081=CARTESIAN_POINT('Ctrl Pts',(5.40594485041393,57.6269305930548,-2.72211410612992));
#7082=CARTESIAN_POINT('Ctrl Pts',(4.52573222705394,57.6464069267401,-4.01306975045855));
#7083=CARTESIAN_POINT('Ctrl Pts',(3.97684854565217,57.6557321097956,-4.55759512082249));
#7084=CARTESIAN_POINT('Ctrl Pts',(2.6826884329283,57.6732100113963,-5.4249508224125));
#7085=CARTESIAN_POINT('Ctrl Pts',(1.94417005043746,57.6819478731405,-5.73124160488625));
#7086=CARTESIAN_POINT('Ctrl Pts',(0.782107764040655,57.6964736517205,-5.96176932725523));
#7087=CARTESIAN_POINT('Ctrl Pts',(0.391053241759171,57.701361833249,-6.));
#7088=CARTESIAN_POINT('Ctrl Pts',(-1.94289029309402E-15,57.706249998771,
-6.));
#7089=CARTESIAN_POINT('Origin',(0.,50.,0.));
#7090=CARTESIAN_POINT('',(-1.93563819391985E-14,58.2125,-6.));
#7091=CARTESIAN_POINT('',(-1.96575190926063E-14,58.156249998771,-6.));
#7092=CARTESIAN_POINT('',(-7.34788079488412E-16,50.,-6.));
#7093=CARTESIAN_POINT('Ctrl Pts',(-7.84095011141517E-15,58.2125,-6.));
#7094=CARTESIAN_POINT('Ctrl Pts',(0.390457421837537,58.207619282227,-6.));
#7095=CARTESIAN_POINT('Ctrl Pts',(0.780918842935951,58.2027385144633,-5.96188574511026));
#7096=CARTESIAN_POINT('Ctrl Pts',(1.94253419381023,58.1882183225773,-5.73180637727347));
#7097=CARTESIAN_POINT('Ctrl Pts',(2.681207844968,58.1794773050473,-5.42569341007508));
#7098=CARTESIAN_POINT('Ctrl Pts',(3.97563925209768,58.1620010529719,-4.55864671700234));
#7099=CARTESIAN_POINT('Ctrl Pts',(4.52465365959551,58.1526767919982,-4.01428199965563));
#7100=CARTESIAN_POINT('Ctrl Pts',(5.40519277828591,58.1332013855122,-2.72360050849763));
#7101=CARTESIAN_POINT('Ctrl Pts',(5.71855682515151,58.1232254511625,-1.98298398415952));
#7102=CARTESIAN_POINT('Ctrl Pts',(6.03210756855281,58.1046780422682,-0.450676347406313));
#7103=CARTESIAN_POINT('Ctrl Pts',(6.04023242288917,58.0967432727997,0.324071772308548));
#7104=CARTESIAN_POINT('Ctrl Pts',(5.76274605643686,58.0785822192762,1.84151120643125));
#7105=CARTESIAN_POINT('Ctrl Pts',(5.47702135089854,58.0689150927559,2.56955886657416));
#7106=CARTESIAN_POINT('Ctrl Pts',(4.6340254354337,58.0493176466484,3.89318947355464));
#7107=CARTESIAN_POINT('Ctrl Pts',(4.07840450937353,58.0395804601485,4.47188434182551));
#7108=CARTESIAN_POINT('Ctrl Pts',(2.8033690403144,58.0220102826005,5.35880574845981));
#7109=CARTESIAN_POINT('Ctrl Pts',(2.10394053493841,58.0137992566867,5.6700197498057));
#7110=CARTESIAN_POINT('Ctrl Pts',(0.601929482491991,57.9950241185311,6.02095503373109));
#7111=CARTESIAN_POINT('Ctrl Pts',(-0.188831349820596,57.9851396081272,6.04802107703606));
#7112=CARTESIAN_POINT('Ctrl Pts',(-1.75284859095268,57.9655893926131,5.79386100479629));
#7113=CARTESIAN_POINT('Ctrl Pts',(-2.50962521800312,57.9564455943931,5.50845291559488));
#7114=CARTESIAN_POINT('Ctrl Pts',(-3.8351523571085,57.939161216313,4.67708391219656));
#7115=CARTESIAN_POINT('Ctrl Pts',(-4.39884929925911,57.9299467530942,4.15133884232404));
#7116=CARTESIAN_POINT('Ctrl Pts',(-5.31627458475805,57.9105867392603,2.8926131061046));
#7117=CARTESIAN_POINT('Ctrl Pts',(-5.65188924961675,57.9006097933443,2.16474953755615));
#7118=CARTESIAN_POINT('Ctrl Pts',(-6.01545511766878,57.8818449263436,0.641230227077598));
#7119=CARTESIAN_POINT('Ctrl Pts',(-6.0479642230219,57.8738075178057,-0.137848943610883));
#7120=CARTESIAN_POINT('Ctrl Pts',(-5.81577020278541,57.8558197836008,-1.66542737316983));
#7121=CARTESIAN_POINT('Ctrl Pts',(-5.55324765720755,57.8462309602226,-2.39963747219516));
#7122=CARTESIAN_POINT('Ctrl Pts',(-4.75304623800897,57.8266443944227,-3.7469704133501));
#7123=CARTESIAN_POINT('Ctrl Pts',(-4.21566411034092,57.8168363161938,-4.34274415418793));
#7124=CARTESIAN_POINT('Ctrl Pts',(-2.96796066775887,57.7990048960901,-5.26957826725007));
#7125=CARTESIAN_POINT('Ctrl Pts',(-2.27751928872034,57.790968991109,-5.60269206319514));
#7126=CARTESIAN_POINT('Ctrl Pts',(-1.03877270146848,57.7754846587683,-5.93241487607021));
#7127=CARTESIAN_POINT('Ctrl Pts',(-0.519928662438415,57.7689991082805,-6.));
#7128=CARTESIAN_POINT('Ctrl Pts',(8.11850586757146E-14,57.7625,-6.));
#7129=CARTESIAN_POINT('Ctrl Pts',(-1.28369537222284E-14,57.706249998771,
-6.));
#7130=CARTESIAN_POINT('Ctrl Pts',(-0.391601361600674,57.711145015791,-6.));
#7131=CARTESIAN_POINT('Ctrl Pts',(-0.783201439086809,57.7160400167596,-5.96166207261296));
#7132=CARTESIAN_POINT('Ctrl Pts',(-1.91335725960868,57.7301669645161,-5.73714195665658));
#7133=CARTESIAN_POINT('Ctrl Pts',(-2.62281749872555,57.73865054735,-5.44945314815992));
#7134=CARTESIAN_POINT('Ctrl Pts',(-3.92669804958441,57.7559342308597,-4.60565064288469));
#7135=CARTESIAN_POINT('Ctrl Pts',(-4.50127582338596,57.7655845989079,-4.04592046079129));
#7136=CARTESIAN_POINT('Ctrl Pts',(-5.38942554973876,57.7851724256882,-2.74924801407657));
#7137=CARTESIAN_POINT('Ctrl Pts',(-5.69991244388084,57.7949140509847,-2.02861490802512));
#7138=CARTESIAN_POINT('Ctrl Pts',(-6.02580821468928,57.813256188233,-0.52239685858074));
#7139=CARTESIAN_POINT('Ctrl Pts',(-6.04332107158197,57.821164533169,0.248056565886231));
#7140=CARTESIAN_POINT('Ctrl Pts',(-5.78257606509501,57.839474882712,1.78895300421315));
#7141=CARTESIAN_POINT('Ctrl Pts',(-5.49318999140679,57.8494389828867,2.54232002356862));
#7142=CARTESIAN_POINT('Ctrl Pts',(-4.65273329361551,57.8690165395379,3.86557933928005));
#7143=CARTESIAN_POINT('Ctrl Pts',(-4.11986225783113,57.8784478281965,4.42915123066452));
#7144=CARTESIAN_POINT('Ctrl Pts',(-2.85826880174532,57.8961207399164,5.3333235633937));
#7145=CARTESIAN_POINT('Ctrl Pts',(-2.13805071417483,57.9045243648438,5.6606351502864));
#7146=CARTESIAN_POINT('Ctrl Pts',(-0.607167279468976,57.9236604077776,6.02113734956474));
#7147=CARTESIAN_POINT('Ctrl Pts',(0.189158021930711,57.9336144740451,6.04871588527682));
#7148=CARTESIAN_POINT('Ctrl Pts',(1.71801944063456,57.9527252417789,5.79879535798965));
#7149=CARTESIAN_POINT('Ctrl Pts',(2.43798162431586,57.9615715966977,5.53478334131579));
#7150=CARTESIAN_POINT('Ctrl Pts',(3.77031407405033,57.9785619662946,4.73450272615289));
#7151=CARTESIAN_POINT('Ctrl Pts',(4.36322000407077,57.9881143046535,4.19440990478975));
#7152=CARTESIAN_POINT('Ctrl Pts',(5.29575070535321,58.007670328558,2.92629864971634));
#7153=CARTESIAN_POINT('Ctrl Pts',(5.63087522327058,58.0174765634655,2.21392170217679));
#7154=CARTESIAN_POINT('Ctrl Pts',(6.00512131537034,58.0359950673901,0.719326668055239));
#7155=CARTESIAN_POINT('Ctrl Pts',(6.04786576453849,58.0439618266081,-0.0472031294460459));
#7156=CARTESIAN_POINT('Ctrl Pts',(5.83917914624789,58.0620314364426,-1.59591691053384));
#7157=CARTESIAN_POINT('Ctrl Pts',(5.57387686409125,58.0719730483531,-2.3611113365425));
#7158=CARTESIAN_POINT('Ctrl Pts',(4.77400611905593,58.0916313179331,-3.71525890399387));
#7159=CARTESIAN_POINT('Ctrl Pts',(4.25766524315068,58.1011589707271,-4.29727622515334));
#7160=CARTESIAN_POINT('Ctrl Pts',(3.02845794881133,58.1190200122784,-5.23752540649854));
#7161=CARTESIAN_POINT('Ctrl Pts',(2.32577158057442,58.1271778540138,-5.58516084716442));
#7162=CARTESIAN_POINT('Ctrl Pts',(1.06150779516445,58.1429811513315,-5.92941344534358));
#7163=CARTESIAN_POINT('Ctrl Pts',(0.53134688384117,58.1496081627229,-6.));
#7164=CARTESIAN_POINT('Ctrl Pts',(-6.77236045021345E-14,58.156249998771,
-6.));
#7165=CARTESIAN_POINT('Origin',(0.,50.,0.));
#7166=CARTESIAN_POINT('',(7.61233394974911E-15,58.6625,-6.));
#7167=CARTESIAN_POINT('',(-2.14616315076222E-14,58.606249998771,-6.));
#7168=CARTESIAN_POINT('',(-7.34788079488412E-16,50.,-6.));
#7169=CARTESIAN_POINT('Ctrl Pts',(6.38378239159465E-14,58.6625,-6.));
#7170=CARTESIAN_POINT('Ctrl Pts',(0.530776948296579,58.6558652881463,-6.));
#7171=CARTESIAN_POINT('Ctrl Pts',(1.06037530332947,58.6492453087083,-5.92956480662758));
#7172=CARTESIAN_POINT('Ctrl Pts',(2.32423742973157,58.6334470321283,-5.58580676470304));
#7173=CARTESIAN_POINT('Ctrl Pts',(3.02706636248606,58.6252875032083,-5.23833760312848));
#7174=CARTESIAN_POINT('Ctrl Pts',(4.25654205503151,58.6074279973176,-4.2983852398153));
#7175=CARTESIAN_POINT('Ctrl Pts',(4.7730223061995,58.597901105114,-3.71651864733174));
#7176=CARTESIAN_POINT('Ctrl Pts',(5.57323346422887,58.5782434223283,-2.36262182315155));
#7177=CARTESIAN_POINT('Ctrl Pts',(5.83873697489378,58.5683015800684,-1.59752229770145));
#7178=CARTESIAN_POINT('Ctrl Pts',(6.04785491129762,58.5502299481763,-0.0488707485619556));
#7179=CARTESIAN_POINT('Ctrl Pts',(6.00531951855148,58.5422640224442,0.717690221353016));
#7180=CARTESIAN_POINT('Ctrl Pts',(5.63147665457864,58.5237469701109,2.21238396707949));
#7181=CARTESIAN_POINT('Ctrl Pts',(5.29655706242653,58.5139412327658,2.92483326571615));
#7182=CARTESIAN_POINT('Ctrl Pts',(4.3643932130471,58.4943848513782,4.19318934571028));
#7183=CARTESIAN_POINT('Ctrl Pts',(3.77163749598118,58.4848316490538,4.73344870227629));
#7184=CARTESIAN_POINT('Ctrl Pts',(2.43954091256409,58.4678388044587,5.53409412546177));
#7185=CARTESIAN_POINT('Ctrl Pts',(1.71966841461828,58.4589958551827,5.79830452948859));
#7186=CARTESIAN_POINT('Ctrl Pts',(0.190917060146435,58.4398864632518,6.04865757988973));
#7187=CARTESIAN_POINT('Ctrl Pts',(-0.605392310407389,58.4299325961199,6.02131301640874));
#7188=CARTESIAN_POINT('Ctrl Pts',(-2.13642329321222,58.4107947088348,5.66125848153069));
#7189=CARTESIAN_POINT('Ctrl Pts',(-2.85679415977466,58.4023886124107,5.33412305523624));
#7190=CARTESIAN_POINT('Ctrl Pts',(-4.11866454336098,58.3847173340954,4.43026149411868));
#7191=CARTESIAN_POINT('Ctrl Pts',(-4.65167436976604,58.3752869090688,3.8668495124502));
#7192=CARTESIAN_POINT('Ctrl Pts',(-5.49247371789428,58.3557101285827,2.54385972506567));
#7193=CARTESIAN_POINT('Ctrl Pts',(-5.78206393462196,58.3457458823708,1.7905970774123));
#7194=CARTESIAN_POINT('Ctrl Pts',(-6.04325418504873,58.3274335033081,0.249770221784229));
#7195=CARTESIAN_POINT('Ctrl Pts',(-6.02595721866325,58.3195252934994,-0.520718130671191));
#7196=CARTESIAN_POINT('Ctrl Pts',(-5.70047225331914,58.30118467433,-2.02703312465037));
#7197=CARTESIAN_POINT('Ctrl Pts',(-5.39019517581812,58.2914436403568,-2.74773274428987));
#7198=CARTESIAN_POINT('Ctrl Pts',(-4.50242576317489,58.271855638718,-4.04464091796179));
#7199=CARTESIAN_POINT('Ctrl Pts',(-3.92800637799208,58.2622044860682,-4.60453502415897));
#7200=CARTESIAN_POINT('Ctrl Pts',(-2.62436906678792,58.2449183407013,-5.44870538053932));
#7201=CARTESIAN_POINT('Ctrl Pts',(-1.91499593268198,58.2364374491585,-5.73659449375919));
#7202=CARTESIAN_POINT('Ctrl Pts',(-0.784344980001046,58.22230431225,-5.96154976010922));
#7203=CARTESIAN_POINT('Ctrl Pts',(-0.392174507256861,58.2174021813407,-6.));
#7204=CARTESIAN_POINT('Ctrl Pts',(1.45716771982052E-14,58.2125,-6.));
#7205=CARTESIAN_POINT('Ctrl Pts',(-5.02375918642883E-14,58.156249998771,
-6.));
#7206=CARTESIAN_POINT('Ctrl Pts',(-0.25714894131831,58.1594643605374,-6.));
#7207=CARTESIAN_POINT('Ctrl Pts',(-0.514575654230465,58.1626821944489,-5.9834690716322));
#7208=CARTESIAN_POINT('Ctrl Pts',(-1.5265971378732,58.1753324629944,-5.85239233164468));
#7209=CARTESIAN_POINT('Ctrl Pts',(-2.25698495692498,58.1844623107326,-5.6113307664574));
#7210=CARTESIAN_POINT('Ctrl Pts',(-3.61632703393217,58.2014540866952,-4.85314392082562));
#7211=CARTESIAN_POINT('Ctrl Pts',(-4.22630969876986,58.2107654711745,-4.33234064579157));
#7212=CARTESIAN_POINT('Ctrl Pts',(-5.20060604096146,58.2302727419895,-3.09284641223551));
#7213=CARTESIAN_POINT('Ctrl Pts',(-5.5591352207356,58.2401313235473,-2.38914657610037));
#7214=CARTESIAN_POINT('Ctrl Pts',(-5.9795861406248,58.2588139326938,-0.906068520694137));
#7215=CARTESIAN_POINT('Ctrl Pts',(-6.04615338414096,58.2669142064327,-0.142936563359255));
#7216=CARTESIAN_POINT('Ctrl Pts',(-5.88759600211521,58.2846366202039,1.40264674728406));
#7217=CARTESIAN_POINT('Ctrl Pts',(-5.65034250025109,58.2944161144496,2.16905935577278));
#7218=CARTESIAN_POINT('Ctrl Pts',(-4.9011161956024,58.314009575749,3.54645977198778));
#7219=CARTESIAN_POINT('Ctrl Pts',(-4.40357509149157,58.3236323117353,4.14811455551955));
#7220=CARTESIAN_POINT('Ctrl Pts',(-3.2099264188501,58.3416933616046,5.1273694936731));
#7221=CARTESIAN_POINT('Ctrl Pts',(-2.52572795615392,58.3496783993191,5.49674864765797));
#7222=CARTESIAN_POINT('Ctrl Pts',(-1.03180736684294,58.3683524066855,5.96381579552218));
#7223=CARTESIAN_POINT('Ctrl Pts',(-0.233589182840623,58.3783301339855,6.04790490889298));
#7224=CARTESIAN_POINT('Ctrl Pts',(1.31928168112156,58.3977410197851,5.90291812233691));
#7225=CARTESIAN_POINT('Ctrl Pts',(2.06022289020428,58.4070027848986,5.68686607011341));
#7226=CARTESIAN_POINT('Ctrl Pts',(3.44950256049131,58.4243687807772,4.97352571573904));
#7227=CARTESIAN_POINT('Ctrl Pts',(4.07883956806913,58.4333327305947,4.47192567472073));
#7228=CARTESIAN_POINT('Ctrl Pts',(5.09696837341051,58.4528001027957,3.26142380164731));
#7229=CARTESIAN_POINT('Ctrl Pts',(5.47942654470292,58.4627028299152,2.56746138288995));
#7230=CARTESIAN_POINT('Ctrl Pts',(5.9474986674038,58.4815497550765,1.09669857848434));
#7231=CARTESIAN_POINT('Ctrl Pts',(6.03838547141748,58.4898651117374,0.336708629691644));
#7232=CARTESIAN_POINT('Ctrl Pts',(5.92966814879028,58.5073150461233,-1.21247928523865));
#7233=CARTESIAN_POINT('Ctrl Pts',(5.71722611244321,58.5170169126582,-1.98604585925342));
#7234=CARTESIAN_POINT('Ctrl Pts',(5.01170895965484,58.5366129890372,-3.38892333677217));
#7235=CARTESIAN_POINT('Ctrl Pts',(4.53192741509464,58.5463127945614,-4.00795098574795));
#7236=CARTESIAN_POINT('Ctrl Pts',(3.37083052662181,58.5645509502237,-5.02236003761031));
#7237=CARTESIAN_POINT('Ctrl Pts',(2.70287198424826,58.5724640989679,-5.41119964526751));
#7238=CARTESIAN_POINT('Ctrl Pts',(1.34267769100579,58.5894665276335,-5.88666693746568));
#7239=CARTESIAN_POINT('Ctrl Pts',(0.673269435414399,58.5978341308283,-6.));
#7240=CARTESIAN_POINT('Ctrl Pts',(-9.29811783123569E-15,58.606249998771,
-6.));
#7241=CARTESIAN_POINT('Origin',(0.,50.,0.));
#7242=CARTESIAN_POINT('',(-8.76345566347195E-15,59.1125,-6.));
#7243=CARTESIAN_POINT('',(-2.67351908745917E-14,59.056249998771,-6.));
#7244=CARTESIAN_POINT('',(-7.34788079488412E-16,50.,-6.));
#7245=CARTESIAN_POINT('Ctrl Pts',(-4.9960036108132E-15,59.1125,-6.));
#7246=CARTESIAN_POINT('Ctrl Pts',(0.672701052867484,59.1040912368392,-6.));
#7247=CARTESIAN_POINT('Ctrl Pts',(1.34155536469756,59.0957305579412,-5.88685820339337));
#7248=CARTESIAN_POINT('Ctrl Pts',(2.70138297915581,59.0787327127605,-5.41194792946457));
#7249=CARTESIAN_POINT('Ctrl Pts',(3.36947757384086,59.0708192903467,-5.02327298442946));
#7250=CARTESIAN_POINT('Ctrl Pts',(4.53085258097578,59.0525826236427,-4.00916204852835));
#7251=CARTESIAN_POINT('Ctrl Pts',(5.01078795041768,59.0428834359837,-3.39028028632475));
#7252=CARTESIAN_POINT('Ctrl Pts',(5.71668122894584,59.0232872955114,-1.98761404442142));
#7253=CARTESIAN_POINT('Ctrl Pts',(5.92933561133885,59.0135847241384,-1.21410495830013));
#7254=CARTESIAN_POINT('Ctrl Pts',(6.03847755750431,58.996132443645,0.335054524239836));
#7255=CARTESIAN_POINT('Ctrl Pts',(5.94779882789026,58.9878192630031,1.09506992468099));
#7256=CARTESIAN_POINT('Ctrl Pts',(5.48013577684982,58.9689737276042,2.5659405259635));
#7257=CARTESIAN_POINT('Ctrl Pts',(5.09788218678483,58.9590713368697,3.25998998583337));
#7258=CARTESIAN_POINT('Ctrl Pts',(4.08006393409214,58.9396023325235,4.47082192767438));
#7259=CARTESIAN_POINT('Ctrl Pts',(3.4508003450447,58.930635004313,4.97263730701852));
#7260=CARTESIAN_POINT('Ctrl Pts',(2.06164762259643,58.9132705952824,5.68634721117428));
#7261=CARTESIAN_POINT('Ctrl Pts',(1.32077933349314,58.9040097416686,5.90258078485799));
#7262=CARTESIAN_POINT('Ctrl Pts',(-0.23201437723163,58.8845998202845,6.04796271876271));
#7263=CARTESIAN_POINT('Ctrl Pts',(-1.030232689666,58.8746220913791,5.96408516844816));
#7264=CARTESIAN_POINT('Ctrl Pts',(-2.52429644274422,58.8559462944656,5.49741187861185));
#7265=CARTESIAN_POINT('Ctrl Pts',(-3.20862663585613,58.8479603586346,5.12818906846544));
#7266=CARTESIAN_POINT('Ctrl Pts',(-4.4025341469145,58.8299007399992,4.14921578246961));
#7267=CARTESIAN_POINT('Ctrl Pts',(-4.90021442968027,58.8202786551822,3.54770150620519));
#7268=CARTESIAN_POINT('Ctrl Pts',(-5.64978560785529,58.8006852968284,2.17050971252699));
#7269=CARTESIAN_POINT('Ctrl Pts',(-5.8872359780719,58.7909052251381,1.40415742399703));
#7270=CARTESIAN_POINT('Ctrl Pts',(-6.04619079040954,58.7731806625371,-0.141394930549601));
#7271=CARTESIAN_POINT('Ctrl Pts',(-5.97981672468023,58.7650817790603,-0.904553185256946));
#7272=CARTESIAN_POINT('Ctrl Pts',(-5.55974238367077,58.7464004891878,-2.38772678926996));
#7273=CARTESIAN_POINT('Ctrl Pts',(-5.20140327459709,58.7365422966134,-3.0915004300368));
#7274=CARTESIAN_POINT('Ctrl Pts',(-4.22744511984234,58.7170345666816,-4.33123232759352));
#7275=CARTESIAN_POINT('Ctrl Pts',(-3.61760080633883,58.7077200100792,-4.85219413907));
#7276=CARTESIAN_POINT('Ctrl Pts',(-2.25847727368889,58.690730965921,-5.61072762006748));
#7277=CARTESIAN_POINT('Ctrl Pts',(-1.52817325669471,58.6816021657086,-5.85197840613562));
#7278=CARTESIAN_POINT('Ctrl Pts',(-0.515664031273792,58.6689458003909,-5.98339903275881));
#7279=CARTESIAN_POINT('Ctrl Pts',(-0.257693111406946,58.6657211638926,-6.));
#7280=CARTESIAN_POINT('Ctrl Pts',(5.77315972805081E-14,58.6625,-6.));
#7281=CARTESIAN_POINT('Ctrl Pts',(-8.6389229103645E-15,58.606249998771,
-6.));
#7282=CARTESIAN_POINT('Ctrl Pts',(-0.122167840796238,58.6077770967809,-6.));
#7283=CARTESIAN_POINT('Ctrl Pts',(-0.24446281392826,58.6093057839451,-5.99626881492867));
#7284=CARTESIAN_POINT('Ctrl Pts',(-1.13242499823765,58.620405311249,-5.94189557440023));
#7285=CARTESIAN_POINT('Ctrl Pts',(-1.88209003706895,58.6297761242344,-5.74858786203242));
#7286=CARTESIAN_POINT('Ctrl Pts',(-3.286925598113,58.6473365687475,-5.08108066159058));
#7287=CARTESIAN_POINT('Ctrl Pts',(-3.9252649774435,58.655923449754,-4.60581917418637));
#7288=CARTESIAN_POINT('Ctrl Pts',(-4.98122649564737,58.6751844809384,-3.43622099470862));
#7289=CARTESIAN_POINT('Ctrl Pts',(-5.38876716441984,58.6851229553633,-2.75343776800202));
#7290=CARTESIAN_POINT('Ctrl Pts',(-5.90728745868403,58.7041382468853,-1.29624821084482));
#7291=CARTESIAN_POINT('Ctrl Pts',(-6.02374820107787,58.7127645881171,-0.539197522072843));
#7292=CARTESIAN_POINT('Ctrl Pts',(-5.96693876608166,58.7299246617597,1.01318323723523));
#7293=CARTESIAN_POINT('Ctrl Pts',(-5.7805594195143,58.7395348055697,1.7933241298239));
#7294=CARTESIAN_POINT('Ctrl Pts',(-5.12147213884938,58.7591118583213,3.22125057908729));
#7295=CARTESIAN_POINT('Ctrl Pts',(-4.66080840540443,58.7688821135053,3.85782376226492));
#7296=CARTESIAN_POINT('Ctrl Pts',(-3.53381833581784,58.7872996547863,4.90849532883619));
#7297=CARTESIAN_POINT('Ctrl Pts',(-2.88219839217209,58.7952225188689,5.31734221965164));
#7298=CARTESIAN_POINT('Ctrl Pts',(-1.42550782171891,58.8134311509996,5.88288560888607));
#7299=CARTESIAN_POINT('Ctrl Pts',(-0.629041201384563,58.8233869837537,6.02035799191243));
#7300=CARTESIAN_POINT('Ctrl Pts',(0.940108615079224,58.8430013564595,5.97564886933408));
#7301=CARTESIAN_POINT('Ctrl Pts',(1.69798518433907,58.8524748135753,5.80594902646743));
#7302=CARTESIAN_POINT('Ctrl Pts',(3.11828402566099,58.8702285490918,5.1851233141816));
#7303=CARTESIAN_POINT('Ctrl Pts',(3.76563250801836,58.878517043524,4.73594961054287));
#7304=CARTESIAN_POINT('Ctrl Pts',(4.85877481455106,58.8975607639645,3.60789207585319));
#7305=CARTESIAN_POINT('Ctrl Pts',(5.29123706747589,58.9075236638755,2.93724100270947));
#7306=CARTESIAN_POINT('Ctrl Pts',(5.86054611470443,58.9267020894045,1.49430467168795));
#7307=CARTESIAN_POINT('Ctrl Pts',(6.00262912888888,58.9357246929159,0.739828071058013));
#7308=CARTESIAN_POINT('Ctrl Pts',(5.99718050207131,58.9525922230467,-0.815181852638874));
#7309=CARTESIAN_POINT('Ctrl Pts',(5.83675262210175,58.9621009230984,-1.60093485847068));
#7310=CARTESIAN_POINT('Ctrl Pts',(5.22441553448639,58.9816373541801,-3.05210007514069));
#7311=CARTESIAN_POINT('Ctrl Pts',(4.7832531634121,58.9914672910168,-3.70544553004886));
#7312=CARTESIAN_POINT('Ctrl Pts',(3.69023259964329,59.0100570779767,-4.79164077420985));
#7313=CARTESIAN_POINT('Ctrl Pts',(3.05422553412945,59.0180721795944,-5.22008986623226));
#7314=CARTESIAN_POINT('Ctrl Pts',(1.62445341044163,59.0359443311405,-5.83030169809409));
#7315=CARTESIAN_POINT('Ctrl Pts',(0.838982768159112,59.0457627141691,-5.99394362288408));
#7316=CARTESIAN_POINT('Ctrl Pts',(0.0296581642327382,59.0558792717181,-5.99994503405408));
#7317=CARTESIAN_POINT('Ctrl Pts',(0.0148278070826941,59.0560646511824,-6.));
#7318=CARTESIAN_POINT('Ctrl Pts',(-5.65218389446823E-14,59.056249998771,
-6.));
#7319=CARTESIAN_POINT('Origin',(0.,50.,0.));
#7320=CARTESIAN_POINT('',(-6.82056537037793E-15,59.5625,-6.));
#7321=CARTESIAN_POINT('',(-1.86166850070202E-14,59.506249998771,-6.));
#7322=CARTESIAN_POINT('',(-7.34788079488412E-16,50.,-6.));
#7323=CARTESIAN_POINT('Ctrl Pts',(-5.67635441770116E-14,59.5625,-6.));
#7324=CARTESIAN_POINT('Ctrl Pts',(0.0142972269403468,59.5623212846632,-6.));
#7325=CARTESIAN_POINT('Ctrl Pts',(0.0285968282160099,59.5621425396472,-5.9999488973426));
#7326=CARTESIAN_POINT('Ctrl Pts',(0.837392612400114,59.5520325923449,-5.9941660570088));
#7327=CARTESIAN_POINT('Ctrl Pts',(1.62290717636517,59.5422136602954,-5.83073236561579));
#7328=CARTESIAN_POINT('Ctrl Pts',(3.05285476740338,59.5243393154074,-5.22089374457676));
#7329=CARTESIAN_POINT('Ctrl Pts',(3.68898612233827,59.5163252834728,-4.79260275836969));
#7330=CARTESIAN_POINT('Ctrl Pts',(4.78228266676363,59.4977368696895,-3.7066937003491));
#7331=CARTESIAN_POINT('Ctrl Pts',(5.22360516457189,59.4879073757064,-3.05348160371385));
#7332=CARTESIAN_POINT('Ctrl Pts',(5.83632373739268,59.4683705289908,-1.60249824301388));
#7333=CARTESIAN_POINT('Ctrl Pts',(5.99696223601562,59.4588609656099,-0.816787086981186));
#7334=CARTESIAN_POINT('Ctrl Pts',(6.0028267344566,59.4419910447185,0.738203582127298));
#7335=CARTESIAN_POINT('Ctrl Pts',(5.86095264654097,59.4329720056696,1.4926997107051));
#7336=CARTESIAN_POINT('Ctrl Pts',(5.29205835188024,59.4137948851477,2.93575494784605));
#7337=CARTESIAN_POINT('Ctrl Pts',(4.85979813697018,59.4038321375293,3.60650859949935));
#7338=CARTESIAN_POINT('Ctrl Pts',(3.7669558879038,59.3847866057346,4.73490669818668));
#7339=CARTESIAN_POINT('Ctrl Pts',(3.11968095784071,59.3764960119729,5.18429174793231));
#7340=CARTESIAN_POINT('Ctrl Pts',(1.69950759641262,59.3587438449551,5.80550095706382));
#7341=CARTESIAN_POINT('Ctrl Pts',(0.941695634254267,59.3492711954281,5.97539643738251));
#7342=CARTESIAN_POINT('Ctrl Pts',(-0.627399432048698,59.3296575070993,6.02052625534498));
#7343=CARTESIAN_POINT('Ctrl Pts',(-1.42388046024521,59.3197014942469,5.88327657912861));
#7344=CARTESIAN_POINT('Ctrl Pts',(-2.88073088984782,59.3014908638768,5.31814090999649));
#7345=CARTESIAN_POINT('Ctrl Pts',(-3.53248421704506,59.293568429975,4.90945933911823));
#7346=CARTESIAN_POINT('Ctrl Pts',(-4.65975855504601,59.2751523573231,3.85908756114137));
#7347=CARTESIAN_POINT('Ctrl Pts',(-5.12058362693479,59.2653826456766,3.22265773660764));
#7348=CARTESIAN_POINT('Ctrl Pts',(-5.78006018634094,59.2458053434966,1.79493299632178));
#7349=CARTESIAN_POINT('Ctrl Pts',(-5.96665683265347,59.2361943925425,1.01484300101855));
#7350=CARTESIAN_POINT('Ctrl Pts',(-6.02389751968685,59.2190318862247,-0.537513495724967));
#7351=CARTESIAN_POINT('Ctrl Pts',(-5.90765047541225,59.21040849796,-1.29458719801825));
#7352=CARTESIAN_POINT('Ctrl Pts',(-5.38955293821489,59.1913945918115,-2.75189285876347));
#7353=CARTESIAN_POINT('Ctrl Pts',(-4.98222117445791,59.181456369504,-3.4347734072283));
#7354=CARTESIAN_POINT('Ctrl Pts',(-3.92657290615344,59.162193568645,-4.60471591715926));
#7355=CARTESIAN_POINT('Ctrl Pts',(-3.28830864106957,59.1536038580133,-5.08019633894838));
#7356=CARTESIAN_POINT('Ctrl Pts',(-1.88360262186521,59.1360450327733,-5.74808979396372));
#7357=CARTESIAN_POINT('Ctrl Pts',(-1.13400840618302,59.1266751050772,-5.94159104245208));
#7358=CARTESIAN_POINT('Ctrl Pts',(-0.245540622028225,59.1155692577753,-5.99623585121819));
#7359=CARTESIAN_POINT('Ctrl Pts',(-0.122706315052604,59.1140338289381,-6.));
#7360=CARTESIAN_POINT('Ctrl Pts',(2.15105711021124E-15,59.1125,-6.));
#7361=CARTESIAN_POINT('Ctrl Pts',(-6.89726054048379E-14,59.056249998771,
-6.));
#7362=CARTESIAN_POINT('Ctrl Pts',(-0.757078466779825,59.0657134796057,-5.99999999999999));
#7363=CARTESIAN_POINT('Ctrl Pts',(-1.5075091086108,59.0750938626287,-5.85670543582169));
#7364=CARTESIAN_POINT('Ctrl Pts',(-2.93051707960641,59.0928814622661,-5.29247310863984));
#7365=CARTESIAN_POINT('Ctrl Pts',(-3.58763195986761,59.1009420642367,-4.87104734369159));
#7366=CARTESIAN_POINT('Ctrl Pts',(-4.72000389175098,59.1197409195129,-3.78825871871639));
#7367=CARTESIAN_POINT('Ctrl Pts',(-5.17898245154283,59.1297171122548,-3.13168890336551));
#7368=CARTESIAN_POINT('Ctrl Pts',(-5.80297691642877,59.1490570771964,-1.70540284121377));
#7369=CARTESIAN_POINT('Ctrl Pts',(-5.97269404694987,59.1582532989466,-0.953878495726881));
#7370=CARTESIAN_POINT('Ctrl Pts',(-6.02247403535284,59.1755065785828,0.611170717347984));
#7371=CARTESIAN_POINT('Ctrl Pts',(-5.8868748344451,59.1847221165161,1.4101281919661));
#7372=CARTESIAN_POINT('Ctrl Pts',(-5.31637666959674,59.2043033009837,2.88958326266276));
#7373=CARTESIAN_POINT('Ctrl Pts',(-4.89414615252563,59.2141803842959,3.55821423342768));
#7374=CARTESIAN_POINT('Ctrl Pts',(-3.83345597946988,59.2329280106712,4.67765601799604));
#7375=CARTESIAN_POINT('Ctrl Pts',(-3.21173159001649,59.2411033538958,5.12451161277228));
#7376=CARTESIAN_POINT('Ctrl Pts',(-1.80247080507788,59.2587191137075,5.77773781424917));
#7377=CARTESIAN_POINT('Ctrl Pts',(-1.02245955129053,59.2684692543798,5.96537636458588));
#7378=CARTESIAN_POINT('Ctrl Pts',(0.545294980710786,59.2880661860299,6.0251496297033));
#7379=CARTESIAN_POINT('Ctrl Pts',(1.31763040516511,59.2977203788355,5.90454359843958));
#7380=CARTESIAN_POINT('Ctrl Pts',(2.7681420431286,59.3158517743101,5.37847456800289));
#7381=CARTESIAN_POINT('Ctrl Pts',(3.43357001355883,59.3237988637257,4.98008002023127));
#7382=CARTESIAN_POINT('Ctrl Pts',(4.59824783273638,59.3423841384353,3.93567293560701));
#7383=CARTESIAN_POINT('Ctrl Pts',(5.07917293181446,59.3523609517956,3.29171663034268));
#7384=CARTESIAN_POINT('Ctrl Pts',(5.7487689124623,59.371817815855,1.88095993765699));
#7385=CARTESIAN_POINT('Ctrl Pts',(5.94166691804369,59.3811237893472,1.13268064497309));
#7386=CARTESIAN_POINT('Ctrl Pts',(6.03738680112009,59.3985674690332,-0.423433560740823));
#7387=CARTESIAN_POINT('Ctrl Pts',(5.92857669505086,59.4073718976364,-1.21710085195043));
#7388=CARTESIAN_POINT('Ctrl Pts',(5.41095745138905,59.4267583370531,-2.70909580482084));
#7389=CARTESIAN_POINT('Ctrl Pts',(5.00996844969224,59.4366766566598,-3.39379981592379));
#7390=CARTESIAN_POINT('Ctrl Pts',(3.98494564711651,59.455591315434,-4.54926395852199));
#7391=CARTESIAN_POINT('Ctrl Pts',(3.37837107878886,59.4640203602861,-5.01619205194707));
#7392=CARTESIAN_POINT('Ctrl Pts',(1.99159585454879,59.4813550505891,-5.71529102862413));
#7393=CARTESIAN_POINT('Ctrl Pts',(1.21827663239224,59.4910215408661,-5.92847273746746));
#7394=CARTESIAN_POINT('Ctrl Pts',(0.283980815507459,59.5027002385771,-5.99496518869567));
#7395=CARTESIAN_POINT('Ctrl Pts',(0.141914105176113,59.5044760724562,-6.));
#7396=CARTESIAN_POINT('Ctrl Pts',(5.58580959264532E-15,59.506249998771,
-6.));
#7397=CARTESIAN_POINT('Origin',(0.,50.,0.));
#7398=CARTESIAN_POINT('',(4.70252513239422E-14,60.0125,-6.));
#7399=CARTESIAN_POINT('',(9.17358507812823E-15,59.956249998771,-6.));
#7400=CARTESIAN_POINT('',(-7.34788079488412E-16,50.,-6.));
#7401=CARTESIAN_POINT('Ctrl Pts',(1.25593979660721E-13,60.0125,-6.));
#7402=CARTESIAN_POINT('Ctrl Pts',(0.141303861427478,60.0107337017321,-6.));
#7403=CARTESIAN_POINT('Ctrl Pts',(0.28275939708923,60.0089655075363,-5.99500839542605));
#7404=CARTESIAN_POINT('Ctrl Pts',(1.21646472782204,59.9972941909021,-5.92884491885588));
#7405=CARTESIAN_POINT('Ctrl Pts',(1.98985001429912,59.9876268748211,-5.71589923330053));
#7406=CARTESIAN_POINT('Ctrl Pts',(3.3768361930805,59.9702895475864,-5.01722489047471));
#7407=CARTESIAN_POINT('Ctrl Pts',(3.98355067371114,59.9618632522133,-4.55048488959786));
#7408=CARTESIAN_POINT('Ctrl Pts',(5.00890949512847,59.9429501315784,-3.3953568347903));
#7409=CARTESIAN_POINT('Ctrl Pts',(5.4101001417314,59.9330321483622,-2.71080031785606));
#7410=CARTESIAN_POINT('Ctrl Pts',(5.92821400384472,59.9136438405904,-1.21891834182566));
#7411=CARTESIAN_POINT('Ctrl Pts',(6.03727302740656,59.9048359031446,-0.425202004778042));
#7412=CARTESIAN_POINT('Ctrl Pts',(5.941984771647,59.8873939952832,1.13099772694377));
#7413=CARTESIAN_POINT('Ctrl Pts',(5.74930537817554,59.878089020869,1.87931094451317));
#7414=CARTESIAN_POINT('Ctrl Pts',(5.08013819823912,59.8586331781096,3.29022086176011));
#7415=CARTESIAN_POINT('Ctrl Pts',(4.59941877272792,59.8486563254349,3.93429954442032));
#7416=CARTESIAN_POINT('Ctrl Pts',(3.43504330283706,59.8300690022009,4.97907042506423));
#7417=CARTESIAN_POINT('Ctrl Pts',(2.76969446582647,59.8221211808227,5.37768131640503));
#7418=CARTESIAN_POINT('Ctrl Pts',(1.31931167178715,59.8039913958972,5.90416531854308));
#7419=CARTESIAN_POINT('Ctrl Pts',(0.547032887913016,59.7943379110988,6.02498930154337));
#7420=CARTESIAN_POINT('Ctrl Pts',(-1.02071810657633,59.7747410236677,5.96567468587889));
#7421=CARTESIAN_POINT('Ctrl Pts',(-1.80078484439692,59.7649901894449,5.77826361325989));
#7422=CARTESIAN_POINT('Ctrl Pts',(-3.21024280951409,59.747371964881,5.12544537310256));
#7423=CARTESIAN_POINT('Ctrl Pts',(-3.83210228483935,59.7391984900125,4.67876614903042));
#7424=CARTESIAN_POINT('Ctrl Pts',(-4.89310404940384,59.7204523559613,3.55964211690044));
#7425=CARTESIAN_POINT('Ctrl Pts',(-5.31551858348093,59.7105756824365,2.89115524293708));
#7426=CARTESIAN_POINT('Ctrl Pts',(-5.88648197201678,59.6909928303025,1.41181471683303));
#7427=CARTESIAN_POINT('Ctrl Pts',(-6.02231852752178,59.6817733575495,0.612810360860394));
#7428=CARTESIAN_POINT('Ctrl Pts',(-5.97294095766319,59.6645217620487,-0.9523156149022));
#7429=CARTESIAN_POINT('Ctrl Pts',(-5.80342604329591,59.6553265314883,-1.70386514775027));
#7430=CARTESIAN_POINT('Ctrl Pts',(-5.17983055745436,59.6359876625287,-3.13028031807604));
#7431=CARTESIAN_POINT('Ctrl Pts',(-4.72104466560709,59.6260115176167,-3.78695695198865));
#7432=CARTESIAN_POINT('Ctrl Pts',(-3.58895685794024,59.6072108315944,-4.87007873323313));
#7433=CARTESIAN_POINT('Ctrl Pts',(-2.93191390328915,59.599148923791,-5.29170631182061));
#7434=CARTESIAN_POINT('Ctrl Pts',(-1.50853114673329,59.5813566393341,-5.85650841985951));
#7435=CARTESIAN_POINT('Ctrl Pts',(-0.757598971356276,59.5719699871419,-5.99999999999999));
#7436=CARTESIAN_POINT('Ctrl Pts',(-5.38458166943201E-14,59.5625,-6.));
#7437=CARTESIAN_POINT('Ctrl Pts',(-1.11022302462516E-14,59.506249998771,
-6.));
#7438=CARTESIAN_POINT('Ctrl Pts',(-0.632821030745593,59.5141602616553,-6.));
#7439=CARTESIAN_POINT('Ctrl Pts',(-1.26260761218587,59.5220325939233,-5.89987618500378));
#7440=CARTESIAN_POINT('Ctrl Pts',(-2.59219414404648,59.5386524255716,-5.46486473433232));
#7441=CARTESIAN_POINT('Ctrl Pts',(-3.26657156372886,59.5465592222212,-5.09055264034919));
#7442=CARTESIAN_POINT('Ctrl Pts',(-4.46476645251953,59.5649116492729,-4.08700619016442));
#7443=CARTESIAN_POINT('Ctrl Pts',(-4.96850192192615,59.5748786230998,-3.45712839551428));
#7444=CARTESIAN_POINT('Ctrl Pts',(-5.68582946429178,59.5944397488744,-2.06429824813703));
#7445=CARTESIAN_POINT('Ctrl Pts',(-5.90313907034519,59.6038529506833,-1.32020767195513));
#7446=CARTESIAN_POINT('Ctrl Pts',(-6.04690002280499,59.6214918266984,0.226201473925191));
#7447=CARTESIAN_POINT('Ctrl Pts',(-5.96548004211257,59.629948119708,1.01450799500909));
#7448=CARTESIAN_POINT('Ctrl Pts',(-5.50263475127271,59.6491224173711,2.51852988851507));
#7449=CARTESIAN_POINT('Ctrl Pts',(-5.12431240893829,59.6590721668368,3.21922386751421));
#7450=CARTESIAN_POINT('Ctrl Pts',(-4.13680068949526,59.6781541992168,4.41180635547012));
#7451=CARTESIAN_POINT('Ctrl Pts',(-3.54553027877212,59.6869308702863,4.89962609971964));
#7452=CARTESIAN_POINT('Ctrl Pts',(-2.18217991660048,59.7039727498135,5.64525560222874));
#7453=CARTESIAN_POINT('Ctrl Pts',(-1.41656447760803,59.7135429428009,5.88422844573759));
#7454=CARTESIAN_POINT('Ctrl Pts',(0.148488043825732,59.7331060993188,6.04859188872487));
#7455=CARTESIAN_POINT('Ctrl Pts',(0.932145238599361,59.7429018142535,5.97817898125281));
#7456=CARTESIAN_POINT('Ctrl Pts',(2.41119858669003,59.7613899811046,5.54668031548456));
#7457=CARTESIAN_POINT('Ctrl Pts',(3.09479081689663,59.7693405589739,5.19632631161659));
#7458=CARTESIAN_POINT('Ctrl Pts',(4.32603853610185,59.7874522861142,4.23409782734767));
#7459=CARTESIAN_POINT('Ctrl Pts',(4.85224268738086,59.7973985542548,3.61910504159258));
#7460=CARTESIAN_POINT('Ctrl Pts',(5.61693867228848,59.8170442900147,2.24580714162143));
#7461=CARTESIAN_POINT('Ctrl Pts',(5.85862805091094,59.8265559336545,1.50669856689779));
#7462=CARTESIAN_POINT('Ctrl Pts',(6.05013056294877,59.8443848385756,-0.0297010951204617));
#7463=CARTESIAN_POINT('Ctrl Pts',(5.99534371003816,59.8525791030305,-0.812909405087863));
#7464=CARTESIAN_POINT('Ctrl Pts',(5.586355194442,59.871535107359,-2.32786044779519));
#7465=CARTESIAN_POINT('Ctrl Pts',(5.23095041176157,59.8815044079573,-3.04359194229456));
#7466=CARTESIAN_POINT('Ctrl Pts',(4.28098368544513,59.9007441194128,-4.27241681121637));
#7467=CARTESIAN_POINT('Ctrl Pts',(3.7044839768511,59.909851938227,-4.78091881232232));
#7468=CARTESIAN_POINT('Ctrl Pts',(2.36423147700459,59.9267863723026,-5.5714596822957));
#7469=CARTESIAN_POINT('Ctrl Pts',(1.60679706958879,59.9361650354012,-5.83515225979701));
#7470=CARTESIAN_POINT('Ctrl Pts',(0.547702715938679,59.9494037148218,-5.98126998655213));
#7471=CARTESIAN_POINT('Ctrl Pts',(0.273718776711667,59.9528285140621,-6.));
#7472=CARTESIAN_POINT('Ctrl Pts',(6.08540995372664E-14,59.956249998771,
-6.));
#7473=CARTESIAN_POINT('Origin',(0.,50.,0.));
#7474=CARTESIAN_POINT('',(3.96941465019781E-15,60.4625,-6.));
#7475=CARTESIAN_POINT('',(-2.9927082070389E-14,60.406249998771,-6.));
#7476=CARTESIAN_POINT('',(-7.34788079488412E-16,50.,-6.));
#7477=CARTESIAN_POINT('Ctrl Pts',(5.44009282066327E-14,60.4625,-6.));
#7478=CARTESIAN_POINT('Ctrl Pts',(0.273148046031432,60.4590856494246,-6.));
#7479=CARTESIAN_POINT('Ctrl Pts',(0.54656143924663,60.4556679820094,-5.98134801383603));
#7480=CARTESIAN_POINT('Ctrl Pts',(1.60512629394782,60.4424359213256,-5.83561176679995));
#7481=CARTESIAN_POINT('Ctrl Pts',(2.36263397232493,60.4330536897797,-5.57213696902889));
#7482=CARTESIAN_POINT('Ctrl Pts',(3.70309278914091,60.4161222630287,-4.78199302095628));
#7483=CARTESIAN_POINT('Ctrl Pts',(4.2797245897032,60.407015601891,-4.27367422475566));
#7484=CARTESIAN_POINT('Ctrl Pts',(5.23002905006472,60.3877772352197,-3.04516857252226));
#7485=CARTESIAN_POINT('Ctrl Pts',(5.58564006177245,60.3778080583442,-2.32956757343556));
#7486=CARTESIAN_POINT('Ctrl Pts',(5.99510697394861,60.3588500744187,-0.814709865771511));
#7487=CARTESIAN_POINT('Ctrl Pts',(6.05012927819066,60.3506538419049,-0.0314571757089235));
#7488=CARTESIAN_POINT('Ctrl Pts',(5.85905319689185,60.3328266168241,1.5050335092036));
#7489=CARTESIAN_POINT('Ctrl Pts',(5.61758195090551,60.3233158153094,2.2441902306893));
#7490=CARTESIAN_POINT('Ctrl Pts',(4.85330844088509,60.3036707493072,3.61767017708307));
#7491=CARTESIAN_POINT('Ctrl Pts',(4.32730392870041,60.293724247221,4.23279983549354));
#7492=CARTESIAN_POINT('Ctrl Pts',(3.09635036143289,60.2756103299423,5.19540046477978));
#7493=CARTESIAN_POINT('Ctrl Pts',(2.41284204109846,60.2676605255137,5.54596868127766));
#7494=CARTESIAN_POINT('Ctrl Pts',(0.933915368168958,60.2491739421021,5.97789972053624));
#7495=CARTESIAN_POINT('Ctrl Pts',(0.1503026571044,60.2393787832138,6.04854411681298));
#7496=CARTESIAN_POINT('Ctrl Pts',(-1.41477809332879,60.2198152738334,5.88465836872042));
#7497=CARTESIAN_POINT('Ctrl Pts',(-2.18046716029772,60.2102441604963,5.64591753364946));
#7498=CARTESIAN_POINT('Ctrl Pts',(-3.54403161793187,60.1931996047758,4.90070794687794));
#7499=CARTESIAN_POINT('Ctrl Pts',(-4.13543995211808,60.1844264853552,4.41307932512849));
#7500=CARTESIAN_POINT('Ctrl Pts',(-5.12329644157916,60.1653459517617,3.2208343421969));
#7501=CARTESIAN_POINT('Ctrl Pts',(-5.50182840474064,60.1553964364731,2.52028302020345));
#7502=CARTESIAN_POINT('Ctrl Pts',(-5.96517307028057,60.1362201587863,1.01636653405098));
#7503=CARTESIAN_POINT('Ctrl Pts',(-6.04684129149082,60.1277610588246,0.228011856647941));
#7504=CARTESIAN_POINT('Ctrl Pts',(-5.90352058767477,60.1101239535066,-1.31848789690941));
#7505=CARTESIAN_POINT('Ctrl Pts',(-5.68643532461062,60.100711697856,-2.0626205952178));
#7506=CARTESIAN_POINT('Ctrl Pts',(-4.96954506868888,60.0811514416167,-3.4556228858106));
#7507=CARTESIAN_POINT('Ctrl Pts',(-4.4660178099647,60.071184327976,-4.08563380639988));
#7508=CARTESIAN_POINT('Ctrl Pts',(-3.26812887880239,60.0528297240221,-5.08955799492021));
#7509=CARTESIAN_POINT('Ctrl Pts',(-2.59383484350845,60.0449229355437,-5.46409084992291));
#7510=CARTESIAN_POINT('Ctrl Pts',(-1.26378368350271,60.0282972960437,-5.89968791431417));
#7511=CARTESIAN_POINT('Ctrl Pts',(-0.633415724091756,60.0204176965511,-6.));
#7512=CARTESIAN_POINT('Ctrl Pts',(1.23512311489549E-13,60.0125,-6.));
#7513=CARTESIAN_POINT('Ctrl Pts',(6.39766017940246E-14,59.956249998771,
-6.));
#7514=CARTESIAN_POINT('Ctrl Pts',(-0.504816217535487,59.9625602014901,-6.));
#7515=CARTESIAN_POINT('Ctrl Pts',(-1.008730511896,59.9688591301697,-5.93628708717274));
#7516=CARTESIAN_POINT('Ctrl Pts',(-2.23495289718686,59.9841869099859,-5.61976064930326));
#7517=CARTESIAN_POINT('Ctrl Pts',(-2.92758705550944,59.9922591355636,-5.2920648335774));
#7518=CARTESIAN_POINT('Ctrl Pts',(-4.18209374514919,60.0100264655069,-4.37507897245537));
#7519=CARTESIAN_POINT('Ctrl Pts',(-4.72403710285573,60.0198179136244,-3.78347488288704));
#7520=CARTESIAN_POINT('Ctrl Pts',(-5.53488436650716,60.0394089485369,-2.44187548395896));
#7521=CARTESIAN_POINT('Ctrl Pts',(-5.80315545641587,60.0490179289523,-1.70912228121668));
#7522=CARTESIAN_POINT('Ctrl Pts',(-6.0465703131164,60.067048945809,-0.184023924503232));
#7523=CARTESIAN_POINT('Ctrl Pts',(-6.0201409300119,60.0750538718755,0.593955224774895));
#7524=CARTESIAN_POINT('Ctrl Pts',(-5.66901998337537,60.0937652990181,2.11972305133975));
#7525=CARTESIAN_POINT('Ctrl Pts',(-5.33889794584649,60.1037429188537,2.85082004378456));
#7526=CARTESIAN_POINT('Ctrl Pts',(-4.4305494316801,60.1231333270827,4.11759397032116));
#7527=CARTESIAN_POINT('Ctrl Pts',(-3.87044926128686,60.1323758654756,4.64800911083874));
#7528=CARTESIAN_POINT('Ctrl Pts',(-2.552659102628,60.149708509365,5.48830366644853));
#7529=CARTESIAN_POINT('Ctrl Pts',(-1.80044317137907,60.1587444591288,5.7789253132565));
#7530=CARTESIAN_POINT('Ctrl Pts',(-0.240323360944891,60.1782459567593,6.04627958233635));
#7531=CARTESIAN_POINT('Ctrl Pts',(0.551317277502825,60.1881414647399,6.02588609015704));
#7532=CARTESIAN_POINT('Ctrl Pts',(2.05673048868537,60.2069591298796,5.68730090375562));
#7533=CARTESIAN_POINT('Ctrl Pts',(2.75862633972365,60.2152299829837,5.38196040493909));
#7534=CARTESIAN_POINT('Ctrl Pts',(4.04091497351422,60.2327291587413,4.50578547936514));
#7535=CARTESIAN_POINT('Ctrl Pts',(4.60133380314792,60.2424456885497,3.93176886543798));
#7536=CARTESIAN_POINT('Ctrl Pts',(5.45569031524612,60.26204279983,2.61472823199752));
#7537=CARTESIAN_POINT('Ctrl Pts',(5.74761730637461,60.2717294731965,1.88845580279189));
#7538=CARTESIAN_POINT('Ctrl Pts',(6.03721775271674,60.2899362502433,0.373786677800705));
#7539=CARTESIAN_POINT('Ctrl Pts',(6.03554735569943,60.2978563703102,-0.399853629555168));
#7540=CARTESIAN_POINT('Ctrl Pts',(5.73527461721579,60.3163448718056,-1.93438569360858));
#7541=CARTESIAN_POINT('Ctrl Pts',(5.42789447758374,60.326318871908,-2.67827835028817));
#7542=CARTESIAN_POINT('Ctrl Pts',(4.55732677402955,60.3458218758435,-3.97726618384324));
#7543=CARTESIAN_POINT('Ctrl Pts',(4.01231068105578,60.3551739173839,-4.52650558797703));
#7544=CARTESIAN_POINT('Ctrl Pts',(2.726135453839,60.3727001821279,-5.4029389611706));
#7545=CARTESIAN_POINT('Ctrl Pts',(1.99216620776156,60.381347921174,-5.71444259303174));
#7546=CARTESIAN_POINT('Ctrl Pts',(0.817020770296382,60.3960372391423,-5.95827073896467));
#7547=CARTESIAN_POINT('Ctrl Pts',(0.408553452683297,60.4011430806124,-6.));
#7548=CARTESIAN_POINT('Ctrl Pts',(4.71844785465692E-15,60.406249998771,
-6.));
#7549=CARTESIAN_POINT('Origin',(0.,50.,0.));
#7550=CARTESIAN_POINT('',(-3.71478685391425E-14,60.9125,-6.));
#7551=CARTESIAN_POINT('',(4.03880358923688E-15,60.856249998771,-6.));
#7552=CARTESIAN_POINT('',(-7.34788079488412E-16,50.,-6.));
#7553=CARTESIAN_POINT('Ctrl Pts',(-1.12618248060414E-13,60.9125,-5.99999999999999));
#7554=CARTESIAN_POINT('Ctrl Pts',(0.407899687187211,60.9074012539101,-6.));
#7555=CARTESIAN_POINT('Ctrl Pts',(0.815716773773336,60.9023035403277,-5.95840419235766));
#7556=CARTESIAN_POINT('Ctrl Pts',(1.99037501211202,60.8876203123485,-5.71507748822328));
#7557=CARTESIAN_POINT('Ctrl Pts',(2.72451380599383,60.8789692960728,-5.40376825943217));
#7558=CARTESIAN_POINT('Ctrl Pts',(4.0109879068283,60.8614448350747,-4.52767406390134));
#7559=CARTESIAN_POINT('Ctrl Pts',(4.55614945694963,60.8520937890426,-3.97861060060485));
#7560=CARTESIAN_POINT('Ctrl Pts',(5.4270793932076,60.8325917617613,-2.67992212165016));
#7561=CARTESIAN_POINT('Ctrl Pts',(5.73467668753441,60.8226176794372,-1.93614724397326));
#7562=CARTESIAN_POINT('Ctrl Pts',(6.0354300753238,60.8041270371724,-0.401694927124871));
#7563=CARTESIAN_POINT('Ctrl Pts',(6.03733400582058,60.7962064800698,0.371985158761497));
#7564=CARTESIAN_POINT('Ctrl Pts',(5.74817275039893,60.7780013559698,1.88675515806456));
#7565=CARTESIAN_POINT('Ctrl Pts',(5.45647056996206,60.7683153808155,2.61309288370565));
#7566=CARTESIAN_POINT('Ctrl Pts',(4.60252525073201,60.7487182333133,3.93037426549416));
#7567=CARTESIAN_POINT('Ctrl Pts',(4.04227975119642,60.7390009421187,4.50456128543735));
#7568=CARTESIAN_POINT('Ctrl Pts',(2.76025366510501,60.721499184061,5.38112633567564));
#7569=CARTESIAN_POINT('Ctrl Pts',(2.05844775600324,60.71323059695,5.68667991738853));
#7570=CARTESIAN_POINT('Ctrl Pts',(0.55315772214554,60.6944144715268,6.0257142941801));
#7571=CARTESIAN_POINT('Ctrl Pts',(-0.238451892510666,60.6845193513435,6.04635055945311));
#7572=CARTESIAN_POINT('Ctrl Pts',(-1.79871426147577,60.6650160717315,5.77947524572385));
#7573=CARTESIAN_POINT('Ctrl Pts',(-2.55109564768498,60.6559762829156,5.48904274206938));
#7574=CARTESIAN_POINT('Ctrl Pts',(-3.86916759984809,60.6386453907715,4.64907269931894));
#7575=CARTESIAN_POINT('Ctrl Pts',(-4.42939943296648,60.6294038661924,4.11882722641972));
#7576=CARTESIAN_POINT('Ctrl Pts',(-5.33807972820677,60.6100145454816,2.85234531440023));
#7577=CARTESIAN_POINT('Ctrl Pts',(-5.66840233303937,60.6000369394427,2.12136539403535));
#7578=CARTESIAN_POINT('Ctrl Pts',(-6.01997653921377,60.5813235580555,0.595678731588266));
#7579=CARTESIAN_POINT('Ctrl Pts',(-6.04662719473821,60.5733175290641,-0.1823402310685));
#7580=CARTESIAN_POINT('Ctrl Pts',(-5.80362157445076,60.5552880868231,-1.70752940377283));
#7581=CARTESIAN_POINT('Ctrl Pts',(-5.53556014903915,60.545679832871,-2.44033654855703));
#7582=CARTESIAN_POINT('Ctrl Pts',(-4.72510067103932,60.5260889405219,-3.7821466661943));
#7583=CARTESIAN_POINT('Ctrl Pts',(-4.18332318495113,60.5162968750893,-4.37390354690658));
#7584=CARTESIAN_POINT('Ctrl Pts',(-2.92906424335277,60.4985272003166,-5.29124905149095));
#7585=CARTESIAN_POINT('Ctrl Pts',(-2.23651043720591,60.490456380465,-5.61914254328846));
#7586=CARTESIAN_POINT('Ctrl Pts',(-1.00982889950544,60.4751228612438,-5.93614756202184));
#7587=CARTESIAN_POINT('Ctrl Pts',(-0.505368605494469,60.4688171075687,-6.));
#7588=CARTESIAN_POINT('Ctrl Pts',(6.12010442324618E-14,60.4625,-6.));
#7589=CARTESIAN_POINT('Ctrl Pts',(1.02001740387436E-14,60.406249998771,
-6.));
#7590=CARTESIAN_POINT('Ctrl Pts',(-0.374775140832848,60.4109346880314,-6.));
#7591=CARTESIAN_POINT('Ctrl Pts',(-0.749622762601871,60.4156202833035,-5.96488608497845));
#7592=CARTESIAN_POINT('Ctrl Pts',(-1.8652081247458,60.4295651003303,-5.75300152969955));
#7593=CARTESIAN_POINT('Ctrl Pts',(-2.57723487707561,60.4381304044621,-5.47118475110046));
#7594=CARTESIAN_POINT('Ctrl Pts',(-3.88822754079226,60.4553417616544,-4.63816964510487));
#7595=CARTESIAN_POINT('Ctrl Pts',(-4.46742436471921,60.464968789911,-4.08326231043965));
#7596=CARTESIAN_POINT('Ctrl Pts',(-5.36668868053248,60.4845507847614,-2.79354560554172));
#7597=CARTESIAN_POINT('Ctrl Pts',(-5.68331709127291,60.4943094131409,-2.07488762823363));
#7598=CARTESIAN_POINT('Ctrl Pts',(-6.02124370086058,60.5126958643704,-0.571522036550122));
#7599=CARTESIAN_POINT('Ctrl Pts',(-6.04506729549864,60.520610878074,0.19792028182648));
#7600=CARTESIAN_POINT('Ctrl Pts',(-5.79733980704217,60.5388616662783,1.74083034691086));
#7601=CARTESIAN_POINT('Ctrl Pts',(-5.51393640302953,60.5488211493281,2.49722495048716));
#7602=CARTESIAN_POINT('Ctrl Pts',(-4.68353189440874,60.5684207561163,3.82832480471795));
#7603=CARTESIAN_POINT('Ctrl Pts',(-4.15473832948569,60.5778770003157,4.39655611911274));
#7604=CARTESIAN_POINT('Ctrl Pts',(-2.90124178378718,60.5955974837708,5.30979769390625));
#7605=CARTESIAN_POINT('Ctrl Pts',(-2.18546918107772,60.6039316340075,5.64224146324259));
#7606=CARTESIAN_POINT('Ctrl Pts',(-0.658912830584277,60.6230135883887,6.01578392027695));
#7607=CARTESIAN_POINT('Ctrl Pts',(0.13784785586468,60.6329730969693,6.05019149924373));
#7608=CARTESIAN_POINT('Ctrl Pts',(1.66990313276243,60.6521237879305,5.81289815367829));
#7609=CARTESIAN_POINT('Ctrl Pts',(2.39249044702777,60.6610720459385,5.554665520313));
#7610=CARTESIAN_POINT('Ctrl Pts',(3.73167477624232,60.6779902018836,4.76501165102443));
#7611=CARTESIAN_POINT('Ctrl Pts',(4.32893078259873,60.6875170653545,4.22978361675552));
#7612=CARTESIAN_POINT('Ctrl Pts',(5.27210873015133,60.7070620082945,2.96884316782837));
#7613=CARTESIAN_POINT('Ctrl Pts',(5.61319037689518,60.7168824116893,2.25859674143006));
#7614=CARTESIAN_POINT('Ctrl Pts',(5.99916745926047,60.7354430011218,0.766886905010639));
#7615=CARTESIAN_POINT('Ctrl Pts',(6.04798468727948,60.7434365357459,0.00125250179310366));
#7616=CARTESIAN_POINT('Ctrl Pts',(5.85182540957717,60.7614472214852,-1.54925076800202));
#7617=CARTESIAN_POINT('Ctrl Pts',(5.59237936868007,60.7713818229691,-2.31717870101808));
#7618=CARTESIAN_POINT('Ctrl Pts',(4.80242486574243,60.7910565371578,-3.67857050139044));
#7619=CARTESIAN_POINT('Ctrl Pts',(4.29014923672744,60.8006060031449,-4.26494991040273));
#7620=CARTESIAN_POINT('Ctrl Pts',(3.06873797490042,60.818511480103,-5.21380490027025));
#7621=CARTESIAN_POINT('Ctrl Pts',(2.37017279154696,60.8266228388767,-5.56625543273656));
#7622=CARTESIAN_POINT('Ctrl Pts',(1.09432066564828,60.8425709904504,-5.92495590370132));
#7623=CARTESIAN_POINT('Ctrl Pts',(0.547865501629616,60.8494016800006,-6.));
#7624=CARTESIAN_POINT('Ctrl Pts',(-6.10622663543836E-14,60.8562499987709,
-6.));
#7625=CARTESIAN_POINT('Origin',(0.,50.,0.));
#7626=CARTESIAN_POINT('',(-4.89396513670948E-14,61.3625,-6.));
#7627=CARTESIAN_POINT('',(-1.48002933598712E-14,61.306249998771,-6.));
#7628=CARTESIAN_POINT('',(-7.34788079488412E-16,50.,-6.));
#7629=CARTESIAN_POINT('Ctrl Pts',(-5.87030424270552E-14,61.3625,-6.));
#7630=CARTESIAN_POINT('Ctrl Pts',(0.547256010313519,61.3556592998711,-6.));
#7631=CARTESIAN_POINT('Ctrl Pts',(1.09311032710014,61.3488361209112,-5.92512279942422));
#7632=CARTESIAN_POINT('Ctrl Pts',(2.36853671641672,61.3328932910448,-5.5669593249633));
#7633=CARTESIAN_POINT('Ctrl Pts',(3.0672535886464,61.3247803003645,-5.21468631722413));
#7634=CARTESIAN_POINT('Ctrl Pts',(4.28895308880416,61.3068764604378,-4.26614896431677));
#7635=CARTESIAN_POINT('Ctrl Pts',(4.80137959754346,61.2973277913116,-3.67993027661039));
#7636=CARTESIAN_POINT('Ctrl Pts',(5.59170169867098,61.2776536644745,-2.3188049663686));
#7637=CARTESIAN_POINT('Ctrl Pts',(5.85136464186537,61.2677187928075,-1.55097730351244));
#7638=CARTESIAN_POINT('Ctrl Pts',(6.04798705243048,61.2497059219882,-0.000539574551999683));
#7639=CARTESIAN_POINT('Ctrl Pts',(5.99939436944144,61.2417134657263,0.765127586001477));
#7640=CARTESIAN_POINT('Ctrl Pts',(5.61385165226514,61.2231544295715,2.25694471763481));
#7641=CARTESIAN_POINT('Ctrl Pts',(5.27299041396996,61.2133345401954,2.96727091390557));
#7642=CARTESIAN_POINT('Ctrl Pts',(4.33020581697961,61.1937891634826,4.22847853409));
#7643=CARTESIAN_POINT('Ctrl Pts',(3.73311018750954,61.1842613450504,4.76388737754585));
#7644=CARTESIAN_POINT('Ctrl Pts',(2.39417921764515,61.1673405080427,5.55393518987752));
#7645=CARTESIAN_POINT('Ctrl Pts',(1.67168965651797,61.1583961207065,5.81238209134706));
#7646=CARTESIAN_POINT('Ctrl Pts',(0.139752350124207,61.1392469043765,6.05014450555849));
#7647=CARTESIAN_POINT('Ctrl Pts',(-0.656993188943331,61.1292875851381,6.01599054763202));
#7648=CARTESIAN_POINT('Ctrl Pts',(-2.1837109481026,61.1102036131486,5.64293150348842));
#7649=CARTESIAN_POINT('Ctrl Pts',(-2.89964817697339,61.10186697484,5.31067801891126));
#7650=CARTESIAN_POINT('Ctrl Pts',(-4.15344592677298,61.0841482546054,4.39777322371879));
#7651=CARTESIAN_POINT('Ctrl Pts',(-4.68239184360215,61.074692928492,3.82971467889929));
#7652=CARTESIAN_POINT('Ctrl Pts',(-5.51317144959492,61.0550941196616,2.49890509940508));
#7653=CARTESIAN_POINT('Ctrl Pts',(-5.79679788338461,61.0451344528347,1.7426222855376));
#7654=CARTESIAN_POINT('Ctrl Pts',(-6.04500959707094,61.0268814413336,0.199786408658281));
#7655=CARTESIAN_POINT('Ctrl Pts',(-6.02142071315293,61.0189667699931,-0.569693169468934));
#7656=CARTESIAN_POINT('Ctrl Pts',(-5.68394232834918,61.0005819647083,-2.07316549798162));
#7657=CARTESIAN_POINT('Ctrl Pts',(-5.36754261280559,60.9908239588702,-2.79189800462317));
#7658=CARTESIAN_POINT('Ctrl Pts',(-4.46869156830285,60.971241722063,-4.08187566283363));
#7659=CARTESIAN_POINT('Ctrl Pts',(-3.88966615171452,60.9616138117079,-4.63696344433425));
#7660=CARTESIAN_POINT('Ctrl Pts',(-2.57893806597757,60.9443997520077,-5.47038095148736));
#7661=CARTESIAN_POINT('Ctrl Pts',(-1.8670074758115,60.9358375934475,-5.75241671135876));
#7662=CARTESIAN_POINT('Ctrl Pts',(-0.750876861534743,60.9218859607691,-5.9647682424307));
#7663=CARTESIAN_POINT('Ctrl Pts',(-0.37540344890043,60.9171925431112,-5.99999999999999));
#7664=CARTESIAN_POINT('Ctrl Pts',(-1.36834987785051E-13,60.9125,-6.));
#7665=CARTESIAN_POINT('Ctrl Pts',(-6.57113252700015E-14,60.856249998771,
-6.));
#7666=CARTESIAN_POINT('Ctrl Pts',(-0.241384366345414,60.8592673033503,-6.));
#7667=CARTESIAN_POINT('Ctrl Pts',(-0.483042507482243,60.8622880301145,-5.98543381416668));
#7668=CARTESIAN_POINT('Ctrl Pts',(-1.48088634413119,60.8747610780727,-5.86420003251657));
#7669=CARTESIAN_POINT('Ctrl Pts',(-2.21368102725674,60.8839210116117,-5.62863230028752));
#7670=CARTESIAN_POINT('Ctrl Pts',(-3.57931748887809,60.900991467382,-4.8805142091203));
#7671=CARTESIAN_POINT('Ctrl Pts',(-4.19329126295089,60.9102129319999,-4.36431882558091));
#7672=CARTESIAN_POINT('Ctrl Pts',(-5.17736054272197,60.9297063369937,-3.13174786985753));
#7673=CARTESIAN_POINT('Ctrl Pts',(-5.54138977875599,60.9395759150596,-2.43020767878148));
#7674=CARTESIAN_POINT('Ctrl Pts',(-5.97274844708689,60.9582966042501,-0.949909531091851));
#7675=CARTESIAN_POINT('Ctrl Pts',(-6.04490483620197,60.9664392786842,-0.187529359001643));
#7676=CARTESIAN_POINT('Ctrl Pts',(-5.89783656108435,60.9840994066076,1.35893347045698));
#7677=CARTESIAN_POINT('Ctrl Pts',(-5.66628129051843,60.9938619224954,2.127067560783));
#7678=CARTESIAN_POINT('Ctrl Pts',(-4.92705043276294,61.0134577989134,3.51046195006189));
#7679=CARTESIAN_POINT('Ctrl Pts',(-4.43354966296899,61.0230991102351,4.11616533768471));
#7680=CARTESIAN_POINT('Ctrl Pts',(-3.24738852655604,61.0412014054,5.10355328409652));
#7681=CARTESIAN_POINT('Ctrl Pts',(-2.56698280158148,61.0491627137512,5.47744365620462));
#7682=CARTESIAN_POINT('Ctrl Pts',(-1.07720954505616,61.0677848794577,5.95586496370465));
#7683=CARTESIAN_POINT('Ctrl Pts',(-0.279018307134967,61.0777622699318,6.04606057744179));
#7684=CARTESIAN_POINT('Ctrl Pts',(1.27603635701102,61.0972004532336,5.91248695432248));
#7685=CARTESIAN_POINT('Ctrl Pts',(2.01906250364592,61.1064882800665,5.70168173011325));
#7686=CARTESIAN_POINT('Ctrl Pts',(3.41199186546582,61.1238998970893,4.99899641261455));
#7687=CARTESIAN_POINT('Ctrl Pts',(4.04343943853173,61.1327687624584,4.50358454524063));
#7688=CARTESIAN_POINT('Ctrl Pts',(5.07048391380239,61.1521888498299,3.30259812204962));
#7689=CARTESIAN_POINT('Ctrl Pts',(5.45882490112482,61.1621009426495,2.6111669823951));
#7690=CARTESIAN_POINT('Ctrl Pts',(5.93867573146569,61.1809877182057,1.14352339622535));
#7691=CARTESIAN_POINT('Ctrl Pts',(6.03554840659564,61.1893681387995,0.384255003332309));
#7692=CARTESIAN_POINT('Ctrl Pts',(5.93903175788826,61.2067504862316,-1.16573355860694));
#7693=CARTESIAN_POINT('Ctrl Pts',(5.73269741445749,61.2164317837732,-1.9409263285586));
#7694=CARTESIAN_POINT('Ctrl Pts',(5.03801375396834,61.2360253839997,-3.34982978860118));
#7695=CARTESIAN_POINT('Ctrl Pts',(4.56267011496105,61.2457426558097,-3.97303312990549));
#7696=CARTESIAN_POINT('Ctrl Pts',(3.40957040924791,61.2640234453728,-4.99599770845838));
#7697=CARTESIAN_POINT('Ctrl Pts',(2.74550424329715,61.2719311957298,-5.38956113336518));
#7698=CARTESIAN_POINT('Ctrl Pts',(1.37485673432524,61.2890642895919,-5.88111192017016));
#7699=CARTESIAN_POINT('Ctrl Pts',(0.689573200401228,61.2976303337659,-6.));
#7700=CARTESIAN_POINT('Ctrl Pts',(7.07767178198537E-15,61.306249998771,
-6.));
#7701=CARTESIAN_POINT('Origin',(0.,50.,0.));
#7702=CARTESIAN_POINT('',(-7.34788079488412E-16,73.,-6.));
#7703=CARTESIAN_POINT('Origin',(0.,73.,0.));
#7704=CARTESIAN_POINT('',(-1.33431256400507E-14,62.206249998771,-6.));
#7705=CARTESIAN_POINT('',(-7.34788079488412E-16,50.,-6.));
#7706=CARTESIAN_POINT('',(-3.,62.393749998771,5.19615242270663));
#7707=CARTESIAN_POINT('Ctrl Pts',(-8.60422844084496E-15,62.206249998771,
-6.));
#7708=CARTESIAN_POINT('Ctrl Pts',(-0.616258639618391,62.2139532317662,-6.));
#7709=CARTESIAN_POINT('Ctrl Pts',(-1.22983984371762,62.2216229968174,-5.90504861391718));
#7710=CARTESIAN_POINT('Ctrl Pts',(-2.5464240496641,62.2380802993918,-5.48621753855818));
#7711=CARTESIAN_POINT('Ctrl Pts',(-3.22312814105713,62.2459901750686,-5.11803689285341));
#7712=CARTESIAN_POINT('Ctrl Pts',(-4.42981084459672,62.2642818352613,-4.12500428678142));
#7713=CARTESIAN_POINT('Ctrl Pts',(-4.93932139761823,62.2742445554702,-3.49885367060309));
#7714=CARTESIAN_POINT('Ctrl Pts',(-5.66878983733698,62.2938291823633,-2.11086213324869));
#7715=CARTESIAN_POINT('Ctrl Pts',(-5.89233336963267,62.3032683826333,-1.36796908110026));
#7716=CARTESIAN_POINT('Ctrl Pts',(-6.04832001623241,62.320956297192,0.175911543593013));
#7717=CARTESIAN_POINT('Ctrl Pts',(-5.97377394326822,62.3293374875246,0.962888696203115));
#7718=CARTESIAN_POINT('Ctrl Pts',(-5.53012411876458,62.348228845472,2.45185624599821));
#7719=CARTESIAN_POINT('Ctrl Pts',(-5.16982972712595,62.3579423477225,3.14113508425838));
#7720=CARTESIAN_POINT('Ctrl Pts',(-4.22166673971517,62.3767254531342,4.32882188275267));
#7721=CARTESIAN_POINT('Ctrl Pts',(-3.64876120915662,62.3856404836565,4.82158996396027));
#7722=CARTESIAN_POINT('Ctrl Pts',(-3.,62.393749998771,5.19615242270663));
#7723=CARTESIAN_POINT('',(-3.,62.,5.19615242270663));
#7724=CARTESIAN_POINT('',(-3.,50.,5.19615242270663));
#7725=CARTESIAN_POINT('',(-2.54168010328493E-14,61.8125,-6.));
#7726=CARTESIAN_POINT('Ctrl Pts',(-3.,62.,5.19615242270663));
#7727=CARTESIAN_POINT('Ctrl Pts',(-3.53098416040067,61.993362697995,4.88958857476387));
#7728=CARTESIAN_POINT('Ctrl Pts',(-4.01184980938664,61.986177110606,4.50344035651509));
#7729=CARTESIAN_POINT('Ctrl Pts',(-4.85405966080593,61.9709529731779,3.58334486618095));
#7730=CARTESIAN_POINT('Ctrl Pts',(-5.20541786447774,61.9629893514596,3.0505537568201));
#7731=CARTESIAN_POINT('Ctrl Pts',(-5.79411617403706,61.9452204120402,1.7490145711897));
#7732=CARTESIAN_POINT('Ctrl Pts',(-5.97451271881476,61.9356327682269,0.96749796704209));
#7733=CARTESIAN_POINT('Ctrl Pts',(-6.01945738911264,61.9185397802293,-0.585535810928422));
#7734=CARTESIAN_POINT('Ctrl Pts',(-5.89710840746593,61.9098297568449,-1.34196254642815));
#7735=CARTESIAN_POINT('Ctrl Pts',(-5.36693302400083,61.8907764468428,-2.79593503145085));
#7736=CARTESIAN_POINT('Ctrl Pts',(-4.95364215667331,61.8808313385913,-3.47601118612493));
#7737=CARTESIAN_POINT('Ctrl Pts',(-3.88906935822695,61.8616193564059,-4.63610668819626));
#7738=CARTESIAN_POINT('Ctrl Pts',(-3.24866047005788,61.8531082558757,-5.10534405456059));
#7739=CARTESIAN_POINT('Ctrl Pts',(-1.84025893941671,61.8355032367427,-5.76218771758364));
#7740=CARTESIAN_POINT('Ctrl Pts',(-1.08865709430635,61.8261082136788,-5.95014037299404));
#7741=CARTESIAN_POINT('Ctrl Pts',(-0.214690057248332,61.8151836257155,-5.99712208047878));
#7742=CARTESIAN_POINT('Ctrl Pts',(-0.107293209532287,61.8138411651192,-6.));
#7743=CARTESIAN_POINT('Ctrl Pts',(-1.49186218934005E-15,61.8125,-6.));
#7744=CARTESIAN_POINT('',(3.0510683832643E-14,61.756249998771,-6.));
#7745=CARTESIAN_POINT('',(-7.34788079488412E-16,50.,-6.));
#7746=CARTESIAN_POINT('Ctrl Pts',(6.59194920871187E-14,61.756249998771,
-6.));
#7747=CARTESIAN_POINT('Ctrl Pts',(-0.742391456204802,61.7655298919735,-6.));
#7748=CARTESIAN_POINT('Ctrl Pts',(-1.47865620397113,61.7747332013206,-5.86220905952843));
#7749=CARTESIAN_POINT('Ctrl Pts',(-2.89102875013166,61.7923878581476,-5.31395788022286));
#7750=CARTESIAN_POINT('Ctrl Pts',(-3.55017353252816,61.8004138992099,-4.89821050585146));
#7751=CARTESIAN_POINT('Ctrl Pts',(-4.69053249859411,61.819160949478,-3.8248187388743));
#7752=CARTESIAN_POINT('Ctrl Pts',(-5.15493007592081,61.8291381888529,-3.17128091093427));
#7753=CARTESIAN_POINT('Ctrl Pts',(-5.79015585618769,61.848508488155,-1.74867708355258));
#7754=CARTESIAN_POINT('Ctrl Pts',(-5.96556963804746,61.857732393193,-0.997884428661905));
#7755=CARTESIAN_POINT('Ctrl Pts',(-6.02667359503539,61.8750329475164,0.564993936637363));
#7756=CARTESIAN_POINT('Ctrl Pts',(-5.89773406647016,61.8841401236578,1.36263557514336));
#7757=CARTESIAN_POINT('Ctrl Pts',(-5.3403131920318,61.9036740996705,2.84527989272617));
#7758=CARTESIAN_POINT('Ctrl Pts',(-4.92327593914152,61.9135623679774,3.51794242151836));
#7759=CARTESIAN_POINT('Ctrl Pts',(-3.87135978464613,61.9323517826686,4.64631012732954));
#7760=CARTESIAN_POINT('Ctrl Pts',(-3.25341935648662,61.9405822568149,5.09812450710615));
#7761=CARTESIAN_POINT('Ctrl Pts',(-1.84970608968904,61.9581286726499,5.76278650867087));
#7762=CARTESIAN_POINT('Ctrl Pts',(-1.0712790534765,61.9678590106026,5.9567999023865));
#7763=CARTESIAN_POINT('Ctrl Pts',(0.496519932524449,61.9874564979276,6.0294433272045));
#7764=CARTESIAN_POINT('Ctrl Pts',(1.27041985657347,61.9971302469782,5.91496086919199));
#7765=CARTESIAN_POINT('Ctrl Pts',(2.72453340113302,62.0153066662852,5.40053328082097));
#7766=CARTESIAN_POINT('Ctrl Pts',(3.39218254958916,62.0232359218829,5.0081872966928));
#7767=CARTESIAN_POINT('Ctrl Pts',(4.56530468786986,62.041763606212,3.97397551344385));
#7768=CARTESIAN_POINT('Ctrl Pts',(5.05197530023428,62.0517389691394,3.33347036706901));
#7769=CARTESIAN_POINT('Ctrl Pts',(5.73356113214312,62.0712237843013,1.92705400599191));
#7770=CARTESIAN_POINT('Ctrl Pts',(5.93257678186554,62.0805574372898,1.17974981446382));
#7771=CARTESIAN_POINT('Ctrl Pts',(6.04036429280152,62.0980505239439,-0.373961163281768));
#7772=CARTESIAN_POINT('Ctrl Pts',(5.93849275700343,62.1067595872934,-1.1662630863717));
#7773=CARTESIAN_POINT('Ctrl Pts',(5.43468465290227,62.1260935095028,-2.66138057257977));
#7774=CARTESIAN_POINT('Ctrl Pts',(5.03934834315488,62.136020843486,-3.35018087933003));
#7775=CARTESIAN_POINT('Ctrl Pts',(4.02372723450545,62.1549782617169,-4.51502304185605));
#7776=CARTESIAN_POINT('Ctrl Pts',(3.42104652316216,62.1634869172315,-4.98720673948494));
#7777=CARTESIAN_POINT('Ctrl Pts',(2.04016613534585,62.1807479220792,-5.69812985528455));
#7778=CARTESIAN_POINT('Ctrl Pts',(1.26871736126363,62.1903910317553,-5.9178795864489));
#7779=CARTESIAN_POINT('Ctrl Pts',(0.318012786659299,62.2022748389378,-5.99368644877733));
#7780=CARTESIAN_POINT('Ctrl Pts',(0.158917369613548,62.2042635316508,-6.));
#7781=CARTESIAN_POINT('Ctrl Pts',(3.85108611666851E-15,62.206249998771,
-6.));
#7782=CARTESIAN_POINT('Origin',(-32.5,400.,0.));
#7783=CARTESIAN_POINT('',(-59.,400.,-7.34788079488412E-16));
#7784=CARTESIAN_POINT('Origin',(-65.,400.,0.));
#7785=CARTESIAN_POINT('',(-6.,400.,-7.34788079488412E-16));
#7786=CARTESIAN_POINT('Origin',(-32.5,400.,-7.34788079488412E-16));
#7787=CARTESIAN_POINT('',(-7.34788079488412E-16,400.,-6.));
#7788=CARTESIAN_POINT('Origin',(0.,400.,0.));
#7789=CARTESIAN_POINT('Origin',(0.,400.,0.));
#7790=CARTESIAN_POINT('Origin',(0.,50.,0.));
#7791=CARTESIAN_POINT('Ctrl Pts',(6.10622663543836E-15,61.8125,-6.));
#7792=CARTESIAN_POINT('Ctrl Pts',(0.688977411814208,61.8038877823523,-6.));
#7793=CARTESIAN_POINT('Ctrl Pts',(1.37368130809246,61.7953289836488,-5.88131725249645));
#7794=CARTESIAN_POINT('Ctrl Pts',(2.74394904548484,61.7782006369314,-5.39035779280095));
#7795=CARTESIAN_POINT('Ctrl Pts',(3.40815710417449,61.7702927728126,-4.9969670152711));
#7796=CARTESIAN_POINT('Ctrl Pts',(4.56154971839444,61.7520135386179,-3.97431522630718));
#7797=CARTESIAN_POINT('Ctrl Pts',(5.03705640032906,61.7422968962984,-3.35126416771986));
#7798=CARTESIAN_POINT('Ctrl Pts',(5.73213746210445,61.7227031838196,-1.94257977799593));
#7799=CARTESIAN_POINT('Ctrl Pts',(5.93869556354502,61.7130211226562,-1.16744565442734));
#7800=CARTESIAN_POINT('Ctrl Pts',(6.03565876475735,61.6956362955159,0.382514155933625));
#7801=CARTESIAN_POINT('Ctrl Pts',(5.93900543025488,61.6872583429851,1.14180862592295));
#7802=CARTESIAN_POINT('Ctrl Pts',(5.45958655778069,61.6683730231512,2.60956712921656));
#7803=CARTESIAN_POINT('Ctrl Pts',(5.07146103767517,61.6584612628592,3.30109195134678));
#7804=CARTESIAN_POINT('Ctrl Pts',(4.04474262900941,61.6390394316112,4.50242772158962));
#7805=CARTESIAN_POINT('Ctrl Pts',(3.41337234460338,61.6301671543074,4.99806610932519));
#7806=CARTESIAN_POINT('Ctrl Pts',(2.02057663579492,61.6127572079474,5.70114266691254));
#7807=CARTESIAN_POINT('Ctrl Pts',(1.27762644404909,61.6034703305505,5.91214099373319));
#7808=CARTESIAN_POINT('Ctrl Pts',(-0.277349429259922,61.5840331321342,6.04613437437175));
#7809=CARTESIAN_POINT('Ctrl Pts',(-1.0755424524712,61.5740557193441,5.95616320624175));
#7810=CARTESIAN_POINT('Ctrl Pts',(-2.56546866044858,61.5554316417444,5.47815875028546));
#7811=CARTESIAN_POINT('Ctrl Pts',(-3.24601346560067,61.5474695363786,5.10443414682062));
#7812=CARTESIAN_POINT('Ctrl Pts',(-4.43245037929907,61.5293687549667,4.11734525500654));
#7813=CARTESIAN_POINT('Ctrl Pts',(-4.92610044599073,61.5197281188353,3.51179043539488));
#7814=CARTESIAN_POINT('Ctrl Pts',(-5.66570009904181,61.5001323120866,2.12861540595986));
#7815=CARTESIAN_POINT('Ctrl Pts',(-5.89746535371471,61.4903691614763,1.36054391686906));
#7816=CARTESIAN_POINT('Ctrl Pts',(-6.04495653006948,61.4727067352036,-0.1858870628551));
#7817=CARTESIAN_POINT('Ctrl Pts',(-5.97300603582938,61.4645656973602,-0.948294617575622));
#7818=CARTESIAN_POINT('Ctrl Pts',(-5.54204960566922,61.4458464078274,-2.42869570274489));
#7819=CARTESIAN_POINT('Ctrl Pts',(-5.17822300239504,61.435977225973,-3.13031628345293));
#7820=CARTESIAN_POINT('Ctrl Pts',(-4.19451332156246,61.4164832901239,-4.36314389203058));
#7821=CARTESIAN_POINT('Ctrl Pts',(-3.58068615913608,61.4072585769892,-4.87950974091398));
#7822=CARTESIAN_POINT('Ctrl Pts',(-2.21528057083094,61.3901910071353,-5.62800009733629));
#7823=CARTESIAN_POINT('Ctrl Pts',(-1.48257393769345,61.3810321742211,-5.86377086286194));
#7824=CARTESIAN_POINT('Ctrl Pts',(-0.484205589379722,61.3685525698672,-5.98536355884337));
#7825=CARTESIAN_POINT('Ctrl Pts',(-0.241965785432547,61.3655245723179,-5.99999999999999));
#7826=CARTESIAN_POINT('Ctrl Pts',(-5.16947595841089E-14,61.3625,-6.));
#7827=CARTESIAN_POINT('Ctrl Pts',(-6.10622663543836E-15,61.306249998771,
-6.));
#7828=CARTESIAN_POINT('Ctrl Pts',(-0.106729287314065,61.3075841148624,-6.));
#7829=CARTESIAN_POINT('Ctrl Pts',(-0.213561336024365,61.3089195154713,-5.99715225278892));
#7830=CARTESIAN_POINT('Ctrl Pts',(-1.08699672790714,61.3198374578698,-5.95044658308879));
#7831=CARTESIAN_POINT('Ctrl Pts',(-1.83867125547181,61.3292333894644,-5.76269728108951));
#7832=CARTESIAN_POINT('Ctrl Pts',(-3.24720750700701,61.3468400926086,-5.10625765691735));
#7833=CARTESIAN_POINT('Ctrl Pts',(-3.88769465486627,61.3553484105835,-4.63724778150705));
#7834=CARTESIAN_POINT('Ctrl Pts',(-4.95259234219971,61.3745585271075,-3.47751219654718));
#7835=CARTESIAN_POINT('Ctrl Pts',(-5.36610042809721,61.3845038743489,-2.79753937612737));
#7836=CARTESIAN_POINT('Ctrl Pts',(-5.89671680417622,61.4035586161729,-1.34368923227328));
#7837=CARTESIAN_POINT('Ctrl Pts',(-6.01928846149221,61.4122718915949,-0.587285709085823));
#7838=CARTESIAN_POINT('Ctrl Pts',(-5.97479179086783,61.4293623406106,0.965772180516679));
#7839=CARTESIAN_POINT('Ctrl Pts',(-5.79462130968838,61.4389491237747,1.74733979918368));
#7840=CARTESIAN_POINT('Ctrl Pts',(-5.14667212347327,61.4585184100986,3.18097939841526));
#7841=CARTESIAN_POINT('Ctrl Pts',(-4.69063201614918,61.4683038868726,3.82162814362452));
#7842=CARTESIAN_POINT('Ctrl Pts',(-3.57176476423818,61.4867632037124,4.88084848198775));
#7843=CARTESIAN_POINT('Ctrl Pts',(-2.92393676174351,61.4947007892492,5.29440987983458));
#7844=CARTESIAN_POINT('Ctrl Pts',(-1.47181638804433,61.5128522939204,5.87156040110856));
#7845=CARTESIAN_POINT('Ctrl Pts',(-0.675785202994409,61.5228026837335,6.01537749055857));
#7846=CARTESIAN_POINT('Ctrl Pts',(0.894878139798812,61.5424359755185,5.98266182998687));
#7847=CARTESIAN_POINT('Ctrl Pts',(1.65457406399191,61.5519321745709,5.8185434487954));
#7848=CARTESIAN_POINT('Ctrl Pts',(3.07843482283189,61.5697304340564,5.20863678491256));
#7849=CARTESIAN_POINT('Ctrl Pts',(3.72787513446006,61.5779615974826,4.76546028819511));
#7850=CARTESIAN_POINT('Ctrl Pts',(4.8295240529824,61.596953576703,3.64709369739952));
#7851=CARTESIAN_POINT('Ctrl Pts',(5.26771952899154,61.6069204809008,2.97938280197875));
#7852=CARTESIAN_POINT('Ctrl Pts',(5.84880821080874,61.6261354247843,1.53987402507703));
#7853=CARTESIAN_POINT('Ctrl Pts',(5.99683789175222,61.6352220280806,0.785954543753677));
#7854=CARTESIAN_POINT('Ctrl Pts',(6.00319560631724,61.6521014459291,-0.76962865820642));
#7855=CARTESIAN_POINT('Ctrl Pts',(5.84873891680039,61.661546013429,-1.55659478942117));
#7856=CARTESIAN_POINT('Ctrl Pts',(5.2471890916287,61.6810709743493,-3.01292846685));
#7857=CARTESIAN_POINT('Ctrl Pts',(4.81057265753534,61.6909131689183,-3.67003084050065));
#7858=CARTESIAN_POINT('Ctrl Pts',(3.72536844370213,61.7095416668843,-4.76431482595817));
#7859=CARTESIAN_POINT('Ctrl Pts',(3.09286458348203,61.7175891914774,-5.19723457773832));
#7860=CARTESIAN_POINT('Ctrl Pts',(1.66805983060747,61.7353992508884,-5.81797373615802));
#7861=CARTESIAN_POINT('Ctrl Pts',(0.883852492299125,61.7452018426172,-5.98748960197925));
#7862=CARTESIAN_POINT('Ctrl Pts',(0.0596203085914308,61.7555047449136,-5.99977791256666));
#7863=CARTESIAN_POINT('Ctrl Pts',(0.0298052166963125,61.7558774335623,-6.));
#7864=CARTESIAN_POINT('Ctrl Pts',(5.89017058476163E-14,61.756249998771,
-6.));
#7865=CARTESIAN_POINT('Origin',(1.33761810195802E-14,73.,0.));
#7866=CARTESIAN_POINT('',(1.22739989003476E-14,75.,-9.));
#7867=CARTESIAN_POINT('Origin',(1.33761810195802E-14,75.,0.));
#7868=CARTESIAN_POINT('',(1.22739989003476E-14,73.,-9.));
#7869=CARTESIAN_POINT('',(1.22739989003476E-14,73.,-9.));
#7870=CARTESIAN_POINT('Origin',(1.33761810195802E-14,73.,0.));
#7871=CARTESIAN_POINT('Origin',(0.,50.,0.));
#7872=CARTESIAN_POINT('',(-7.34788079488412E-16,75.,-6.));
#7873=CARTESIAN_POINT('',(-7.34788079488412E-16,50.,-6.));
#7874=CARTESIAN_POINT('Origin',(0.,75.,0.));
#7875=CARTESIAN_POINT('Origin',(-65.,400.,0.));
#7876=CARTESIAN_POINT('Origin',(1.33761810195802E-14,73.,0.));
#7877=CARTESIAN_POINT('Origin',(1.33761810195802E-14,75.,0.));
#7878=CARTESIAN_POINT('Origin',(0.,50.,0.));
#7879=CARTESIAN_POINT('Origin',(5.878215178125,50.0703124996927,0.));
#7880=CARTESIAN_POINT('',(5.75643035625,50.1406249993855,0.));
#7881=CARTESIAN_POINT('',(5.878215178125,50.0703124996927,0.));
#7882=CARTESIAN_POINT('',(5.75643035625,50.2531249993855,0.));
#7883=CARTESIAN_POINT('',(5.75643035625,50.1968749993855,0.));
#7884=CARTESIAN_POINT('',(5.878215178125,50.3234374990782,0.));
#7885=CARTESIAN_POINT('Origin',(-2.96955379453125,62.0351562498464,5.14341804793707));
#7886=CARTESIAN_POINT('',(-3.,62.,5.19615242270663));
#7887=CARTESIAN_POINT('',(-2.878215178125,62.2531249993855,4.9852149236284));
#7888=CARTESIAN_POINT('Ctrl Pts',(5.75643035625,50.1406249993855,0.));
#7889=CARTESIAN_POINT('Ctrl Pts',(5.75643035625,50.1781249993855,-3.32347661575227));
#7890=CARTESIAN_POINT('Ctrl Pts',(2.878215178125,50.2156249993855,-4.9852149236284));
#7891=CARTESIAN_POINT('Ctrl Pts',(4.0700849995221E-16,50.2531249993855,
-6.64695323150454));
#7892=CARTESIAN_POINT('Ctrl Pts',(-2.878215178125,50.2906249993855,-4.9852149236284));
#7893=CARTESIAN_POINT('Ctrl Pts',(-5.75643035625,50.3281249993855,-3.32347661575227));
#7894=CARTESIAN_POINT('Ctrl Pts',(-5.75643035625,50.3656249993855,-7.04959401029622E-16));
#7895=CARTESIAN_POINT('Ctrl Pts',(-5.75643035625,50.4031249993855,3.32347661575227));
#7896=CARTESIAN_POINT('Ctrl Pts',(-2.878215178125,50.4406249993855,4.9852149236284));
#7897=CARTESIAN_POINT('Ctrl Pts',(-1.22102549985663E-15,50.4781249993855,
6.64695323150454));
#7898=CARTESIAN_POINT('Ctrl Pts',(2.878215178125,50.5156249993855,4.98521492362841));
#7899=CARTESIAN_POINT('Ctrl Pts',(5.75643035625,50.5531249993855,3.32347661575227));
#7900=CARTESIAN_POINT('Ctrl Pts',(5.75643035625,50.5906249993855,0.));
#7901=CARTESIAN_POINT('Ctrl Pts',(5.75643035625,50.6281249993855,-3.32347661575227));
#7902=CARTESIAN_POINT('Ctrl Pts',(2.878215178125,50.6656249993855,-4.9852149236284));
#7903=CARTESIAN_POINT('Ctrl Pts',(4.0700849995221E-16,50.7031249993855,
-6.64695323150454));
#7904=CARTESIAN_POINT('Ctrl Pts',(-2.878215178125,50.7406249993855,-4.9852149236284));
#7905=CARTESIAN_POINT('Ctrl Pts',(-5.75643035625,50.7781249993855,-3.32347661575227));
#7906=CARTESIAN_POINT('Ctrl Pts',(-5.75643035625,50.8156249993855,-7.04959401029622E-16));
#7907=CARTESIAN_POINT('Ctrl Pts',(-5.75643035625,50.8531249993855,3.32347661575227));
#7908=CARTESIAN_POINT('Ctrl Pts',(-2.878215178125,50.8906249993855,4.9852149236284));
#7909=CARTESIAN_POINT('Ctrl Pts',(-1.22102549985663E-15,50.9281249993855,
6.64695323150454));
#7910=CARTESIAN_POINT('Ctrl Pts',(2.878215178125,50.9656249993855,4.98521492362841));
#7911=CARTESIAN_POINT('Ctrl Pts',(5.75643035625,51.0031249993855,3.32347661575227));
#7912=CARTESIAN_POINT('Ctrl Pts',(5.75643035625,51.0406249993855,0.));
#7913=CARTESIAN_POINT('Ctrl Pts',(5.75643035625,51.0781249993855,-3.32347661575227));
#7914=CARTESIAN_POINT('Ctrl Pts',(2.878215178125,51.1156249993855,-4.9852149236284));
#7915=CARTESIAN_POINT('Ctrl Pts',(4.0700849995221E-16,51.1531249993855,
-6.64695323150454));
#7916=CARTESIAN_POINT('Ctrl Pts',(-2.878215178125,51.1906249993855,-4.9852149236284));
#7917=CARTESIAN_POINT('Ctrl Pts',(-5.75643035625,51.2281249993855,-3.32347661575227));
#7918=CARTESIAN_POINT('Ctrl Pts',(-5.75643035625,51.2656249993855,-7.04959401029622E-16));
#7919=CARTESIAN_POINT('Ctrl Pts',(-5.75643035625,51.3031249993855,3.32347661575227));
#7920=CARTESIAN_POINT('Ctrl Pts',(-2.878215178125,51.3406249993855,4.9852149236284));
#7921=CARTESIAN_POINT('Ctrl Pts',(-1.22102549985663E-15,51.3781249993855,
6.64695323150454));
#7922=CARTESIAN_POINT('Ctrl Pts',(2.878215178125,51.4156249993855,4.98521492362841));
#7923=CARTESIAN_POINT('Ctrl Pts',(5.75643035625,51.4531249993855,3.32347661575227));
#7924=CARTESIAN_POINT('Ctrl Pts',(5.75643035625,51.4906249993855,0.));
#7925=CARTESIAN_POINT('Ctrl Pts',(5.75643035625,51.5281249993855,-3.32347661575227));
#7926=CARTESIAN_POINT('Ctrl Pts',(2.878215178125,51.5656249993855,-4.9852149236284));
#7927=CARTESIAN_POINT('Ctrl Pts',(4.0700849995221E-16,51.6031249993855,
-6.64695323150454));
#7928=CARTESIAN_POINT('Ctrl Pts',(-2.878215178125,51.6406249993855,-4.9852149236284));
#7929=CARTESIAN_POINT('Ctrl Pts',(-5.75643035625,51.6781249993855,-3.32347661575227));
#7930=CARTESIAN_POINT('Ctrl Pts',(-5.75643035625,51.7156249993855,-7.04959401029622E-16));
#7931=CARTESIAN_POINT('Ctrl Pts',(-5.75643035625,51.7531249993855,3.32347661575227));
#7932=CARTESIAN_POINT('Ctrl Pts',(-2.878215178125,51.7906249993855,4.9852149236284));
#7933=CARTESIAN_POINT('Ctrl Pts',(-1.22102549985663E-15,51.8281249993855,
6.64695323150454));
#7934=CARTESIAN_POINT('Ctrl Pts',(2.878215178125,51.8656249993855,4.98521492362841));
#7935=CARTESIAN_POINT('Ctrl Pts',(5.75643035625,51.9031249993855,3.32347661575227));
#7936=CARTESIAN_POINT('Ctrl Pts',(5.75643035625,51.9406249993855,0.));
#7937=CARTESIAN_POINT('Ctrl Pts',(5.75643035625,51.9781249993855,-3.32347661575227));
#7938=CARTESIAN_POINT('Ctrl Pts',(2.878215178125,52.0156249993855,-4.9852149236284));
#7939=CARTESIAN_POINT('Ctrl Pts',(4.0700849995221E-16,52.0531249993855,
-6.64695323150454));
#7940=CARTESIAN_POINT('Ctrl Pts',(-2.878215178125,52.0906249993855,-4.9852149236284));
#7941=CARTESIAN_POINT('Ctrl Pts',(-5.75643035625,52.1281249993855,-3.32347661575227));
#7942=CARTESIAN_POINT('Ctrl Pts',(-5.75643035625,52.1656249993855,-7.04959401029622E-16));
#7943=CARTESIAN_POINT('Ctrl Pts',(-5.75643035625,52.2031249993855,3.32347661575227));
#7944=CARTESIAN_POINT('Ctrl Pts',(-2.878215178125,52.2406249993855,4.9852149236284));
#7945=CARTESIAN_POINT('Ctrl Pts',(-1.22102549985663E-15,52.2781249993855,
6.64695323150454));
#7946=CARTESIAN_POINT('Ctrl Pts',(2.878215178125,52.3156249993855,4.98521492362841));
#7947=CARTESIAN_POINT('Ctrl Pts',(5.75643035625,52.3531249993855,3.32347661575227));
#7948=CARTESIAN_POINT('Ctrl Pts',(5.75643035625,52.3906249993855,0.));
#7949=CARTESIAN_POINT('Ctrl Pts',(5.75643035625,52.4281249993855,-3.32347661575227));
#7950=CARTESIAN_POINT('Ctrl Pts',(2.878215178125,52.4656249993855,-4.9852149236284));
#7951=CARTESIAN_POINT('Ctrl Pts',(4.0700849995221E-16,52.5031249993855,
-6.64695323150454));
#7952=CARTESIAN_POINT('Ctrl Pts',(-2.878215178125,52.5406249993855,-4.9852149236284));
#7953=CARTESIAN_POINT('Ctrl Pts',(-5.75643035625,52.5781249993855,-3.32347661575227));
#7954=CARTESIAN_POINT('Ctrl Pts',(-5.75643035625,52.6156249993855,-7.04959401029622E-16));
#7955=CARTESIAN_POINT('Ctrl Pts',(-5.75643035625,52.6531249993855,3.32347661575227));
#7956=CARTESIAN_POINT('Ctrl Pts',(-2.878215178125,52.6906249993855,4.9852149236284));
#7957=CARTESIAN_POINT('Ctrl Pts',(-1.22102549985663E-15,52.7281249993855,
6.64695323150454));
#7958=CARTESIAN_POINT('Ctrl Pts',(2.878215178125,52.7656249993855,4.98521492362841));
#7959=CARTESIAN_POINT('Ctrl Pts',(5.75643035625,52.8031249993855,3.32347661575227));
#7960=CARTESIAN_POINT('Ctrl Pts',(5.75643035625,52.8406249993855,0.));
#7961=CARTESIAN_POINT('Ctrl Pts',(5.75643035625,52.8781249993855,-3.32347661575227));
#7962=CARTESIAN_POINT('Ctrl Pts',(2.878215178125,52.9156249993855,-4.9852149236284));
#7963=CARTESIAN_POINT('Ctrl Pts',(4.0700849995221E-16,52.9531249993855,
-6.64695323150454));
#7964=CARTESIAN_POINT('Ctrl Pts',(-2.878215178125,52.9906249993855,-4.9852149236284));
#7965=CARTESIAN_POINT('Ctrl Pts',(-5.75643035625,53.0281249993855,-3.32347661575227));
#7966=CARTESIAN_POINT('Ctrl Pts',(-5.75643035625,53.0656249993855,-7.04959401029622E-16));
#7967=CARTESIAN_POINT('Ctrl Pts',(-5.75643035625,53.1031249993855,3.32347661575227));
#7968=CARTESIAN_POINT('Ctrl Pts',(-2.878215178125,53.1406249993855,4.9852149236284));
#7969=CARTESIAN_POINT('Ctrl Pts',(-1.22102549985663E-15,53.1781249993855,
6.64695323150454));
#7970=CARTESIAN_POINT('Ctrl Pts',(2.878215178125,53.2156249993855,4.98521492362841));
#7971=CARTESIAN_POINT('Ctrl Pts',(5.75643035625,53.2531249993855,3.32347661575227));
#7972=CARTESIAN_POINT('Ctrl Pts',(5.75643035625,53.2906249993855,0.));
#7973=CARTESIAN_POINT('Ctrl Pts',(5.75643035625,53.3281249993855,-3.32347661575227));
#7974=CARTESIAN_POINT('Ctrl Pts',(2.878215178125,53.3656249993855,-4.9852149236284));
#7975=CARTESIAN_POINT('Ctrl Pts',(4.0700849995221E-16,53.4031249993855,
-6.64695323150454));
#7976=CARTESIAN_POINT('Ctrl Pts',(-2.878215178125,53.4406249993855,-4.9852149236284));
#7977=CARTESIAN_POINT('Ctrl Pts',(-5.75643035625,53.4781249993855,-3.32347661575227));
#7978=CARTESIAN_POINT('Ctrl Pts',(-5.75643035625,53.5156249993855,-7.04959401029622E-16));
#7979=CARTESIAN_POINT('Ctrl Pts',(-5.75643035625,53.5531249993855,3.32347661575227));
#7980=CARTESIAN_POINT('Ctrl Pts',(-2.878215178125,53.5906249993855,4.9852149236284));
#7981=CARTESIAN_POINT('Ctrl Pts',(-1.22102549985663E-15,53.6281249993855,
6.64695323150454));
#7982=CARTESIAN_POINT('Ctrl Pts',(2.878215178125,53.6656249993855,4.98521492362841));
#7983=CARTESIAN_POINT('Ctrl Pts',(5.75643035625,53.7031249993855,3.32347661575227));
#7984=CARTESIAN_POINT('Ctrl Pts',(5.75643035625,53.7406249993855,0.));
#7985=CARTESIAN_POINT('Ctrl Pts',(5.75643035625,53.7781249993855,-3.32347661575227));
#7986=CARTESIAN_POINT('Ctrl Pts',(2.878215178125,53.8156249993855,-4.9852149236284));
#7987=CARTESIAN_POINT('Ctrl Pts',(4.0700849995221E-16,53.8531249993855,
-6.64695323150454));
#7988=CARTESIAN_POINT('Ctrl Pts',(-2.878215178125,53.8906249993855,-4.9852149236284));
#7989=CARTESIAN_POINT('Ctrl Pts',(-5.75643035625,53.9281249993855,-3.32347661575227));
#7990=CARTESIAN_POINT('Ctrl Pts',(-5.75643035625,53.9656249993855,-7.04959401029622E-16));
#7991=CARTESIAN_POINT('Ctrl Pts',(-5.75643035625,54.0031249993855,3.32347661575227));
#7992=CARTESIAN_POINT('Ctrl Pts',(-2.878215178125,54.0406249993855,4.9852149236284));
#7993=CARTESIAN_POINT('Ctrl Pts',(-1.22102549985663E-15,54.0781249993855,
6.64695323150454));
#7994=CARTESIAN_POINT('Ctrl Pts',(2.878215178125,54.1156249993855,4.98521492362841));
#7995=CARTESIAN_POINT('Ctrl Pts',(5.75643035625,54.1531249993855,3.32347661575227));
#7996=CARTESIAN_POINT('Ctrl Pts',(5.75643035625,54.1906249993855,0.));
#7997=CARTESIAN_POINT('Ctrl Pts',(5.75643035625,54.2281249993855,-3.32347661575227));
#7998=CARTESIAN_POINT('Ctrl Pts',(2.878215178125,54.2656249993855,-4.9852149236284));
#7999=CARTESIAN_POINT('Ctrl Pts',(4.0700849995221E-16,54.3031249993855,
-6.64695323150454));
#8000=CARTESIAN_POINT('Ctrl Pts',(-2.878215178125,54.3406249993855,-4.9852149236284));
#8001=CARTESIAN_POINT('Ctrl Pts',(-5.75643035625,54.3781249993855,-3.32347661575227));
#8002=CARTESIAN_POINT('Ctrl Pts',(-5.75643035625,54.4156249993855,-7.04959401029622E-16));
#8003=CARTESIAN_POINT('Ctrl Pts',(-5.75643035625,54.4531249993855,3.32347661575227));
#8004=CARTESIAN_POINT('Ctrl Pts',(-2.878215178125,54.4906249993855,4.9852149236284));
#8005=CARTESIAN_POINT('Ctrl Pts',(-1.22102549985663E-15,54.5281249993855,
6.64695323150454));
#8006=CARTESIAN_POINT('Ctrl Pts',(2.878215178125,54.5656249993855,4.98521492362841));
#8007=CARTESIAN_POINT('Ctrl Pts',(5.75643035625,54.6031249993855,3.32347661575227));
#8008=CARTESIAN_POINT('Ctrl Pts',(5.75643035625,54.6406249993855,0.));
#8009=CARTESIAN_POINT('Ctrl Pts',(5.75643035625,54.6781249993855,-3.32347661575227));
#8010=CARTESIAN_POINT('Ctrl Pts',(2.878215178125,54.7156249993855,-4.9852149236284));
#8011=CARTESIAN_POINT('Ctrl Pts',(4.0700849995221E-16,54.7531249993855,
-6.64695323150454));
#8012=CARTESIAN_POINT('Ctrl Pts',(-2.878215178125,54.7906249993855,-4.9852149236284));
#8013=CARTESIAN_POINT('Ctrl Pts',(-5.75643035625,54.8281249993855,-3.32347661575227));
#8014=CARTESIAN_POINT('Ctrl Pts',(-5.75643035625,54.8656249993855,-7.04959401029622E-16));
#8015=CARTESIAN_POINT('Ctrl Pts',(-5.75643035625,54.9031249993855,3.32347661575227));
#8016=CARTESIAN_POINT('Ctrl Pts',(-2.878215178125,54.9406249993855,4.9852149236284));
#8017=CARTESIAN_POINT('Ctrl Pts',(-1.22102549985663E-15,54.9781249993855,
6.64695323150454));
#8018=CARTESIAN_POINT('Ctrl Pts',(2.878215178125,55.0156249993855,4.98521492362841));
#8019=CARTESIAN_POINT('Ctrl Pts',(5.75643035625,55.0531249993855,3.32347661575227));
#8020=CARTESIAN_POINT('Ctrl Pts',(5.75643035625,55.0906249993855,0.));
#8021=CARTESIAN_POINT('Ctrl Pts',(5.75643035625,55.1281249993855,-3.32347661575227));
#8022=CARTESIAN_POINT('Ctrl Pts',(2.878215178125,55.1656249993855,-4.9852149236284));
#8023=CARTESIAN_POINT('Ctrl Pts',(4.0700849995221E-16,55.2031249993855,
-6.64695323150454));
#8024=CARTESIAN_POINT('Ctrl Pts',(-2.878215178125,55.2406249993855,-4.9852149236284));
#8025=CARTESIAN_POINT('Ctrl Pts',(-5.75643035625,55.2781249993855,-3.32347661575227));
#8026=CARTESIAN_POINT('Ctrl Pts',(-5.75643035625,55.3156249993855,-7.04959401029622E-16));
#8027=CARTESIAN_POINT('Ctrl Pts',(-5.75643035625,55.3531249993855,3.32347661575227));
#8028=CARTESIAN_POINT('Ctrl Pts',(-2.878215178125,55.3906249993855,4.9852149236284));
#8029=CARTESIAN_POINT('Ctrl Pts',(-1.22102549985663E-15,55.4281249993855,
6.64695323150454));
#8030=CARTESIAN_POINT('Ctrl Pts',(2.878215178125,55.4656249993855,4.98521492362841));
#8031=CARTESIAN_POINT('Ctrl Pts',(5.75643035625,55.5031249993855,3.32347661575227));
#8032=CARTESIAN_POINT('Ctrl Pts',(5.75643035625,55.5406249993855,0.));
#8033=CARTESIAN_POINT('Ctrl Pts',(5.75643035625,55.5781249993855,-3.32347661575227));
#8034=CARTESIAN_POINT('Ctrl Pts',(2.878215178125,55.6156249993855,-4.9852149236284));
#8035=CARTESIAN_POINT('Ctrl Pts',(4.0700849995221E-16,55.6531249993855,
-6.64695323150454));
#8036=CARTESIAN_POINT('Ctrl Pts',(-2.878215178125,55.6906249993855,-4.9852149236284));
#8037=CARTESIAN_POINT('Ctrl Pts',(-5.75643035625,55.7281249993855,-3.32347661575227));
#8038=CARTESIAN_POINT('Ctrl Pts',(-5.75643035625,55.7656249993855,-7.04959401029622E-16));
#8039=CARTESIAN_POINT('Ctrl Pts',(-5.75643035625,55.8031249993855,3.32347661575227));
#8040=CARTESIAN_POINT('Ctrl Pts',(-2.878215178125,55.8406249993855,4.9852149236284));
#8041=CARTESIAN_POINT('Ctrl Pts',(-1.22102549985663E-15,55.8781249993855,
6.64695323150454));
#8042=CARTESIAN_POINT('Ctrl Pts',(2.878215178125,55.9156249993855,4.98521492362841));
#8043=CARTESIAN_POINT('Ctrl Pts',(5.75643035625,55.9531249993855,3.32347661575227));
#8044=CARTESIAN_POINT('Ctrl Pts',(5.75643035625,55.9906249993855,0.));
#8045=CARTESIAN_POINT('Ctrl Pts',(5.75643035625,56.0281249993855,-3.32347661575227));
#8046=CARTESIAN_POINT('Ctrl Pts',(2.878215178125,56.0656249993855,-4.9852149236284));
#8047=CARTESIAN_POINT('Ctrl Pts',(4.0700849995221E-16,56.1031249993855,
-6.64695323150454));
#8048=CARTESIAN_POINT('Ctrl Pts',(-2.878215178125,56.1406249993855,-4.9852149236284));
#8049=CARTESIAN_POINT('Ctrl Pts',(-5.75643035625,56.1781249993855,-3.32347661575227));
#8050=CARTESIAN_POINT('Ctrl Pts',(-5.75643035625,56.2156249993855,-7.04959401029622E-16));
#8051=CARTESIAN_POINT('Ctrl Pts',(-5.75643035625,56.2531249993855,3.32347661575227));
#8052=CARTESIAN_POINT('Ctrl Pts',(-2.878215178125,56.2906249993855,4.9852149236284));
#8053=CARTESIAN_POINT('Ctrl Pts',(-1.22102549985663E-15,56.3281249993855,
6.64695323150454));
#8054=CARTESIAN_POINT('Ctrl Pts',(2.878215178125,56.3656249993855,4.98521492362841));
#8055=CARTESIAN_POINT('Ctrl Pts',(5.75643035625,56.4031249993855,3.32347661575227));
#8056=CARTESIAN_POINT('Ctrl Pts',(5.75643035625,56.4406249993855,0.));
#8057=CARTESIAN_POINT('Ctrl Pts',(5.75643035625,56.4781249993855,-3.32347661575227));
#8058=CARTESIAN_POINT('Ctrl Pts',(2.878215178125,56.5156249993855,-4.9852149236284));
#8059=CARTESIAN_POINT('Ctrl Pts',(4.0700849995221E-16,56.5531249993855,
-6.64695323150454));
#8060=CARTESIAN_POINT('Ctrl Pts',(-2.878215178125,56.5906249993855,-4.9852149236284));
#8061=CARTESIAN_POINT('Ctrl Pts',(-5.75643035625,56.6281249993855,-3.32347661575227));
#8062=CARTESIAN_POINT('Ctrl Pts',(-5.75643035625,56.6656249993855,-7.04959401029622E-16));
#8063=CARTESIAN_POINT('Ctrl Pts',(-5.75643035625,56.7031249993855,3.32347661575227));
#8064=CARTESIAN_POINT('Ctrl Pts',(-2.878215178125,56.7406249993855,4.9852149236284));
#8065=CARTESIAN_POINT('Ctrl Pts',(-1.22102549985663E-15,56.7781249993855,
6.64695323150454));
#8066=CARTESIAN_POINT('Ctrl Pts',(2.878215178125,56.8156249993855,4.98521492362841));
#8067=CARTESIAN_POINT('Ctrl Pts',(5.75643035625,56.8531249993855,3.32347661575227));
#8068=CARTESIAN_POINT('Ctrl Pts',(5.75643035625,56.8906249993855,0.));
#8069=CARTESIAN_POINT('Ctrl Pts',(5.75643035625,56.9281249993855,-3.32347661575227));
#8070=CARTESIAN_POINT('Ctrl Pts',(2.878215178125,56.9656249993855,-4.9852149236284));
#8071=CARTESIAN_POINT('Ctrl Pts',(4.0700849995221E-16,57.0031249993855,
-6.64695323150454));
#8072=CARTESIAN_POINT('Ctrl Pts',(-2.878215178125,57.0406249993855,-4.9852149236284));
#8073=CARTESIAN_POINT('Ctrl Pts',(-5.75643035625,57.0781249993855,-3.32347661575227));
#8074=CARTESIAN_POINT('Ctrl Pts',(-5.75643035625,57.1156249993855,-7.04959401029622E-16));
#8075=CARTESIAN_POINT('Ctrl Pts',(-5.75643035625,57.1531249993855,3.32347661575227));
#8076=CARTESIAN_POINT('Ctrl Pts',(-2.878215178125,57.1906249993855,4.9852149236284));
#8077=CARTESIAN_POINT('Ctrl Pts',(-1.22102549985663E-15,57.2281249993855,
6.64695323150454));
#8078=CARTESIAN_POINT('Ctrl Pts',(2.878215178125,57.2656249993855,4.98521492362841));
#8079=CARTESIAN_POINT('Ctrl Pts',(5.75643035625,57.3031249993855,3.32347661575227));
#8080=CARTESIAN_POINT('Ctrl Pts',(5.75643035625,57.3406249993855,0.));
#8081=CARTESIAN_POINT('Ctrl Pts',(5.75643035625,57.3781249993855,-3.32347661575227));
#8082=CARTESIAN_POINT('Ctrl Pts',(2.878215178125,57.4156249993855,-4.9852149236284));
#8083=CARTESIAN_POINT('Ctrl Pts',(4.0700849995221E-16,57.4531249993855,
-6.64695323150454));
#8084=CARTESIAN_POINT('Ctrl Pts',(-2.878215178125,57.4906249993855,-4.9852149236284));
#8085=CARTESIAN_POINT('Ctrl Pts',(-5.75643035625,57.5281249993855,-3.32347661575227));
#8086=CARTESIAN_POINT('Ctrl Pts',(-5.75643035625,57.5656249993855,-7.04959401029622E-16));
#8087=CARTESIAN_POINT('Ctrl Pts',(-5.75643035625,57.6031249993855,3.32347661575227));
#8088=CARTESIAN_POINT('Ctrl Pts',(-2.878215178125,57.6406249993855,4.9852149236284));
#8089=CARTESIAN_POINT('Ctrl Pts',(-1.22102549985663E-15,57.6781249993855,
6.64695323150454));
#8090=CARTESIAN_POINT('Ctrl Pts',(2.878215178125,57.7156249993855,4.98521492362841));
#8091=CARTESIAN_POINT('Ctrl Pts',(5.75643035625,57.7531249993855,3.32347661575227));
#8092=CARTESIAN_POINT('Ctrl Pts',(5.75643035625,57.7906249993855,0.));
#8093=CARTESIAN_POINT('Ctrl Pts',(5.75643035625,57.8281249993855,-3.32347661575227));
#8094=CARTESIAN_POINT('Ctrl Pts',(2.878215178125,57.8656249993855,-4.9852149236284));
#8095=CARTESIAN_POINT('Ctrl Pts',(4.0700849995221E-16,57.9031249993855,
-6.64695323150454));
#8096=CARTESIAN_POINT('Ctrl Pts',(-2.878215178125,57.9406249993855,-4.9852149236284));
#8097=CARTESIAN_POINT('Ctrl Pts',(-5.75643035625,57.9781249993855,-3.32347661575227));
#8098=CARTESIAN_POINT('Ctrl Pts',(-5.75643035625,58.0156249993855,-7.04959401029622E-16));
#8099=CARTESIAN_POINT('Ctrl Pts',(-5.75643035625,58.0531249993855,3.32347661575227));
#8100=CARTESIAN_POINT('Ctrl Pts',(-2.878215178125,58.0906249993855,4.9852149236284));
#8101=CARTESIAN_POINT('Ctrl Pts',(-1.22102549985663E-15,58.1281249993855,
6.64695323150454));
#8102=CARTESIAN_POINT('Ctrl Pts',(2.878215178125,58.1656249993855,4.98521492362841));
#8103=CARTESIAN_POINT('Ctrl Pts',(5.75643035625,58.2031249993855,3.32347661575227));
#8104=CARTESIAN_POINT('Ctrl Pts',(5.75643035625,58.2406249993855,0.));
#8105=CARTESIAN_POINT('Ctrl Pts',(5.75643035625,58.2781249993855,-3.32347661575227));
#8106=CARTESIAN_POINT('Ctrl Pts',(2.878215178125,58.3156249993855,-4.9852149236284));
#8107=CARTESIAN_POINT('Ctrl Pts',(4.0700849995221E-16,58.3531249993855,
-6.64695323150454));
#8108=CARTESIAN_POINT('Ctrl Pts',(-2.878215178125,58.3906249993855,-4.9852149236284));
#8109=CARTESIAN_POINT('Ctrl Pts',(-5.75643035625,58.4281249993855,-3.32347661575227));
#8110=CARTESIAN_POINT('Ctrl Pts',(-5.75643035625,58.4656249993855,-7.04959401029622E-16));
#8111=CARTESIAN_POINT('Ctrl Pts',(-5.75643035625,58.5031249993855,3.32347661575227));
#8112=CARTESIAN_POINT('Ctrl Pts',(-2.878215178125,58.5406249993855,4.9852149236284));
#8113=CARTESIAN_POINT('Ctrl Pts',(-1.22102549985663E-15,58.5781249993855,
6.64695323150454));
#8114=CARTESIAN_POINT('Ctrl Pts',(2.878215178125,58.6156249993855,4.98521492362841));
#8115=CARTESIAN_POINT('Ctrl Pts',(5.75643035625,58.6531249993855,3.32347661575227));
#8116=CARTESIAN_POINT('Ctrl Pts',(5.75643035625,58.6906249993855,0.));
#8117=CARTESIAN_POINT('Ctrl Pts',(5.75643035625,58.7281249993855,-3.32347661575227));
#8118=CARTESIAN_POINT('Ctrl Pts',(2.878215178125,58.7656249993855,-4.9852149236284));
#8119=CARTESIAN_POINT('Ctrl Pts',(4.0700849995221E-16,58.8031249993855,
-6.64695323150454));
#8120=CARTESIAN_POINT('Ctrl Pts',(-2.878215178125,58.8406249993855,-4.9852149236284));
#8121=CARTESIAN_POINT('Ctrl Pts',(-5.75643035625,58.8781249993855,-3.32347661575227));
#8122=CARTESIAN_POINT('Ctrl Pts',(-5.75643035625,58.9156249993855,-7.04959401029622E-16));
#8123=CARTESIAN_POINT('Ctrl Pts',(-5.75643035625,58.9531249993855,3.32347661575227));
#8124=CARTESIAN_POINT('Ctrl Pts',(-2.878215178125,58.9906249993855,4.9852149236284));
#8125=CARTESIAN_POINT('Ctrl Pts',(-1.22102549985663E-15,59.0281249993855,
6.64695323150454));
#8126=CARTESIAN_POINT('Ctrl Pts',(2.878215178125,59.0656249993855,4.98521492362841));
#8127=CARTESIAN_POINT('Ctrl Pts',(5.75643035625,59.1031249993855,3.32347661575227));
#8128=CARTESIAN_POINT('Ctrl Pts',(5.75643035625,59.1406249993855,0.));
#8129=CARTESIAN_POINT('Ctrl Pts',(5.75643035625,59.1781249993855,-3.32347661575227));
#8130=CARTESIAN_POINT('Ctrl Pts',(2.878215178125,59.2156249993855,-4.9852149236284));
#8131=CARTESIAN_POINT('Ctrl Pts',(4.0700849995221E-16,59.2531249993855,
-6.64695323150454));
#8132=CARTESIAN_POINT('Ctrl Pts',(-2.878215178125,59.2906249993855,-4.9852149236284));
#8133=CARTESIAN_POINT('Ctrl Pts',(-5.75643035625,59.3281249993855,-3.32347661575227));
#8134=CARTESIAN_POINT('Ctrl Pts',(-5.75643035625,59.3656249993855,-7.04959401029622E-16));
#8135=CARTESIAN_POINT('Ctrl Pts',(-5.75643035625,59.4031249993855,3.32347661575227));
#8136=CARTESIAN_POINT('Ctrl Pts',(-2.878215178125,59.4406249993855,4.9852149236284));
#8137=CARTESIAN_POINT('Ctrl Pts',(-1.22102549985663E-15,59.4781249993855,
6.64695323150454));
#8138=CARTESIAN_POINT('Ctrl Pts',(2.878215178125,59.5156249993855,4.98521492362841));
#8139=CARTESIAN_POINT('Ctrl Pts',(5.75643035625,59.5531249993855,3.32347661575227));
#8140=CARTESIAN_POINT('Ctrl Pts',(5.75643035625,59.5906249993855,0.));
#8141=CARTESIAN_POINT('Ctrl Pts',(5.75643035625,59.6281249993855,-3.32347661575227));
#8142=CARTESIAN_POINT('Ctrl Pts',(2.878215178125,59.6656249993855,-4.9852149236284));
#8143=CARTESIAN_POINT('Ctrl Pts',(4.0700849995221E-16,59.7031249993855,
-6.64695323150454));
#8144=CARTESIAN_POINT('Ctrl Pts',(-2.878215178125,59.7406249993855,-4.9852149236284));
#8145=CARTESIAN_POINT('Ctrl Pts',(-5.75643035625,59.7781249993855,-3.32347661575227));
#8146=CARTESIAN_POINT('Ctrl Pts',(-5.75643035625,59.8156249993855,-7.04959401029622E-16));
#8147=CARTESIAN_POINT('Ctrl Pts',(-5.75643035625,59.8531249993855,3.32347661575227));
#8148=CARTESIAN_POINT('Ctrl Pts',(-2.878215178125,59.8906249993855,4.9852149236284));
#8149=CARTESIAN_POINT('Ctrl Pts',(-1.22102549985663E-15,59.9281249993855,
6.64695323150454));
#8150=CARTESIAN_POINT('Ctrl Pts',(2.878215178125,59.9656249993855,4.98521492362841));
#8151=CARTESIAN_POINT('Ctrl Pts',(5.75643035625,60.0031249993855,3.32347661575227));
#8152=CARTESIAN_POINT('Ctrl Pts',(5.75643035625,60.0406249993855,0.));
#8153=CARTESIAN_POINT('Ctrl Pts',(5.75643035625,60.0781249993855,-3.32347661575227));
#8154=CARTESIAN_POINT('Ctrl Pts',(2.878215178125,60.1156249993855,-4.9852149236284));
#8155=CARTESIAN_POINT('Ctrl Pts',(4.0700849995221E-16,60.1531249993855,
-6.64695323150454));
#8156=CARTESIAN_POINT('Ctrl Pts',(-2.878215178125,60.1906249993855,-4.9852149236284));
#8157=CARTESIAN_POINT('Ctrl Pts',(-5.75643035625,60.2281249993855,-3.32347661575227));
#8158=CARTESIAN_POINT('Ctrl Pts',(-5.75643035625,60.2656249993855,-7.04959401029622E-16));
#8159=CARTESIAN_POINT('Ctrl Pts',(-5.75643035625,60.3031249993855,3.32347661575227));
#8160=CARTESIAN_POINT('Ctrl Pts',(-2.878215178125,60.3406249993855,4.9852149236284));
#8161=CARTESIAN_POINT('Ctrl Pts',(-1.22102549985663E-15,60.3781249993855,
6.64695323150454));
#8162=CARTESIAN_POINT('Ctrl Pts',(2.878215178125,60.4156249993855,4.98521492362841));
#8163=CARTESIAN_POINT('Ctrl Pts',(5.75643035625,60.4531249993855,3.32347661575227));
#8164=CARTESIAN_POINT('Ctrl Pts',(5.75643035625,60.4906249993855,0.));
#8165=CARTESIAN_POINT('Ctrl Pts',(5.75643035625,60.5281249993855,-3.32347661575227));
#8166=CARTESIAN_POINT('Ctrl Pts',(2.878215178125,60.5656249993855,-4.9852149236284));
#8167=CARTESIAN_POINT('Ctrl Pts',(4.0700849995221E-16,60.6031249993855,
-6.64695323150454));
#8168=CARTESIAN_POINT('Ctrl Pts',(-2.878215178125,60.6406249993855,-4.9852149236284));
#8169=CARTESIAN_POINT('Ctrl Pts',(-5.75643035625,60.6781249993855,-3.32347661575227));
#8170=CARTESIAN_POINT('Ctrl Pts',(-5.75643035625,60.7156249993855,-7.04959401029622E-16));
#8171=CARTESIAN_POINT('Ctrl Pts',(-5.75643035625,60.7531249993855,3.32347661575227));
#8172=CARTESIAN_POINT('Ctrl Pts',(-2.878215178125,60.7906249993855,4.9852149236284));
#8173=CARTESIAN_POINT('Ctrl Pts',(-1.22102549985663E-15,60.8281249993855,
6.64695323150454));
#8174=CARTESIAN_POINT('Ctrl Pts',(2.878215178125,60.8656249993855,4.98521492362841));
#8175=CARTESIAN_POINT('Ctrl Pts',(5.75643035625,60.9031249993855,3.32347661575227));
#8176=CARTESIAN_POINT('Ctrl Pts',(5.75643035625,60.9406249993855,0.));
#8177=CARTESIAN_POINT('Ctrl Pts',(5.75643035625,60.9781249993855,-3.32347661575227));
#8178=CARTESIAN_POINT('Ctrl Pts',(2.878215178125,61.0156249993855,-4.9852149236284));
#8179=CARTESIAN_POINT('Ctrl Pts',(4.0700849995221E-16,61.0531249993855,
-6.64695323150454));
#8180=CARTESIAN_POINT('Ctrl Pts',(-2.878215178125,61.0906249993855,-4.9852149236284));
#8181=CARTESIAN_POINT('Ctrl Pts',(-5.75643035625,61.1281249993855,-3.32347661575227));
#8182=CARTESIAN_POINT('Ctrl Pts',(-5.75643035625,61.1656249993855,-7.04959401029622E-16));
#8183=CARTESIAN_POINT('Ctrl Pts',(-5.75643035625,61.2031249993855,3.32347661575227));
#8184=CARTESIAN_POINT('Ctrl Pts',(-2.878215178125,61.2406249993855,4.9852149236284));
#8185=CARTESIAN_POINT('Ctrl Pts',(-1.22102549985663E-15,61.2781249993855,
6.64695323150454));
#8186=CARTESIAN_POINT('Ctrl Pts',(2.878215178125,61.3156249993855,4.98521492362841));
#8187=CARTESIAN_POINT('Ctrl Pts',(5.75643035625,61.3531249993855,3.32347661575227));
#8188=CARTESIAN_POINT('Ctrl Pts',(5.75643035625,61.3906249993855,0.));
#8189=CARTESIAN_POINT('Ctrl Pts',(5.75643035625,61.4281249993855,-3.32347661575227));
#8190=CARTESIAN_POINT('Ctrl Pts',(2.878215178125,61.4656249993855,-4.9852149236284));
#8191=CARTESIAN_POINT('Ctrl Pts',(4.0700849995221E-16,61.5031249993855,
-6.64695323150454));
#8192=CARTESIAN_POINT('Ctrl Pts',(-2.878215178125,61.5406249993855,-4.9852149236284));
#8193=CARTESIAN_POINT('Ctrl Pts',(-5.75643035625,61.5781249993855,-3.32347661575227));
#8194=CARTESIAN_POINT('Ctrl Pts',(-5.75643035625,61.6156249993855,-7.04959401029622E-16));
#8195=CARTESIAN_POINT('Ctrl Pts',(-5.75643035625,61.6531249993855,3.32347661575227));
#8196=CARTESIAN_POINT('Ctrl Pts',(-2.878215178125,61.6906249993855,4.9852149236284));
#8197=CARTESIAN_POINT('Ctrl Pts',(-1.22102549985663E-15,61.7281249993855,
6.64695323150454));
#8198=CARTESIAN_POINT('Ctrl Pts',(2.878215178125,61.7656249993855,4.98521492362841));
#8199=CARTESIAN_POINT('Ctrl Pts',(5.75643035625,61.8031249993855,3.32347661575227));
#8200=CARTESIAN_POINT('Ctrl Pts',(5.75643035625,61.8406249993855,0.));
#8201=CARTESIAN_POINT('Ctrl Pts',(5.75643035625,61.8781249993855,-3.32347661575227));
#8202=CARTESIAN_POINT('Ctrl Pts',(2.878215178125,61.9156249993855,-4.9852149236284));
#8203=CARTESIAN_POINT('Ctrl Pts',(4.0700849995221E-16,61.9531249993855,
-6.64695323150454));
#8204=CARTESIAN_POINT('Ctrl Pts',(-2.878215178125,61.9906249993855,-4.9852149236284));
#8205=CARTESIAN_POINT('Ctrl Pts',(-5.75643035625,62.0281249993855,-3.32347661575227));
#8206=CARTESIAN_POINT('Ctrl Pts',(-5.75643035625,62.0656249993855,-7.04959401029622E-16));
#8207=CARTESIAN_POINT('Ctrl Pts',(-5.75643035625,62.1031249993855,3.32347661575227));
#8208=CARTESIAN_POINT('Ctrl Pts',(-2.878215178125,62.1406249993855,4.9852149236284));
#8209=CARTESIAN_POINT('Ctrl Pts',(6.,50.,0.));
#8210=CARTESIAN_POINT('Ctrl Pts',(6.,50.0375,-3.46410161513775));
#8211=CARTESIAN_POINT('Ctrl Pts',(3.,50.075,-5.19615242270663));
#8212=CARTESIAN_POINT('Ctrl Pts',(4.24230095489963E-16,50.1125,-6.92820323027551));
#8213=CARTESIAN_POINT('Ctrl Pts',(-3.,50.15,-5.19615242270663));
#8214=CARTESIAN_POINT('Ctrl Pts',(-6.,50.1875,-3.46410161513776));
#8215=CARTESIAN_POINT('Ctrl Pts',(-6.,50.225,-7.34788079488412E-16));
#8216=CARTESIAN_POINT('Ctrl Pts',(-6.,50.2625,3.46410161513775));
#8217=CARTESIAN_POINT('Ctrl Pts',(-3.,50.3,5.19615242270663));
#8218=CARTESIAN_POINT('Ctrl Pts',(-1.27269028646989E-15,50.3375,6.92820323027551));
#8219=CARTESIAN_POINT('Ctrl Pts',(3.,50.375,5.19615242270663));
#8220=CARTESIAN_POINT('Ctrl Pts',(6.,50.4125,3.46410161513776));
#8221=CARTESIAN_POINT('Ctrl Pts',(6.,50.45,0.));
#8222=CARTESIAN_POINT('Ctrl Pts',(6.,50.4875,-3.46410161513775));
#8223=CARTESIAN_POINT('Ctrl Pts',(3.,50.525,-5.19615242270663));
#8224=CARTESIAN_POINT('Ctrl Pts',(4.24230095489963E-16,50.5625,-6.92820323027551));
#8225=CARTESIAN_POINT('Ctrl Pts',(-3.,50.6,-5.19615242270663));
#8226=CARTESIAN_POINT('Ctrl Pts',(-6.,50.6375,-3.46410161513776));
#8227=CARTESIAN_POINT('Ctrl Pts',(-6.,50.675,-7.34788079488412E-16));
#8228=CARTESIAN_POINT('Ctrl Pts',(-6.,50.7125,3.46410161513775));
#8229=CARTESIAN_POINT('Ctrl Pts',(-3.,50.75,5.19615242270663));
#8230=CARTESIAN_POINT('Ctrl Pts',(-1.27269028646989E-15,50.7875,6.92820323027551));
#8231=CARTESIAN_POINT('Ctrl Pts',(3.,50.825,5.19615242270663));
#8232=CARTESIAN_POINT('Ctrl Pts',(6.,50.8625,3.46410161513776));
#8233=CARTESIAN_POINT('Ctrl Pts',(6.,50.9,0.));
#8234=CARTESIAN_POINT('Ctrl Pts',(6.,50.9375,-3.46410161513775));
#8235=CARTESIAN_POINT('Ctrl Pts',(3.,50.975,-5.19615242270663));
#8236=CARTESIAN_POINT('Ctrl Pts',(4.24230095489963E-16,51.0125,-6.92820323027551));
#8237=CARTESIAN_POINT('Ctrl Pts',(-3.,51.05,-5.19615242270663));
#8238=CARTESIAN_POINT('Ctrl Pts',(-6.,51.0875,-3.46410161513776));
#8239=CARTESIAN_POINT('Ctrl Pts',(-6.,51.125,-7.34788079488412E-16));
#8240=CARTESIAN_POINT('Ctrl Pts',(-6.,51.1625,3.46410161513775));
#8241=CARTESIAN_POINT('Ctrl Pts',(-3.,51.2,5.19615242270663));
#8242=CARTESIAN_POINT('Ctrl Pts',(-1.27269028646989E-15,51.2375,6.92820323027551));
#8243=CARTESIAN_POINT('Ctrl Pts',(3.,51.275,5.19615242270663));
#8244=CARTESIAN_POINT('Ctrl Pts',(6.,51.3125,3.46410161513776));
#8245=CARTESIAN_POINT('Ctrl Pts',(6.,51.35,0.));
#8246=CARTESIAN_POINT('Ctrl Pts',(6.,51.3875,-3.46410161513775));
#8247=CARTESIAN_POINT('Ctrl Pts',(3.,51.425,-5.19615242270663));
#8248=CARTESIAN_POINT('Ctrl Pts',(4.24230095489963E-16,51.4625,-6.92820323027551));
#8249=CARTESIAN_POINT('Ctrl Pts',(-3.,51.5,-5.19615242270663));
#8250=CARTESIAN_POINT('Ctrl Pts',(-6.,51.5375,-3.46410161513776));
#8251=CARTESIAN_POINT('Ctrl Pts',(-6.,51.575,-7.34788079488412E-16));
#8252=CARTESIAN_POINT('Ctrl Pts',(-6.,51.6125,3.46410161513775));
#8253=CARTESIAN_POINT('Ctrl Pts',(-3.,51.65,5.19615242270663));
#8254=CARTESIAN_POINT('Ctrl Pts',(-1.27269028646989E-15,51.6875,6.92820323027551));
#8255=CARTESIAN_POINT('Ctrl Pts',(3.,51.725,5.19615242270663));
#8256=CARTESIAN_POINT('Ctrl Pts',(6.,51.7625,3.46410161513776));
#8257=CARTESIAN_POINT('Ctrl Pts',(6.,51.8,0.));
#8258=CARTESIAN_POINT('Ctrl Pts',(6.,51.8375,-3.46410161513775));
#8259=CARTESIAN_POINT('Ctrl Pts',(3.,51.875,-5.19615242270663));
#8260=CARTESIAN_POINT('Ctrl Pts',(4.24230095489963E-16,51.9125,-6.92820323027551));
#8261=CARTESIAN_POINT('Ctrl Pts',(-3.,51.95,-5.19615242270663));
#8262=CARTESIAN_POINT('Ctrl Pts',(-6.,51.9875,-3.46410161513776));
#8263=CARTESIAN_POINT('Ctrl Pts',(-6.,52.025,-7.34788079488412E-16));
#8264=CARTESIAN_POINT('Ctrl Pts',(-6.,52.0625,3.46410161513775));
#8265=CARTESIAN_POINT('Ctrl Pts',(-3.,52.1,5.19615242270663));
#8266=CARTESIAN_POINT('Ctrl Pts',(-1.27269028646989E-15,52.1375,6.92820323027551));
#8267=CARTESIAN_POINT('Ctrl Pts',(3.,52.175,5.19615242270663));
#8268=CARTESIAN_POINT('Ctrl Pts',(6.,52.2125,3.46410161513776));
#8269=CARTESIAN_POINT('Ctrl Pts',(6.,52.25,0.));
#8270=CARTESIAN_POINT('Ctrl Pts',(6.,52.2875,-3.46410161513775));
#8271=CARTESIAN_POINT('Ctrl Pts',(3.,52.325,-5.19615242270663));
#8272=CARTESIAN_POINT('Ctrl Pts',(4.24230095489963E-16,52.3625,-6.92820323027551));
#8273=CARTESIAN_POINT('Ctrl Pts',(-3.,52.4,-5.19615242270663));
#8274=CARTESIAN_POINT('Ctrl Pts',(-6.,52.4375,-3.46410161513776));
#8275=CARTESIAN_POINT('Ctrl Pts',(-6.,52.475,-7.34788079488412E-16));
#8276=CARTESIAN_POINT('Ctrl Pts',(-6.,52.5125,3.46410161513775));
#8277=CARTESIAN_POINT('Ctrl Pts',(-3.,52.55,5.19615242270663));
#8278=CARTESIAN_POINT('Ctrl Pts',(-1.27269028646989E-15,52.5875,6.92820323027551));
#8279=CARTESIAN_POINT('Ctrl Pts',(3.,52.625,5.19615242270663));
#8280=CARTESIAN_POINT('Ctrl Pts',(6.,52.6625,3.46410161513776));
#8281=CARTESIAN_POINT('Ctrl Pts',(6.,52.7,0.));
#8282=CARTESIAN_POINT('Ctrl Pts',(6.,52.7375,-3.46410161513775));
#8283=CARTESIAN_POINT('Ctrl Pts',(3.,52.775,-5.19615242270663));
#8284=CARTESIAN_POINT('Ctrl Pts',(4.24230095489963E-16,52.8125,-6.92820323027551));
#8285=CARTESIAN_POINT('Ctrl Pts',(-3.,52.85,-5.19615242270663));
#8286=CARTESIAN_POINT('Ctrl Pts',(-6.,52.8875,-3.46410161513776));
#8287=CARTESIAN_POINT('Ctrl Pts',(-6.,52.925,-7.34788079488412E-16));
#8288=CARTESIAN_POINT('Ctrl Pts',(-6.,52.9625,3.46410161513775));
#8289=CARTESIAN_POINT('Ctrl Pts',(-3.,53.,5.19615242270663));
#8290=CARTESIAN_POINT('Ctrl Pts',(-1.27269028646989E-15,53.0375,6.92820323027551));
#8291=CARTESIAN_POINT('Ctrl Pts',(3.,53.075,5.19615242270663));
#8292=CARTESIAN_POINT('Ctrl Pts',(6.,53.1125,3.46410161513776));
#8293=CARTESIAN_POINT('Ctrl Pts',(6.,53.15,0.));
#8294=CARTESIAN_POINT('Ctrl Pts',(6.,53.1875,-3.46410161513775));
#8295=CARTESIAN_POINT('Ctrl Pts',(3.,53.225,-5.19615242270663));
#8296=CARTESIAN_POINT('Ctrl Pts',(4.24230095489963E-16,53.2625,-6.92820323027551));
#8297=CARTESIAN_POINT('Ctrl Pts',(-3.,53.3,-5.19615242270663));
#8298=CARTESIAN_POINT('Ctrl Pts',(-6.,53.3375,-3.46410161513776));
#8299=CARTESIAN_POINT('Ctrl Pts',(-6.,53.375,-7.34788079488412E-16));
#8300=CARTESIAN_POINT('Ctrl Pts',(-6.,53.4125,3.46410161513775));
#8301=CARTESIAN_POINT('Ctrl Pts',(-3.,53.45,5.19615242270663));
#8302=CARTESIAN_POINT('Ctrl Pts',(-1.27269028646989E-15,53.4875,6.92820323027551));
#8303=CARTESIAN_POINT('Ctrl Pts',(3.,53.525,5.19615242270663));
#8304=CARTESIAN_POINT('Ctrl Pts',(6.,53.5625,3.46410161513776));
#8305=CARTESIAN_POINT('Ctrl Pts',(6.,53.6,0.));
#8306=CARTESIAN_POINT('Ctrl Pts',(6.,53.6375,-3.46410161513775));
#8307=CARTESIAN_POINT('Ctrl Pts',(3.,53.675,-5.19615242270663));
#8308=CARTESIAN_POINT('Ctrl Pts',(4.24230095489963E-16,53.7125,-6.92820323027551));
#8309=CARTESIAN_POINT('Ctrl Pts',(-3.,53.75,-5.19615242270663));
#8310=CARTESIAN_POINT('Ctrl Pts',(-6.,53.7875,-3.46410161513776));
#8311=CARTESIAN_POINT('Ctrl Pts',(-6.,53.825,-7.34788079488412E-16));
#8312=CARTESIAN_POINT('Ctrl Pts',(-6.,53.8625,3.46410161513775));
#8313=CARTESIAN_POINT('Ctrl Pts',(-3.,53.9,5.19615242270663));
#8314=CARTESIAN_POINT('Ctrl Pts',(-1.27269028646989E-15,53.9375,6.92820323027551));
#8315=CARTESIAN_POINT('Ctrl Pts',(3.,53.975,5.19615242270663));
#8316=CARTESIAN_POINT('Ctrl Pts',(6.,54.0125,3.46410161513776));
#8317=CARTESIAN_POINT('Ctrl Pts',(6.,54.05,0.));
#8318=CARTESIAN_POINT('Ctrl Pts',(6.,54.0875,-3.46410161513775));
#8319=CARTESIAN_POINT('Ctrl Pts',(3.,54.125,-5.19615242270663));
#8320=CARTESIAN_POINT('Ctrl Pts',(4.24230095489963E-16,54.1625,-6.92820323027551));
#8321=CARTESIAN_POINT('Ctrl Pts',(-3.,54.2,-5.19615242270663));
#8322=CARTESIAN_POINT('Ctrl Pts',(-6.,54.2375,-3.46410161513776));
#8323=CARTESIAN_POINT('Ctrl Pts',(-6.,54.275,-7.34788079488412E-16));
#8324=CARTESIAN_POINT('Ctrl Pts',(-6.,54.3125,3.46410161513775));
#8325=CARTESIAN_POINT('Ctrl Pts',(-3.,54.35,5.19615242270663));
#8326=CARTESIAN_POINT('Ctrl Pts',(-1.27269028646989E-15,54.3875,6.92820323027551));
#8327=CARTESIAN_POINT('Ctrl Pts',(3.,54.425,5.19615242270663));
#8328=CARTESIAN_POINT('Ctrl Pts',(6.,54.4625,3.46410161513776));
#8329=CARTESIAN_POINT('Ctrl Pts',(6.,54.5,0.));
#8330=CARTESIAN_POINT('Ctrl Pts',(6.,54.5375,-3.46410161513775));
#8331=CARTESIAN_POINT('Ctrl Pts',(3.,54.575,-5.19615242270663));
#8332=CARTESIAN_POINT('Ctrl Pts',(4.24230095489963E-16,54.6125,-6.92820323027551));
#8333=CARTESIAN_POINT('Ctrl Pts',(-3.,54.65,-5.19615242270663));
#8334=CARTESIAN_POINT('Ctrl Pts',(-6.,54.6875,-3.46410161513776));
#8335=CARTESIAN_POINT('Ctrl Pts',(-6.,54.725,-7.34788079488412E-16));
#8336=CARTESIAN_POINT('Ctrl Pts',(-6.,54.7625,3.46410161513775));
#8337=CARTESIAN_POINT('Ctrl Pts',(-3.,54.8,5.19615242270663));
#8338=CARTESIAN_POINT('Ctrl Pts',(-1.27269028646989E-15,54.8375,6.92820323027551));
#8339=CARTESIAN_POINT('Ctrl Pts',(3.,54.875,5.19615242270663));
#8340=CARTESIAN_POINT('Ctrl Pts',(6.,54.9125,3.46410161513776));
#8341=CARTESIAN_POINT('Ctrl Pts',(6.,54.95,0.));
#8342=CARTESIAN_POINT('Ctrl Pts',(6.,54.9875,-3.46410161513775));
#8343=CARTESIAN_POINT('Ctrl Pts',(3.,55.025,-5.19615242270663));
#8344=CARTESIAN_POINT('Ctrl Pts',(4.24230095489963E-16,55.0625,-6.92820323027551));
#8345=CARTESIAN_POINT('Ctrl Pts',(-3.,55.1,-5.19615242270663));
#8346=CARTESIAN_POINT('Ctrl Pts',(-6.,55.1375,-3.46410161513776));
#8347=CARTESIAN_POINT('Ctrl Pts',(-6.,55.175,-7.34788079488412E-16));
#8348=CARTESIAN_POINT('Ctrl Pts',(-6.,55.2125,3.46410161513775));
#8349=CARTESIAN_POINT('Ctrl Pts',(-3.,55.25,5.19615242270663));
#8350=CARTESIAN_POINT('Ctrl Pts',(-1.27269028646989E-15,55.2875,6.92820323027551));
#8351=CARTESIAN_POINT('Ctrl Pts',(3.,55.325,5.19615242270663));
#8352=CARTESIAN_POINT('Ctrl Pts',(6.,55.3625,3.46410161513776));
#8353=CARTESIAN_POINT('Ctrl Pts',(6.,55.4,0.));
#8354=CARTESIAN_POINT('Ctrl Pts',(6.,55.4375,-3.46410161513775));
#8355=CARTESIAN_POINT('Ctrl Pts',(3.,55.475,-5.19615242270663));
#8356=CARTESIAN_POINT('Ctrl Pts',(4.24230095489963E-16,55.5125,-6.92820323027551));
#8357=CARTESIAN_POINT('Ctrl Pts',(-3.,55.55,-5.19615242270663));
#8358=CARTESIAN_POINT('Ctrl Pts',(-6.,55.5875,-3.46410161513776));
#8359=CARTESIAN_POINT('Ctrl Pts',(-6.,55.625,-7.34788079488412E-16));
#8360=CARTESIAN_POINT('Ctrl Pts',(-6.,55.6625,3.46410161513775));
#8361=CARTESIAN_POINT('Ctrl Pts',(-3.,55.7,5.19615242270663));
#8362=CARTESIAN_POINT('Ctrl Pts',(-1.27269028646989E-15,55.7375,6.92820323027551));
#8363=CARTESIAN_POINT('Ctrl Pts',(3.,55.775,5.19615242270663));
#8364=CARTESIAN_POINT('Ctrl Pts',(6.,55.8125,3.46410161513776));
#8365=CARTESIAN_POINT('Ctrl Pts',(6.,55.85,0.));
#8366=CARTESIAN_POINT('Ctrl Pts',(6.,55.8875,-3.46410161513775));
#8367=CARTESIAN_POINT('Ctrl Pts',(3.,55.925,-5.19615242270663));
#8368=CARTESIAN_POINT('Ctrl Pts',(4.24230095489963E-16,55.9625,-6.92820323027551));
#8369=CARTESIAN_POINT('Ctrl Pts',(-3.,56.,-5.19615242270663));
#8370=CARTESIAN_POINT('Ctrl Pts',(-6.,56.0375,-3.46410161513776));
#8371=CARTESIAN_POINT('Ctrl Pts',(-6.,56.075,-7.34788079488412E-16));
#8372=CARTESIAN_POINT('Ctrl Pts',(-6.,56.1125,3.46410161513775));
#8373=CARTESIAN_POINT('Ctrl Pts',(-3.,56.15,5.19615242270663));
#8374=CARTESIAN_POINT('Ctrl Pts',(-1.27269028646989E-15,56.1875,6.92820323027551));
#8375=CARTESIAN_POINT('Ctrl Pts',(3.,56.225,5.19615242270663));
#8376=CARTESIAN_POINT('Ctrl Pts',(6.,56.2625,3.46410161513776));
#8377=CARTESIAN_POINT('Ctrl Pts',(6.,56.3,0.));
#8378=CARTESIAN_POINT('Ctrl Pts',(6.,56.3375,-3.46410161513775));
#8379=CARTESIAN_POINT('Ctrl Pts',(3.,56.375,-5.19615242270663));
#8380=CARTESIAN_POINT('Ctrl Pts',(4.24230095489963E-16,56.4125,-6.92820323027551));
#8381=CARTESIAN_POINT('Ctrl Pts',(-3.,56.45,-5.19615242270663));
#8382=CARTESIAN_POINT('Ctrl Pts',(-6.,56.4875,-3.46410161513776));
#8383=CARTESIAN_POINT('Ctrl Pts',(-6.,56.525,-7.34788079488412E-16));
#8384=CARTESIAN_POINT('Ctrl Pts',(-6.,56.5625,3.46410161513775));
#8385=CARTESIAN_POINT('Ctrl Pts',(-3.,56.6,5.19615242270663));
#8386=CARTESIAN_POINT('Ctrl Pts',(-1.27269028646989E-15,56.6375,6.92820323027551));
#8387=CARTESIAN_POINT('Ctrl Pts',(3.,56.675,5.19615242270663));
#8388=CARTESIAN_POINT('Ctrl Pts',(6.,56.7125,3.46410161513776));
#8389=CARTESIAN_POINT('Ctrl Pts',(6.,56.75,0.));
#8390=CARTESIAN_POINT('Ctrl Pts',(6.,56.7875,-3.46410161513775));
#8391=CARTESIAN_POINT('Ctrl Pts',(3.,56.825,-5.19615242270663));
#8392=CARTESIAN_POINT('Ctrl Pts',(4.24230095489963E-16,56.8625,-6.92820323027551));
#8393=CARTESIAN_POINT('Ctrl Pts',(-3.,56.9,-5.19615242270663));
#8394=CARTESIAN_POINT('Ctrl Pts',(-6.,56.9375,-3.46410161513776));
#8395=CARTESIAN_POINT('Ctrl Pts',(-6.,56.975,-7.34788079488412E-16));
#8396=CARTESIAN_POINT('Ctrl Pts',(-6.,57.0125,3.46410161513775));
#8397=CARTESIAN_POINT('Ctrl Pts',(-3.,57.05,5.19615242270663));
#8398=CARTESIAN_POINT('Ctrl Pts',(-1.27269028646989E-15,57.0875,6.92820323027551));
#8399=CARTESIAN_POINT('Ctrl Pts',(3.,57.125,5.19615242270663));
#8400=CARTESIAN_POINT('Ctrl Pts',(6.,57.1625,3.46410161513776));
#8401=CARTESIAN_POINT('Ctrl Pts',(6.,57.2,0.));
#8402=CARTESIAN_POINT('Ctrl Pts',(6.,57.2375,-3.46410161513775));
#8403=CARTESIAN_POINT('Ctrl Pts',(3.,57.275,-5.19615242270663));
#8404=CARTESIAN_POINT('Ctrl Pts',(4.24230095489963E-16,57.3125,-6.92820323027551));
#8405=CARTESIAN_POINT('Ctrl Pts',(-3.,57.35,-5.19615242270663));
#8406=CARTESIAN_POINT('Ctrl Pts',(-6.,57.3875,-3.46410161513776));
#8407=CARTESIAN_POINT('Ctrl Pts',(-6.,57.425,-7.34788079488412E-16));
#8408=CARTESIAN_POINT('Ctrl Pts',(-6.,57.4625,3.46410161513775));
#8409=CARTESIAN_POINT('Ctrl Pts',(-3.,57.5,5.19615242270663));
#8410=CARTESIAN_POINT('Ctrl Pts',(-1.27269028646989E-15,57.5375,6.92820323027551));
#8411=CARTESIAN_POINT('Ctrl Pts',(3.,57.575,5.19615242270663));
#8412=CARTESIAN_POINT('Ctrl Pts',(6.,57.6125,3.46410161513776));
#8413=CARTESIAN_POINT('Ctrl Pts',(6.,57.65,0.));
#8414=CARTESIAN_POINT('Ctrl Pts',(6.,57.6875,-3.46410161513775));
#8415=CARTESIAN_POINT('Ctrl Pts',(3.,57.725,-5.19615242270663));
#8416=CARTESIAN_POINT('Ctrl Pts',(4.24230095489963E-16,57.7625,-6.92820323027551));
#8417=CARTESIAN_POINT('Ctrl Pts',(-3.,57.8,-5.19615242270663));
#8418=CARTESIAN_POINT('Ctrl Pts',(-6.,57.8375,-3.46410161513776));
#8419=CARTESIAN_POINT('Ctrl Pts',(-6.,57.875,-7.34788079488412E-16));
#8420=CARTESIAN_POINT('Ctrl Pts',(-6.,57.9125,3.46410161513775));
#8421=CARTESIAN_POINT('Ctrl Pts',(-3.,57.95,5.19615242270663));
#8422=CARTESIAN_POINT('Ctrl Pts',(-1.27269028646989E-15,57.9875,6.92820323027551));
#8423=CARTESIAN_POINT('Ctrl Pts',(3.,58.025,5.19615242270663));
#8424=CARTESIAN_POINT('Ctrl Pts',(6.,58.0625,3.46410161513776));
#8425=CARTESIAN_POINT('Ctrl Pts',(6.,58.1,0.));
#8426=CARTESIAN_POINT('Ctrl Pts',(6.,58.1375,-3.46410161513775));
#8427=CARTESIAN_POINT('Ctrl Pts',(3.,58.175,-5.19615242270663));
#8428=CARTESIAN_POINT('Ctrl Pts',(4.24230095489963E-16,58.2125,-6.92820323027551));
#8429=CARTESIAN_POINT('Ctrl Pts',(-3.,58.25,-5.19615242270663));
#8430=CARTESIAN_POINT('Ctrl Pts',(-6.,58.2875,-3.46410161513776));
#8431=CARTESIAN_POINT('Ctrl Pts',(-6.,58.325,-7.34788079488412E-16));
#8432=CARTESIAN_POINT('Ctrl Pts',(-6.,58.3625,3.46410161513775));
#8433=CARTESIAN_POINT('Ctrl Pts',(-3.,58.4,5.19615242270663));
#8434=CARTESIAN_POINT('Ctrl Pts',(-1.27269028646989E-15,58.4375,6.92820323027551));
#8435=CARTESIAN_POINT('Ctrl Pts',(3.,58.475,5.19615242270663));
#8436=CARTESIAN_POINT('Ctrl Pts',(6.,58.5125,3.46410161513776));
#8437=CARTESIAN_POINT('Ctrl Pts',(6.,58.55,0.));
#8438=CARTESIAN_POINT('Ctrl Pts',(6.,58.5875,-3.46410161513775));
#8439=CARTESIAN_POINT('Ctrl Pts',(3.,58.625,-5.19615242270663));
#8440=CARTESIAN_POINT('Ctrl Pts',(4.24230095489963E-16,58.6625,-6.92820323027551));
#8441=CARTESIAN_POINT('Ctrl Pts',(-3.,58.7,-5.19615242270663));
#8442=CARTESIAN_POINT('Ctrl Pts',(-6.,58.7375,-3.46410161513776));
#8443=CARTESIAN_POINT('Ctrl Pts',(-6.,58.775,-7.34788079488412E-16));
#8444=CARTESIAN_POINT('Ctrl Pts',(-6.,58.8125,3.46410161513775));
#8445=CARTESIAN_POINT('Ctrl Pts',(-3.,58.85,5.19615242270663));
#8446=CARTESIAN_POINT('Ctrl Pts',(-1.27269028646989E-15,58.8875,6.92820323027551));
#8447=CARTESIAN_POINT('Ctrl Pts',(3.,58.925,5.19615242270663));
#8448=CARTESIAN_POINT('Ctrl Pts',(6.,58.9625,3.46410161513776));
#8449=CARTESIAN_POINT('Ctrl Pts',(6.,59.,0.));
#8450=CARTESIAN_POINT('Ctrl Pts',(6.,59.0375,-3.46410161513775));
#8451=CARTESIAN_POINT('Ctrl Pts',(3.,59.075,-5.19615242270663));
#8452=CARTESIAN_POINT('Ctrl Pts',(4.24230095489963E-16,59.1125,-6.92820323027551));
#8453=CARTESIAN_POINT('Ctrl Pts',(-3.,59.15,-5.19615242270663));
#8454=CARTESIAN_POINT('Ctrl Pts',(-6.,59.1875,-3.46410161513776));
#8455=CARTESIAN_POINT('Ctrl Pts',(-6.,59.225,-7.34788079488412E-16));
#8456=CARTESIAN_POINT('Ctrl Pts',(-6.,59.2625,3.46410161513775));
#8457=CARTESIAN_POINT('Ctrl Pts',(-3.,59.3,5.19615242270663));
#8458=CARTESIAN_POINT('Ctrl Pts',(-1.27269028646989E-15,59.3375,6.92820323027551));
#8459=CARTESIAN_POINT('Ctrl Pts',(3.,59.375,5.19615242270663));
#8460=CARTESIAN_POINT('Ctrl Pts',(6.,59.4125,3.46410161513776));
#8461=CARTESIAN_POINT('Ctrl Pts',(6.,59.45,0.));
#8462=CARTESIAN_POINT('Ctrl Pts',(6.,59.4875,-3.46410161513775));
#8463=CARTESIAN_POINT('Ctrl Pts',(3.,59.525,-5.19615242270663));
#8464=CARTESIAN_POINT('Ctrl Pts',(4.24230095489963E-16,59.5625,-6.92820323027551));
#8465=CARTESIAN_POINT('Ctrl Pts',(-3.,59.6,-5.19615242270663));
#8466=CARTESIAN_POINT('Ctrl Pts',(-6.,59.6375,-3.46410161513776));
#8467=CARTESIAN_POINT('Ctrl Pts',(-6.,59.675,-7.34788079488412E-16));
#8468=CARTESIAN_POINT('Ctrl Pts',(-6.,59.7125,3.46410161513775));
#8469=CARTESIAN_POINT('Ctrl Pts',(-3.,59.75,5.19615242270663));
#8470=CARTESIAN_POINT('Ctrl Pts',(-1.27269028646989E-15,59.7875,6.92820323027551));
#8471=CARTESIAN_POINT('Ctrl Pts',(3.,59.825,5.19615242270663));
#8472=CARTESIAN_POINT('Ctrl Pts',(6.,59.8625,3.46410161513776));
#8473=CARTESIAN_POINT('Ctrl Pts',(6.,59.9,0.));
#8474=CARTESIAN_POINT('Ctrl Pts',(6.,59.9375,-3.46410161513775));
#8475=CARTESIAN_POINT('Ctrl Pts',(3.,59.975,-5.19615242270663));
#8476=CARTESIAN_POINT('Ctrl Pts',(4.24230095489963E-16,60.0125,-6.92820323027551));
#8477=CARTESIAN_POINT('Ctrl Pts',(-3.,60.05,-5.19615242270663));
#8478=CARTESIAN_POINT('Ctrl Pts',(-6.,60.0875,-3.46410161513776));
#8479=CARTESIAN_POINT('Ctrl Pts',(-6.,60.125,-7.34788079488412E-16));
#8480=CARTESIAN_POINT('Ctrl Pts',(-6.,60.1625,3.46410161513775));
#8481=CARTESIAN_POINT('Ctrl Pts',(-3.,60.2,5.19615242270663));
#8482=CARTESIAN_POINT('Ctrl Pts',(-1.27269028646989E-15,60.2375,6.92820323027551));
#8483=CARTESIAN_POINT('Ctrl Pts',(3.,60.275,5.19615242270663));
#8484=CARTESIAN_POINT('Ctrl Pts',(6.,60.3125,3.46410161513776));
#8485=CARTESIAN_POINT('Ctrl Pts',(6.,60.35,0.));
#8486=CARTESIAN_POINT('Ctrl Pts',(6.,60.3875,-3.46410161513775));
#8487=CARTESIAN_POINT('Ctrl Pts',(3.,60.425,-5.19615242270663));
#8488=CARTESIAN_POINT('Ctrl Pts',(4.24230095489963E-16,60.4625,-6.92820323027551));
#8489=CARTESIAN_POINT('Ctrl Pts',(-3.,60.5,-5.19615242270663));
#8490=CARTESIAN_POINT('Ctrl Pts',(-6.,60.5375,-3.46410161513776));
#8491=CARTESIAN_POINT('Ctrl Pts',(-6.,60.575,-7.34788079488412E-16));
#8492=CARTESIAN_POINT('Ctrl Pts',(-6.,60.6125,3.46410161513775));
#8493=CARTESIAN_POINT('Ctrl Pts',(-3.,60.65,5.19615242270663));
#8494=CARTESIAN_POINT('Ctrl Pts',(-1.27269028646989E-15,60.6875,6.92820323027551));
#8495=CARTESIAN_POINT('Ctrl Pts',(3.,60.725,5.19615242270663));
#8496=CARTESIAN_POINT('Ctrl Pts',(6.,60.7625,3.46410161513776));
#8497=CARTESIAN_POINT('Ctrl Pts',(6.,60.8,0.));
#8498=CARTESIAN_POINT('Ctrl Pts',(6.,60.8375,-3.46410161513775));
#8499=CARTESIAN_POINT('Ctrl Pts',(3.,60.875,-5.19615242270663));
#8500=CARTESIAN_POINT('Ctrl Pts',(4.24230095489963E-16,60.9125,-6.92820323027551));
#8501=CARTESIAN_POINT('Ctrl Pts',(-3.,60.95,-5.19615242270663));
#8502=CARTESIAN_POINT('Ctrl Pts',(-6.,60.9875,-3.46410161513776));
#8503=CARTESIAN_POINT('Ctrl Pts',(-6.,61.025,-7.34788079488412E-16));
#8504=CARTESIAN_POINT('Ctrl Pts',(-6.,61.0625,3.46410161513775));
#8505=CARTESIAN_POINT('Ctrl Pts',(-3.,61.1,5.19615242270663));
#8506=CARTESIAN_POINT('Ctrl Pts',(-1.27269028646989E-15,61.1375,6.92820323027551));
#8507=CARTESIAN_POINT('Ctrl Pts',(3.,61.175,5.19615242270663));
#8508=CARTESIAN_POINT('Ctrl Pts',(6.,61.2125,3.46410161513776));
#8509=CARTESIAN_POINT('Ctrl Pts',(6.,61.25,0.));
#8510=CARTESIAN_POINT('Ctrl Pts',(6.,61.2875,-3.46410161513775));
#8511=CARTESIAN_POINT('Ctrl Pts',(3.,61.325,-5.19615242270663));
#8512=CARTESIAN_POINT('Ctrl Pts',(4.24230095489963E-16,61.3625,-6.92820323027551));
#8513=CARTESIAN_POINT('Ctrl Pts',(-3.,61.4,-5.19615242270663));
#8514=CARTESIAN_POINT('Ctrl Pts',(-6.,61.4375,-3.46410161513776));
#8515=CARTESIAN_POINT('Ctrl Pts',(-6.,61.475,-7.34788079488412E-16));
#8516=CARTESIAN_POINT('Ctrl Pts',(-6.,61.5125,3.46410161513775));
#8517=CARTESIAN_POINT('Ctrl Pts',(-3.,61.55,5.19615242270663));
#8518=CARTESIAN_POINT('Ctrl Pts',(-1.27269028646989E-15,61.5875,6.92820323027551));
#8519=CARTESIAN_POINT('Ctrl Pts',(3.,61.625,5.19615242270663));
#8520=CARTESIAN_POINT('Ctrl Pts',(6.,61.6625,3.46410161513776));
#8521=CARTESIAN_POINT('Ctrl Pts',(6.,61.7,0.));
#8522=CARTESIAN_POINT('Ctrl Pts',(6.,61.7375,-3.46410161513775));
#8523=CARTESIAN_POINT('Ctrl Pts',(3.,61.775,-5.19615242270663));
#8524=CARTESIAN_POINT('Ctrl Pts',(4.24230095489963E-16,61.8125,-6.92820323027551));
#8525=CARTESIAN_POINT('Ctrl Pts',(-3.,61.85,-5.19615242270663));
#8526=CARTESIAN_POINT('Ctrl Pts',(-6.,61.8875,-3.46410161513776));
#8527=CARTESIAN_POINT('Ctrl Pts',(-6.,61.925,-7.34788079488412E-16));
#8528=CARTESIAN_POINT('Ctrl Pts',(-6.,61.9625,3.46410161513775));
#8529=CARTESIAN_POINT('Ctrl Pts',(-3.,62.,5.19615242270663));
#8530=CARTESIAN_POINT('Ctrl Pts',(5.75643035625,50.1406249993855,0.));
#8531=CARTESIAN_POINT('Ctrl Pts',(5.75643035625,50.1781249993855,-3.32347661575227));
#8532=CARTESIAN_POINT('Ctrl Pts',(2.878215178125,50.2156249993855,-4.9852149236284));
#8533=CARTESIAN_POINT('Ctrl Pts',(4.0700849995221E-16,50.2531249993855,
-6.64695323150454));
#8534=CARTESIAN_POINT('Ctrl Pts',(-2.878215178125,50.2906249993855,-4.9852149236284));
#8535=CARTESIAN_POINT('Ctrl Pts',(-5.75643035625,50.3281249993855,-3.32347661575227));
#8536=CARTESIAN_POINT('Ctrl Pts',(-5.75643035625,50.3656249993855,-7.04959401029622E-16));
#8537=CARTESIAN_POINT('Origin',(-2.22044604925031E-15,50.1968749993855,
-2.77555756156289E-16));
#8538=CARTESIAN_POINT('Ctrl Pts',(5.75643035625,50.2531249993855,0.));
#8539=CARTESIAN_POINT('Ctrl Pts',(5.75643035625,50.2906249993855,-3.32347661575227));
#8540=CARTESIAN_POINT('Ctrl Pts',(2.878215178125,50.3281249993855,-4.9852149236284));
#8541=CARTESIAN_POINT('Ctrl Pts',(4.0700849995221E-16,50.3656249993855,
-6.64695323150454));
#8542=CARTESIAN_POINT('Ctrl Pts',(-2.878215178125,50.4031249993855,-4.9852149236284));
#8543=CARTESIAN_POINT('Ctrl Pts',(-5.75643035625,50.4406249993855,-3.32347661575227));
#8544=CARTESIAN_POINT('Ctrl Pts',(-5.75643035625,50.4781249993855,-7.04959401029622E-16));
#8545=CARTESIAN_POINT('Ctrl Pts',(6.,50.393749998771,0.));
#8546=CARTESIAN_POINT('Ctrl Pts',(6.,50.431249998771,-3.46410161513775));
#8547=CARTESIAN_POINT('Ctrl Pts',(3.,50.468749998771,-5.19615242270663));
#8548=CARTESIAN_POINT('Ctrl Pts',(4.24230095489963E-16,50.506249998771,
-6.92820323027551));
#8549=CARTESIAN_POINT('Ctrl Pts',(-3.,50.543749998771,-5.19615242270663));
#8550=CARTESIAN_POINT('Ctrl Pts',(-6.,50.581249998771,-3.46410161513776));
#8551=CARTESIAN_POINT('Ctrl Pts',(-6.,50.618749998771,-7.34788079488412E-16));
#8552=CARTESIAN_POINT('Ctrl Pts',(-6.,50.656249998771,3.46410161513775));
#8553=CARTESIAN_POINT('Ctrl Pts',(-3.,50.693749998771,5.19615242270663));
#8554=CARTESIAN_POINT('Ctrl Pts',(-1.27269028646989E-15,50.731249998771,
6.92820323027551));
#8555=CARTESIAN_POINT('Ctrl Pts',(3.,50.768749998771,5.19615242270663));
#8556=CARTESIAN_POINT('Ctrl Pts',(6.,50.806249998771,3.46410161513776));
#8557=CARTESIAN_POINT('Ctrl Pts',(6.,50.843749998771,0.));
#8558=CARTESIAN_POINT('Ctrl Pts',(6.,50.881249998771,-3.46410161513775));
#8559=CARTESIAN_POINT('Ctrl Pts',(3.,50.918749998771,-5.19615242270663));
#8560=CARTESIAN_POINT('Ctrl Pts',(4.24230095489963E-16,50.956249998771,
-6.92820323027551));
#8561=CARTESIAN_POINT('Ctrl Pts',(-3.,50.993749998771,-5.19615242270663));
#8562=CARTESIAN_POINT('Ctrl Pts',(-6.,51.031249998771,-3.46410161513776));
#8563=CARTESIAN_POINT('Ctrl Pts',(-6.,51.068749998771,-7.34788079488412E-16));
#8564=CARTESIAN_POINT('Ctrl Pts',(-6.,51.106249998771,3.46410161513775));
#8565=CARTESIAN_POINT('Ctrl Pts',(-3.,51.143749998771,5.19615242270663));
#8566=CARTESIAN_POINT('Ctrl Pts',(-1.27269028646989E-15,51.181249998771,
6.92820323027551));
#8567=CARTESIAN_POINT('Ctrl Pts',(3.,51.218749998771,5.19615242270663));
#8568=CARTESIAN_POINT('Ctrl Pts',(6.,51.256249998771,3.46410161513776));
#8569=CARTESIAN_POINT('Ctrl Pts',(6.,51.293749998771,0.));
#8570=CARTESIAN_POINT('Ctrl Pts',(6.,51.331249998771,-3.46410161513775));
#8571=CARTESIAN_POINT('Ctrl Pts',(3.,51.368749998771,-5.19615242270663));
#8572=CARTESIAN_POINT('Ctrl Pts',(4.24230095489963E-16,51.406249998771,
-6.92820323027551));
#8573=CARTESIAN_POINT('Ctrl Pts',(-3.,51.443749998771,-5.19615242270663));
#8574=CARTESIAN_POINT('Ctrl Pts',(-6.,51.481249998771,-3.46410161513776));
#8575=CARTESIAN_POINT('Ctrl Pts',(-6.,51.518749998771,-7.34788079488412E-16));
#8576=CARTESIAN_POINT('Ctrl Pts',(-6.,51.556249998771,3.46410161513775));
#8577=CARTESIAN_POINT('Ctrl Pts',(-3.,51.593749998771,5.19615242270663));
#8578=CARTESIAN_POINT('Ctrl Pts',(-1.27269028646989E-15,51.631249998771,
6.92820323027551));
#8579=CARTESIAN_POINT('Ctrl Pts',(3.,51.668749998771,5.19615242270663));
#8580=CARTESIAN_POINT('Ctrl Pts',(6.,51.706249998771,3.46410161513776));
#8581=CARTESIAN_POINT('Ctrl Pts',(6.,51.743749998771,0.));
#8582=CARTESIAN_POINT('Ctrl Pts',(6.,51.781249998771,-3.46410161513775));
#8583=CARTESIAN_POINT('Ctrl Pts',(3.,51.818749998771,-5.19615242270663));
#8584=CARTESIAN_POINT('Ctrl Pts',(4.24230095489963E-16,51.856249998771,
-6.92820323027551));
#8585=CARTESIAN_POINT('Ctrl Pts',(-3.,51.893749998771,-5.19615242270663));
#8586=CARTESIAN_POINT('Ctrl Pts',(-6.,51.931249998771,-3.46410161513776));
#8587=CARTESIAN_POINT('Ctrl Pts',(-6.,51.968749998771,-7.34788079488412E-16));
#8588=CARTESIAN_POINT('Ctrl Pts',(-6.,52.006249998771,3.46410161513775));
#8589=CARTESIAN_POINT('Ctrl Pts',(-3.,52.043749998771,5.19615242270663));
#8590=CARTESIAN_POINT('Ctrl Pts',(-1.27269028646989E-15,52.081249998771,
6.92820323027551));
#8591=CARTESIAN_POINT('Ctrl Pts',(3.,52.118749998771,5.19615242270663));
#8592=CARTESIAN_POINT('Ctrl Pts',(6.,52.156249998771,3.46410161513776));
#8593=CARTESIAN_POINT('Ctrl Pts',(6.,52.193749998771,0.));
#8594=CARTESIAN_POINT('Ctrl Pts',(6.,52.231249998771,-3.46410161513775));
#8595=CARTESIAN_POINT('Ctrl Pts',(3.,52.268749998771,-5.19615242270663));
#8596=CARTESIAN_POINT('Ctrl Pts',(4.24230095489963E-16,52.306249998771,
-6.92820323027551));
#8597=CARTESIAN_POINT('Ctrl Pts',(-3.,52.343749998771,-5.19615242270663));
#8598=CARTESIAN_POINT('Ctrl Pts',(-6.,52.381249998771,-3.46410161513776));
#8599=CARTESIAN_POINT('Ctrl Pts',(-6.,52.418749998771,-7.34788079488412E-16));
#8600=CARTESIAN_POINT('Ctrl Pts',(-6.,52.456249998771,3.46410161513775));
#8601=CARTESIAN_POINT('Ctrl Pts',(-3.,52.493749998771,5.19615242270663));
#8602=CARTESIAN_POINT('Ctrl Pts',(-1.27269028646989E-15,52.531249998771,
6.92820323027551));
#8603=CARTESIAN_POINT('Ctrl Pts',(3.,52.568749998771,5.19615242270663));
#8604=CARTESIAN_POINT('Ctrl Pts',(6.,52.606249998771,3.46410161513776));
#8605=CARTESIAN_POINT('Ctrl Pts',(6.,52.643749998771,0.));
#8606=CARTESIAN_POINT('Ctrl Pts',(6.,52.681249998771,-3.46410161513775));
#8607=CARTESIAN_POINT('Ctrl Pts',(3.,52.718749998771,-5.19615242270663));
#8608=CARTESIAN_POINT('Ctrl Pts',(4.24230095489963E-16,52.756249998771,
-6.92820323027551));
#8609=CARTESIAN_POINT('Ctrl Pts',(-3.,52.793749998771,-5.19615242270663));
#8610=CARTESIAN_POINT('Ctrl Pts',(-6.,52.831249998771,-3.46410161513776));
#8611=CARTESIAN_POINT('Ctrl Pts',(-6.,52.868749998771,-7.34788079488412E-16));
#8612=CARTESIAN_POINT('Ctrl Pts',(-6.,52.906249998771,3.46410161513775));
#8613=CARTESIAN_POINT('Ctrl Pts',(-3.,52.943749998771,5.19615242270663));
#8614=CARTESIAN_POINT('Ctrl Pts',(-1.27269028646989E-15,52.981249998771,
6.92820323027551));
#8615=CARTESIAN_POINT('Ctrl Pts',(3.,53.018749998771,5.19615242270663));
#8616=CARTESIAN_POINT('Ctrl Pts',(6.,53.056249998771,3.46410161513776));
#8617=CARTESIAN_POINT('Ctrl Pts',(6.,53.093749998771,0.));
#8618=CARTESIAN_POINT('Ctrl Pts',(6.,53.131249998771,-3.46410161513775));
#8619=CARTESIAN_POINT('Ctrl Pts',(3.,53.168749998771,-5.19615242270663));
#8620=CARTESIAN_POINT('Ctrl Pts',(4.24230095489963E-16,53.206249998771,
-6.92820323027551));
#8621=CARTESIAN_POINT('Ctrl Pts',(-3.,53.243749998771,-5.19615242270663));
#8622=CARTESIAN_POINT('Ctrl Pts',(-6.,53.281249998771,-3.46410161513776));
#8623=CARTESIAN_POINT('Ctrl Pts',(-6.,53.318749998771,-7.34788079488412E-16));
#8624=CARTESIAN_POINT('Ctrl Pts',(-6.,53.356249998771,3.46410161513775));
#8625=CARTESIAN_POINT('Ctrl Pts',(-3.,53.393749998771,5.19615242270663));
#8626=CARTESIAN_POINT('Ctrl Pts',(-1.27269028646989E-15,53.431249998771,
6.92820323027551));
#8627=CARTESIAN_POINT('Ctrl Pts',(3.,53.468749998771,5.19615242270663));
#8628=CARTESIAN_POINT('Ctrl Pts',(6.,53.506249998771,3.46410161513776));
#8629=CARTESIAN_POINT('Ctrl Pts',(6.,53.543749998771,0.));
#8630=CARTESIAN_POINT('Ctrl Pts',(6.,53.581249998771,-3.46410161513775));
#8631=CARTESIAN_POINT('Ctrl Pts',(3.,53.618749998771,-5.19615242270663));
#8632=CARTESIAN_POINT('Ctrl Pts',(4.24230095489963E-16,53.656249998771,
-6.92820323027551));
#8633=CARTESIAN_POINT('Ctrl Pts',(-3.,53.693749998771,-5.19615242270663));
#8634=CARTESIAN_POINT('Ctrl Pts',(-6.,53.731249998771,-3.46410161513776));
#8635=CARTESIAN_POINT('Ctrl Pts',(-6.,53.768749998771,-7.34788079488412E-16));
#8636=CARTESIAN_POINT('Ctrl Pts',(-6.,53.806249998771,3.46410161513775));
#8637=CARTESIAN_POINT('Ctrl Pts',(-3.,53.843749998771,5.19615242270663));
#8638=CARTESIAN_POINT('Ctrl Pts',(-1.27269028646989E-15,53.881249998771,
6.92820323027551));
#8639=CARTESIAN_POINT('Ctrl Pts',(3.,53.918749998771,5.19615242270663));
#8640=CARTESIAN_POINT('Ctrl Pts',(6.,53.956249998771,3.46410161513776));
#8641=CARTESIAN_POINT('Ctrl Pts',(6.,53.993749998771,0.));
#8642=CARTESIAN_POINT('Ctrl Pts',(6.,54.031249998771,-3.46410161513775));
#8643=CARTESIAN_POINT('Ctrl Pts',(3.,54.068749998771,-5.19615242270663));
#8644=CARTESIAN_POINT('Ctrl Pts',(4.24230095489963E-16,54.106249998771,
-6.92820323027551));
#8645=CARTESIAN_POINT('Ctrl Pts',(-3.,54.143749998771,-5.19615242270663));
#8646=CARTESIAN_POINT('Ctrl Pts',(-6.,54.181249998771,-3.46410161513776));
#8647=CARTESIAN_POINT('Ctrl Pts',(-6.,54.218749998771,-7.34788079488412E-16));
#8648=CARTESIAN_POINT('Ctrl Pts',(-6.,54.256249998771,3.46410161513775));
#8649=CARTESIAN_POINT('Ctrl Pts',(-3.,54.293749998771,5.19615242270663));
#8650=CARTESIAN_POINT('Ctrl Pts',(-1.27269028646989E-15,54.331249998771,
6.92820323027551));
#8651=CARTESIAN_POINT('Ctrl Pts',(3.,54.368749998771,5.19615242270663));
#8652=CARTESIAN_POINT('Ctrl Pts',(6.,54.406249998771,3.46410161513776));
#8653=CARTESIAN_POINT('Ctrl Pts',(6.,54.443749998771,0.));
#8654=CARTESIAN_POINT('Ctrl Pts',(6.,54.481249998771,-3.46410161513775));
#8655=CARTESIAN_POINT('Ctrl Pts',(3.,54.518749998771,-5.19615242270663));
#8656=CARTESIAN_POINT('Ctrl Pts',(4.24230095489963E-16,54.556249998771,
-6.92820323027551));
#8657=CARTESIAN_POINT('Ctrl Pts',(-3.,54.593749998771,-5.19615242270663));
#8658=CARTESIAN_POINT('Ctrl Pts',(-6.,54.631249998771,-3.46410161513776));
#8659=CARTESIAN_POINT('Ctrl Pts',(-6.,54.668749998771,-7.34788079488412E-16));
#8660=CARTESIAN_POINT('Ctrl Pts',(-6.,54.706249998771,3.46410161513775));
#8661=CARTESIAN_POINT('Ctrl Pts',(-3.,54.743749998771,5.19615242270663));
#8662=CARTESIAN_POINT('Ctrl Pts',(-1.27269028646989E-15,54.781249998771,
6.92820323027551));
#8663=CARTESIAN_POINT('Ctrl Pts',(3.,54.818749998771,5.19615242270663));
#8664=CARTESIAN_POINT('Ctrl Pts',(6.,54.856249998771,3.46410161513776));
#8665=CARTESIAN_POINT('Ctrl Pts',(6.,54.893749998771,0.));
#8666=CARTESIAN_POINT('Ctrl Pts',(6.,54.931249998771,-3.46410161513775));
#8667=CARTESIAN_POINT('Ctrl Pts',(3.,54.968749998771,-5.19615242270663));
#8668=CARTESIAN_POINT('Ctrl Pts',(4.24230095489963E-16,55.006249998771,
-6.92820323027551));
#8669=CARTESIAN_POINT('Ctrl Pts',(-3.,55.043749998771,-5.19615242270663));
#8670=CARTESIAN_POINT('Ctrl Pts',(-6.,55.081249998771,-3.46410161513776));
#8671=CARTESIAN_POINT('Ctrl Pts',(-6.,55.118749998771,-7.34788079488412E-16));
#8672=CARTESIAN_POINT('Ctrl Pts',(-6.,55.156249998771,3.46410161513775));
#8673=CARTESIAN_POINT('Ctrl Pts',(-3.,55.193749998771,5.19615242270663));
#8674=CARTESIAN_POINT('Ctrl Pts',(-1.27269028646989E-15,55.231249998771,
6.92820323027551));
#8675=CARTESIAN_POINT('Ctrl Pts',(3.,55.268749998771,5.19615242270663));
#8676=CARTESIAN_POINT('Ctrl Pts',(6.,55.306249998771,3.46410161513776));
#8677=CARTESIAN_POINT('Ctrl Pts',(6.,55.343749998771,0.));
#8678=CARTESIAN_POINT('Ctrl Pts',(6.,55.381249998771,-3.46410161513775));
#8679=CARTESIAN_POINT('Ctrl Pts',(3.,55.418749998771,-5.19615242270663));
#8680=CARTESIAN_POINT('Ctrl Pts',(4.24230095489963E-16,55.456249998771,
-6.92820323027551));
#8681=CARTESIAN_POINT('Ctrl Pts',(-3.,55.493749998771,-5.19615242270663));
#8682=CARTESIAN_POINT('Ctrl Pts',(-6.,55.531249998771,-3.46410161513776));
#8683=CARTESIAN_POINT('Ctrl Pts',(-6.,55.568749998771,-7.34788079488412E-16));
#8684=CARTESIAN_POINT('Ctrl Pts',(-6.,55.606249998771,3.46410161513775));
#8685=CARTESIAN_POINT('Ctrl Pts',(-3.,55.643749998771,5.19615242270663));
#8686=CARTESIAN_POINT('Ctrl Pts',(-1.27269028646989E-15,55.681249998771,
6.92820323027551));
#8687=CARTESIAN_POINT('Ctrl Pts',(3.,55.718749998771,5.19615242270663));
#8688=CARTESIAN_POINT('Ctrl Pts',(6.,55.756249998771,3.46410161513776));
#8689=CARTESIAN_POINT('Ctrl Pts',(6.,55.793749998771,0.));
#8690=CARTESIAN_POINT('Ctrl Pts',(6.,55.831249998771,-3.46410161513775));
#8691=CARTESIAN_POINT('Ctrl Pts',(3.,55.868749998771,-5.19615242270663));
#8692=CARTESIAN_POINT('Ctrl Pts',(4.24230095489963E-16,55.906249998771,
-6.92820323027551));
#8693=CARTESIAN_POINT('Ctrl Pts',(-3.,55.943749998771,-5.19615242270663));
#8694=CARTESIAN_POINT('Ctrl Pts',(-6.,55.981249998771,-3.46410161513776));
#8695=CARTESIAN_POINT('Ctrl Pts',(-6.,56.018749998771,-7.34788079488412E-16));
#8696=CARTESIAN_POINT('Ctrl Pts',(-6.,56.056249998771,3.46410161513775));
#8697=CARTESIAN_POINT('Ctrl Pts',(-3.,56.093749998771,5.19615242270663));
#8698=CARTESIAN_POINT('Ctrl Pts',(-1.27269028646989E-15,56.1312499987709,
6.92820323027551));
#8699=CARTESIAN_POINT('Ctrl Pts',(3.,56.168749998771,5.19615242270663));
#8700=CARTESIAN_POINT('Ctrl Pts',(6.,56.206249998771,3.46410161513776));
#8701=CARTESIAN_POINT('Ctrl Pts',(6.,56.243749998771,0.));
#8702=CARTESIAN_POINT('Ctrl Pts',(6.,56.281249998771,-3.46410161513775));
#8703=CARTESIAN_POINT('Ctrl Pts',(3.,56.318749998771,-5.19615242270663));
#8704=CARTESIAN_POINT('Ctrl Pts',(4.24230095489963E-16,56.3562499987709,
-6.92820323027551));
#8705=CARTESIAN_POINT('Ctrl Pts',(-3.,56.393749998771,-5.19615242270663));
#8706=CARTESIAN_POINT('Ctrl Pts',(-6.,56.431249998771,-3.46410161513776));
#8707=CARTESIAN_POINT('Ctrl Pts',(-6.,56.468749998771,-7.34788079488412E-16));
#8708=CARTESIAN_POINT('Ctrl Pts',(-6.,56.506249998771,3.46410161513775));
#8709=CARTESIAN_POINT('Ctrl Pts',(-3.,56.543749998771,5.19615242270663));
#8710=CARTESIAN_POINT('Ctrl Pts',(-1.27269028646989E-15,56.581249998771,
6.92820323027551));
#8711=CARTESIAN_POINT('Ctrl Pts',(3.,56.618749998771,5.19615242270663));
#8712=CARTESIAN_POINT('Ctrl Pts',(6.,56.656249998771,3.46410161513776));
#8713=CARTESIAN_POINT('Ctrl Pts',(6.,56.693749998771,0.));
#8714=CARTESIAN_POINT('Ctrl Pts',(6.,56.731249998771,-3.46410161513775));
#8715=CARTESIAN_POINT('Ctrl Pts',(3.,56.768749998771,-5.19615242270663));
#8716=CARTESIAN_POINT('Ctrl Pts',(4.24230095489963E-16,56.806249998771,
-6.92820323027551));
#8717=CARTESIAN_POINT('Ctrl Pts',(-3.,56.843749998771,-5.19615242270663));
#8718=CARTESIAN_POINT('Ctrl Pts',(-6.,56.881249998771,-3.46410161513776));
#8719=CARTESIAN_POINT('Ctrl Pts',(-6.,56.918749998771,-7.34788079488412E-16));
#8720=CARTESIAN_POINT('Ctrl Pts',(-6.,56.956249998771,3.46410161513775));
#8721=CARTESIAN_POINT('Ctrl Pts',(-3.,56.993749998771,5.19615242270663));
#8722=CARTESIAN_POINT('Ctrl Pts',(-1.27269028646989E-15,57.031249998771,
6.92820323027551));
#8723=CARTESIAN_POINT('Ctrl Pts',(3.,57.068749998771,5.19615242270663));
#8724=CARTESIAN_POINT('Ctrl Pts',(6.,57.106249998771,3.46410161513776));
#8725=CARTESIAN_POINT('Ctrl Pts',(6.,57.143749998771,0.));
#8726=CARTESIAN_POINT('Ctrl Pts',(6.,57.181249998771,-3.46410161513775));
#8727=CARTESIAN_POINT('Ctrl Pts',(3.,57.218749998771,-5.19615242270663));
#8728=CARTESIAN_POINT('Ctrl Pts',(4.24230095489963E-16,57.256249998771,
-6.92820323027551));
#8729=CARTESIAN_POINT('Ctrl Pts',(-3.,57.293749998771,-5.19615242270663));
#8730=CARTESIAN_POINT('Ctrl Pts',(-6.,57.331249998771,-3.46410161513776));
#8731=CARTESIAN_POINT('Ctrl Pts',(-6.,57.368749998771,-7.34788079488412E-16));
#8732=CARTESIAN_POINT('Ctrl Pts',(-6.,57.406249998771,3.46410161513775));
#8733=CARTESIAN_POINT('Ctrl Pts',(-3.,57.443749998771,5.19615242270663));
#8734=CARTESIAN_POINT('Ctrl Pts',(-1.27269028646989E-15,57.481249998771,
6.92820323027551));
#8735=CARTESIAN_POINT('Ctrl Pts',(3.,57.518749998771,5.19615242270663));
#8736=CARTESIAN_POINT('Ctrl Pts',(6.,57.556249998771,3.46410161513776));
#8737=CARTESIAN_POINT('Ctrl Pts',(6.,57.593749998771,0.));
#8738=CARTESIAN_POINT('Ctrl Pts',(6.,57.631249998771,-3.46410161513775));
#8739=CARTESIAN_POINT('Ctrl Pts',(3.,57.668749998771,-5.19615242270663));
#8740=CARTESIAN_POINT('Ctrl Pts',(4.24230095489963E-16,57.706249998771,
-6.92820323027551));
#8741=CARTESIAN_POINT('Ctrl Pts',(-3.,57.743749998771,-5.19615242270663));
#8742=CARTESIAN_POINT('Ctrl Pts',(-6.,57.781249998771,-3.46410161513776));
#8743=CARTESIAN_POINT('Ctrl Pts',(-6.,57.818749998771,-7.34788079488412E-16));
#8744=CARTESIAN_POINT('Ctrl Pts',(-6.,57.8562499987709,3.46410161513775));
#8745=CARTESIAN_POINT('Ctrl Pts',(-3.,57.893749998771,5.19615242270663));
#8746=CARTESIAN_POINT('Ctrl Pts',(-1.27269028646989E-15,57.931249998771,
6.92820323027551));
#8747=CARTESIAN_POINT('Ctrl Pts',(3.,57.968749998771,5.19615242270663));
#8748=CARTESIAN_POINT('Ctrl Pts',(6.,58.0062499987709,3.46410161513776));
#8749=CARTESIAN_POINT('Ctrl Pts',(6.,58.043749998771,0.));
#8750=CARTESIAN_POINT('Ctrl Pts',(6.,58.081249998771,-3.46410161513775));
#8751=CARTESIAN_POINT('Ctrl Pts',(3.,58.118749998771,-5.19615242270663));
#8752=CARTESIAN_POINT('Ctrl Pts',(4.24230095489963E-16,58.156249998771,
-6.92820323027551));
#8753=CARTESIAN_POINT('Ctrl Pts',(-3.,58.193749998771,-5.19615242270663));
#8754=CARTESIAN_POINT('Ctrl Pts',(-6.,58.231249998771,-3.46410161513776));
#8755=CARTESIAN_POINT('Ctrl Pts',(-6.,58.268749998771,-7.34788079488412E-16));
#8756=CARTESIAN_POINT('Ctrl Pts',(-6.,58.306249998771,3.46410161513775));
#8757=CARTESIAN_POINT('Ctrl Pts',(-3.,58.343749998771,5.19615242270663));
#8758=CARTESIAN_POINT('Ctrl Pts',(-1.27269028646989E-15,58.381249998771,
6.92820323027551));
#8759=CARTESIAN_POINT('Ctrl Pts',(3.,58.418749998771,5.19615242270663));
#8760=CARTESIAN_POINT('Ctrl Pts',(6.,58.456249998771,3.46410161513776));
#8761=CARTESIAN_POINT('Ctrl Pts',(6.,58.493749998771,0.));
#8762=CARTESIAN_POINT('Ctrl Pts',(6.,58.531249998771,-3.46410161513775));
#8763=CARTESIAN_POINT('Ctrl Pts',(3.,58.568749998771,-5.19615242270663));
#8764=CARTESIAN_POINT('Ctrl Pts',(4.24230095489963E-16,58.606249998771,
-6.92820323027551));
#8765=CARTESIAN_POINT('Ctrl Pts',(-3.,58.643749998771,-5.19615242270663));
#8766=CARTESIAN_POINT('Ctrl Pts',(-6.,58.681249998771,-3.46410161513776));
#8767=CARTESIAN_POINT('Ctrl Pts',(-6.,58.718749998771,-7.34788079488412E-16));
#8768=CARTESIAN_POINT('Ctrl Pts',(-6.,58.756249998771,3.46410161513775));
#8769=CARTESIAN_POINT('Ctrl Pts',(-3.,58.793749998771,5.19615242270663));
#8770=CARTESIAN_POINT('Ctrl Pts',(-1.27269028646989E-15,58.831249998771,
6.92820323027551));
#8771=CARTESIAN_POINT('Ctrl Pts',(3.,58.868749998771,5.19615242270663));
#8772=CARTESIAN_POINT('Ctrl Pts',(6.,58.906249998771,3.46410161513776));
#8773=CARTESIAN_POINT('Ctrl Pts',(6.,58.943749998771,0.));
#8774=CARTESIAN_POINT('Ctrl Pts',(6.,58.981249998771,-3.46410161513775));
#8775=CARTESIAN_POINT('Ctrl Pts',(3.,59.018749998771,-5.19615242270663));
#8776=CARTESIAN_POINT('Ctrl Pts',(4.24230095489963E-16,59.056249998771,
-6.92820323027551));
#8777=CARTESIAN_POINT('Ctrl Pts',(-3.,59.093749998771,-5.19615242270663));
#8778=CARTESIAN_POINT('Ctrl Pts',(-6.,59.1312499987709,-3.46410161513776));
#8779=CARTESIAN_POINT('Ctrl Pts',(-6.,59.168749998771,-7.34788079488412E-16));
#8780=CARTESIAN_POINT('Ctrl Pts',(-6.,59.206249998771,3.46410161513775));
#8781=CARTESIAN_POINT('Ctrl Pts',(-3.,59.243749998771,5.19615242270663));
#8782=CARTESIAN_POINT('Ctrl Pts',(-1.27269028646989E-15,59.281249998771,
6.92820323027551));
#8783=CARTESIAN_POINT('Ctrl Pts',(3.,59.318749998771,5.19615242270663));
#8784=CARTESIAN_POINT('Ctrl Pts',(6.,59.356249998771,3.46410161513776));
#8785=CARTESIAN_POINT('Ctrl Pts',(6.,59.393749998771,0.));
#8786=CARTESIAN_POINT('Ctrl Pts',(6.,59.431249998771,-3.46410161513775));
#8787=CARTESIAN_POINT('Ctrl Pts',(3.,59.468749998771,-5.19615242270663));
#8788=CARTESIAN_POINT('Ctrl Pts',(4.24230095489963E-16,59.506249998771,
-6.92820323027551));
#8789=CARTESIAN_POINT('Ctrl Pts',(-3.,59.543749998771,-5.19615242270663));
#8790=CARTESIAN_POINT('Ctrl Pts',(-6.,59.581249998771,-3.46410161513776));
#8791=CARTESIAN_POINT('Ctrl Pts',(-6.,59.618749998771,-7.34788079488412E-16));
#8792=CARTESIAN_POINT('Ctrl Pts',(-6.,59.656249998771,3.46410161513775));
#8793=CARTESIAN_POINT('Ctrl Pts',(-3.,59.693749998771,5.19615242270663));
#8794=CARTESIAN_POINT('Ctrl Pts',(-1.27269028646989E-15,59.731249998771,
6.92820323027551));
#8795=CARTESIAN_POINT('Ctrl Pts',(3.,59.768749998771,5.19615242270663));
#8796=CARTESIAN_POINT('Ctrl Pts',(6.,59.806249998771,3.46410161513776));
#8797=CARTESIAN_POINT('Ctrl Pts',(6.,59.843749998771,0.));
#8798=CARTESIAN_POINT('Ctrl Pts',(6.,59.881249998771,-3.46410161513775));
#8799=CARTESIAN_POINT('Ctrl Pts',(3.,59.918749998771,-5.19615242270663));
#8800=CARTESIAN_POINT('Ctrl Pts',(4.24230095489963E-16,59.956249998771,
-6.92820323027551));
#8801=CARTESIAN_POINT('Ctrl Pts',(-3.,59.993749998771,-5.19615242270663));
#8802=CARTESIAN_POINT('Ctrl Pts',(-6.,60.031249998771,-3.46410161513776));
#8803=CARTESIAN_POINT('Ctrl Pts',(-6.,60.068749998771,-7.34788079488412E-16));
#8804=CARTESIAN_POINT('Ctrl Pts',(-6.,60.106249998771,3.46410161513775));
#8805=CARTESIAN_POINT('Ctrl Pts',(-3.,60.143749998771,5.19615242270663));
#8806=CARTESIAN_POINT('Ctrl Pts',(-1.27269028646989E-15,60.181249998771,
6.92820323027551));
#8807=CARTESIAN_POINT('Ctrl Pts',(3.,60.218749998771,5.19615242270663));
#8808=CARTESIAN_POINT('Ctrl Pts',(6.,60.256249998771,3.46410161513776));
#8809=CARTESIAN_POINT('Ctrl Pts',(6.,60.293749998771,0.));
#8810=CARTESIAN_POINT('Ctrl Pts',(6.,60.331249998771,-3.46410161513775));
#8811=CARTESIAN_POINT('Ctrl Pts',(3.,60.368749998771,-5.19615242270663));
#8812=CARTESIAN_POINT('Ctrl Pts',(4.24230095489963E-16,60.406249998771,
-6.92820323027551));
#8813=CARTESIAN_POINT('Ctrl Pts',(-3.,60.443749998771,-5.19615242270663));
#8814=CARTESIAN_POINT('Ctrl Pts',(-6.,60.481249998771,-3.46410161513776));
#8815=CARTESIAN_POINT('Ctrl Pts',(-6.,60.518749998771,-7.34788079488412E-16));
#8816=CARTESIAN_POINT('Ctrl Pts',(-6.,60.556249998771,3.46410161513775));
#8817=CARTESIAN_POINT('Ctrl Pts',(-3.,60.593749998771,5.19615242270663));
#8818=CARTESIAN_POINT('Ctrl Pts',(-1.27269028646989E-15,60.631249998771,
6.92820323027551));
#8819=CARTESIAN_POINT('Ctrl Pts',(3.,60.668749998771,5.19615242270663));
#8820=CARTESIAN_POINT('Ctrl Pts',(6.,60.706249998771,3.46410161513776));
#8821=CARTESIAN_POINT('Ctrl Pts',(6.,60.743749998771,0.));
#8822=CARTESIAN_POINT('Ctrl Pts',(6.,60.781249998771,-3.46410161513775));
#8823=CARTESIAN_POINT('Ctrl Pts',(3.,60.818749998771,-5.19615242270663));
#8824=CARTESIAN_POINT('Ctrl Pts',(4.24230095489963E-16,60.856249998771,
-6.92820323027551));
#8825=CARTESIAN_POINT('Ctrl Pts',(-3.,60.893749998771,-5.19615242270663));
#8826=CARTESIAN_POINT('Ctrl Pts',(-6.,60.931249998771,-3.46410161513776));
#8827=CARTESIAN_POINT('Ctrl Pts',(-6.,60.968749998771,-7.34788079488412E-16));
#8828=CARTESIAN_POINT('Ctrl Pts',(-6.,61.0062499987709,3.46410161513775));
#8829=CARTESIAN_POINT('Ctrl Pts',(-3.,61.043749998771,5.19615242270663));
#8830=CARTESIAN_POINT('Ctrl Pts',(-1.27269028646989E-15,61.081249998771,
6.92820323027551));
#8831=CARTESIAN_POINT('Ctrl Pts',(3.,61.118749998771,5.19615242270663));
#8832=CARTESIAN_POINT('Ctrl Pts',(6.,61.156249998771,3.46410161513776));
#8833=CARTESIAN_POINT('Ctrl Pts',(6.,61.193749998771,0.));
#8834=CARTESIAN_POINT('Ctrl Pts',(6.,61.231249998771,-3.46410161513775));
#8835=CARTESIAN_POINT('Ctrl Pts',(3.,61.268749998771,-5.19615242270663));
#8836=CARTESIAN_POINT('Ctrl Pts',(4.24230095489963E-16,61.306249998771,
-6.92820323027551));
#8837=CARTESIAN_POINT('Ctrl Pts',(-3.,61.343749998771,-5.19615242270663));
#8838=CARTESIAN_POINT('Ctrl Pts',(-6.,61.381249998771,-3.46410161513776));
#8839=CARTESIAN_POINT('Ctrl Pts',(-6.,61.418749998771,-7.34788079488412E-16));
#8840=CARTESIAN_POINT('Ctrl Pts',(-6.,61.456249998771,3.46410161513775));
#8841=CARTESIAN_POINT('Ctrl Pts',(-3.,61.493749998771,5.19615242270663));
#8842=CARTESIAN_POINT('Ctrl Pts',(-1.27269028646989E-15,61.531249998771,
6.92820323027551));
#8843=CARTESIAN_POINT('Ctrl Pts',(3.,61.568749998771,5.19615242270663));
#8844=CARTESIAN_POINT('Ctrl Pts',(6.,61.606249998771,3.46410161513776));
#8845=CARTESIAN_POINT('Ctrl Pts',(6.,61.643749998771,0.));
#8846=CARTESIAN_POINT('Ctrl Pts',(6.,61.681249998771,-3.46410161513775));
#8847=CARTESIAN_POINT('Ctrl Pts',(3.,61.718749998771,-5.19615242270663));
#8848=CARTESIAN_POINT('Ctrl Pts',(4.24230095489963E-16,61.756249998771,
-6.92820323027551));
#8849=CARTESIAN_POINT('Ctrl Pts',(-3.,61.793749998771,-5.19615242270663));
#8850=CARTESIAN_POINT('Ctrl Pts',(-6.,61.831249998771,-3.46410161513776));
#8851=CARTESIAN_POINT('Ctrl Pts',(-6.,61.868749998771,-7.34788079488412E-16));
#8852=CARTESIAN_POINT('Ctrl Pts',(-6.,61.906249998771,3.46410161513775));
#8853=CARTESIAN_POINT('Ctrl Pts',(-3.,61.943749998771,5.19615242270663));
#8854=CARTESIAN_POINT('Ctrl Pts',(-1.27269028646989E-15,61.981249998771,
6.92820323027551));
#8855=CARTESIAN_POINT('Ctrl Pts',(3.,62.018749998771,5.19615242270663));
#8856=CARTESIAN_POINT('Ctrl Pts',(6.,62.056249998771,3.46410161513776));
#8857=CARTESIAN_POINT('Ctrl Pts',(6.,62.093749998771,0.));
#8858=CARTESIAN_POINT('Ctrl Pts',(6.,62.131249998771,-3.46410161513775));
#8859=CARTESIAN_POINT('Ctrl Pts',(3.,62.168749998771,-5.19615242270663));
#8860=CARTESIAN_POINT('Ctrl Pts',(4.24230095489963E-16,62.206249998771,
-6.92820323027551));
#8861=CARTESIAN_POINT('Ctrl Pts',(-3.,62.243749998771,-5.19615242270663));
#8862=CARTESIAN_POINT('Ctrl Pts',(-6.,62.281249998771,-3.46410161513776));
#8863=CARTESIAN_POINT('Ctrl Pts',(-6.,62.318749998771,-7.34788079488412E-16));
#8864=CARTESIAN_POINT('Ctrl Pts',(-6.,62.356249998771,3.46410161513775));
#8865=CARTESIAN_POINT('Ctrl Pts',(-3.,62.393749998771,5.19615242270663));
#8866=CARTESIAN_POINT('Ctrl Pts',(5.75643035625,50.2531249993855,0.));
#8867=CARTESIAN_POINT('Ctrl Pts',(5.75643035625,50.2906249993855,-3.32347661575227));
#8868=CARTESIAN_POINT('Ctrl Pts',(2.878215178125,50.3281249993855,-4.9852149236284));
#8869=CARTESIAN_POINT('Ctrl Pts',(4.0700849995221E-16,50.3656249993855,
-6.64695323150454));
#8870=CARTESIAN_POINT('Ctrl Pts',(-2.878215178125,50.4031249993855,-4.9852149236284));
#8871=CARTESIAN_POINT('Ctrl Pts',(-5.75643035625,50.4406249993855,-3.32347661575227));
#8872=CARTESIAN_POINT('Ctrl Pts',(-5.75643035625,50.4781249993855,-7.04959401029622E-16));
#8873=CARTESIAN_POINT('Ctrl Pts',(-5.75643035625,50.5156249993855,3.32347661575227));
#8874=CARTESIAN_POINT('Ctrl Pts',(-2.878215178125,50.5531249993855,4.9852149236284));
#8875=CARTESIAN_POINT('Ctrl Pts',(-1.22102549985663E-15,50.5906249993855,
6.64695323150454));
#8876=CARTESIAN_POINT('Ctrl Pts',(2.878215178125,50.6281249993855,4.98521492362841));
#8877=CARTESIAN_POINT('Ctrl Pts',(5.75643035625,50.6656249993855,3.32347661575227));
#8878=CARTESIAN_POINT('Ctrl Pts',(5.75643035625,50.7031249993855,0.));
#8879=CARTESIAN_POINT('Ctrl Pts',(5.75643035625,50.7406249993855,-3.32347661575227));
#8880=CARTESIAN_POINT('Ctrl Pts',(2.878215178125,50.7781249993855,-4.9852149236284));
#8881=CARTESIAN_POINT('Ctrl Pts',(4.0700849995221E-16,50.8156249993855,
-6.64695323150454));
#8882=CARTESIAN_POINT('Ctrl Pts',(-2.878215178125,50.8531249993855,-4.9852149236284));
#8883=CARTESIAN_POINT('Ctrl Pts',(-5.75643035625,50.8906249993855,-3.32347661575227));
#8884=CARTESIAN_POINT('Ctrl Pts',(-5.75643035625,50.9281249993855,-7.04959401029622E-16));
#8885=CARTESIAN_POINT('Ctrl Pts',(-5.75643035625,50.9656249993855,3.32347661575227));
#8886=CARTESIAN_POINT('Ctrl Pts',(-2.878215178125,51.0031249993855,4.9852149236284));
#8887=CARTESIAN_POINT('Ctrl Pts',(-1.22102549985663E-15,51.0406249993855,
6.64695323150454));
#8888=CARTESIAN_POINT('Ctrl Pts',(2.878215178125,51.0781249993855,4.98521492362841));
#8889=CARTESIAN_POINT('Ctrl Pts',(5.75643035625,51.1156249993855,3.32347661575227));
#8890=CARTESIAN_POINT('Ctrl Pts',(5.75643035625,51.1531249993855,0.));
#8891=CARTESIAN_POINT('Ctrl Pts',(5.75643035625,51.1906249993855,-3.32347661575227));
#8892=CARTESIAN_POINT('Ctrl Pts',(2.878215178125,51.2281249993855,-4.9852149236284));
#8893=CARTESIAN_POINT('Ctrl Pts',(4.0700849995221E-16,51.2656249993855,
-6.64695323150454));
#8894=CARTESIAN_POINT('Ctrl Pts',(-2.878215178125,51.3031249993855,-4.9852149236284));
#8895=CARTESIAN_POINT('Ctrl Pts',(-5.75643035625,51.3406249993855,-3.32347661575227));
#8896=CARTESIAN_POINT('Ctrl Pts',(-5.75643035625,51.3781249993855,-7.04959401029622E-16));
#8897=CARTESIAN_POINT('Ctrl Pts',(-5.75643035625,51.4156249993855,3.32347661575227));
#8898=CARTESIAN_POINT('Ctrl Pts',(-2.878215178125,51.4531249993855,4.9852149236284));
#8899=CARTESIAN_POINT('Ctrl Pts',(-1.22102549985663E-15,51.4906249993855,
6.64695323150454));
#8900=CARTESIAN_POINT('Ctrl Pts',(2.878215178125,51.5281249993855,4.98521492362841));
#8901=CARTESIAN_POINT('Ctrl Pts',(5.75643035625,51.5656249993855,3.32347661575227));
#8902=CARTESIAN_POINT('Ctrl Pts',(5.75643035625,51.6031249993855,0.));
#8903=CARTESIAN_POINT('Ctrl Pts',(5.75643035625,51.6406249993855,-3.32347661575227));
#8904=CARTESIAN_POINT('Ctrl Pts',(2.878215178125,51.6781249993855,-4.9852149236284));
#8905=CARTESIAN_POINT('Ctrl Pts',(4.0700849995221E-16,51.7156249993855,
-6.64695323150454));
#8906=CARTESIAN_POINT('Ctrl Pts',(-2.878215178125,51.7531249993855,-4.9852149236284));
#8907=CARTESIAN_POINT('Ctrl Pts',(-5.75643035625,51.7906249993855,-3.32347661575227));
#8908=CARTESIAN_POINT('Ctrl Pts',(-5.75643035625,51.8281249993855,-7.04959401029622E-16));
#8909=CARTESIAN_POINT('Ctrl Pts',(-5.75643035625,51.8656249993855,3.32347661575227));
#8910=CARTESIAN_POINT('Ctrl Pts',(-2.878215178125,51.9031249993855,4.9852149236284));
#8911=CARTESIAN_POINT('Ctrl Pts',(-1.22102549985663E-15,51.9406249993855,
6.64695323150454));
#8912=CARTESIAN_POINT('Ctrl Pts',(2.878215178125,51.9781249993855,4.98521492362841));
#8913=CARTESIAN_POINT('Ctrl Pts',(5.75643035625,52.0156249993855,3.32347661575227));
#8914=CARTESIAN_POINT('Ctrl Pts',(5.75643035625,52.0531249993855,0.));
#8915=CARTESIAN_POINT('Ctrl Pts',(5.75643035625,52.0906249993855,-3.32347661575227));
#8916=CARTESIAN_POINT('Ctrl Pts',(2.878215178125,52.1281249993855,-4.9852149236284));
#8917=CARTESIAN_POINT('Ctrl Pts',(4.0700849995221E-16,52.1656249993855,
-6.64695323150454));
#8918=CARTESIAN_POINT('Ctrl Pts',(-2.878215178125,52.2031249993855,-4.9852149236284));
#8919=CARTESIAN_POINT('Ctrl Pts',(-5.75643035625,52.2406249993855,-3.32347661575227));
#8920=CARTESIAN_POINT('Ctrl Pts',(-5.75643035625,52.2781249993855,-7.04959401029622E-16));
#8921=CARTESIAN_POINT('Ctrl Pts',(-5.75643035625,52.3156249993855,3.32347661575227));
#8922=CARTESIAN_POINT('Ctrl Pts',(-2.878215178125,52.3531249993855,4.9852149236284));
#8923=CARTESIAN_POINT('Ctrl Pts',(-1.22102549985663E-15,52.3906249993855,
6.64695323150454));
#8924=CARTESIAN_POINT('Ctrl Pts',(2.878215178125,52.4281249993855,4.98521492362841));
#8925=CARTESIAN_POINT('Ctrl Pts',(5.75643035625,52.4656249993855,3.32347661575227));
#8926=CARTESIAN_POINT('Ctrl Pts',(5.75643035625,52.5031249993855,0.));
#8927=CARTESIAN_POINT('Ctrl Pts',(5.75643035625,52.5406249993855,-3.32347661575227));
#8928=CARTESIAN_POINT('Ctrl Pts',(2.878215178125,52.5781249993855,-4.9852149236284));
#8929=CARTESIAN_POINT('Ctrl Pts',(4.0700849995221E-16,52.6156249993855,
-6.64695323150454));
#8930=CARTESIAN_POINT('Ctrl Pts',(-2.878215178125,52.6531249993855,-4.9852149236284));
#8931=CARTESIAN_POINT('Ctrl Pts',(-5.75643035625,52.6906249993855,-3.32347661575227));
#8932=CARTESIAN_POINT('Ctrl Pts',(-5.75643035625,52.7281249993855,-7.04959401029622E-16));
#8933=CARTESIAN_POINT('Ctrl Pts',(-5.75643035625,52.7656249993855,3.32347661575227));
#8934=CARTESIAN_POINT('Ctrl Pts',(-2.878215178125,52.8031249993855,4.9852149236284));
#8935=CARTESIAN_POINT('Ctrl Pts',(-1.22102549985663E-15,52.8406249993855,
6.64695323150454));
#8936=CARTESIAN_POINT('Ctrl Pts',(2.878215178125,52.8781249993855,4.98521492362841));
#8937=CARTESIAN_POINT('Ctrl Pts',(5.75643035625,52.9156249993855,3.32347661575227));
#8938=CARTESIAN_POINT('Ctrl Pts',(5.75643035625,52.9531249993855,0.));
#8939=CARTESIAN_POINT('Ctrl Pts',(5.75643035625,52.9906249993855,-3.32347661575227));
#8940=CARTESIAN_POINT('Ctrl Pts',(2.878215178125,53.0281249993855,-4.9852149236284));
#8941=CARTESIAN_POINT('Ctrl Pts',(4.0700849995221E-16,53.0656249993855,
-6.64695323150454));
#8942=CARTESIAN_POINT('Ctrl Pts',(-2.878215178125,53.1031249993855,-4.9852149236284));
#8943=CARTESIAN_POINT('Ctrl Pts',(-5.75643035625,53.1406249993855,-3.32347661575227));
#8944=CARTESIAN_POINT('Ctrl Pts',(-5.75643035625,53.1781249993855,-7.04959401029622E-16));
#8945=CARTESIAN_POINT('Ctrl Pts',(-5.75643035625,53.2156249993855,3.32347661575227));
#8946=CARTESIAN_POINT('Ctrl Pts',(-2.878215178125,53.2531249993855,4.9852149236284));
#8947=CARTESIAN_POINT('Ctrl Pts',(-1.22102549985663E-15,53.2906249993855,
6.64695323150454));
#8948=CARTESIAN_POINT('Ctrl Pts',(2.878215178125,53.3281249993855,4.98521492362841));
#8949=CARTESIAN_POINT('Ctrl Pts',(5.75643035625,53.3656249993855,3.32347661575227));
#8950=CARTESIAN_POINT('Ctrl Pts',(5.75643035625,53.4031249993855,0.));
#8951=CARTESIAN_POINT('Ctrl Pts',(5.75643035625,53.4406249993855,-3.32347661575227));
#8952=CARTESIAN_POINT('Ctrl Pts',(2.878215178125,53.4781249993855,-4.9852149236284));
#8953=CARTESIAN_POINT('Ctrl Pts',(4.0700849995221E-16,53.5156249993855,
-6.64695323150454));
#8954=CARTESIAN_POINT('Ctrl Pts',(-2.878215178125,53.5531249993855,-4.9852149236284));
#8955=CARTESIAN_POINT('Ctrl Pts',(-5.75643035625,53.5906249993855,-3.32347661575227));
#8956=CARTESIAN_POINT('Ctrl Pts',(-5.75643035625,53.6281249993855,-7.04959401029622E-16));
#8957=CARTESIAN_POINT('Ctrl Pts',(-5.75643035625,53.6656249993855,3.32347661575227));
#8958=CARTESIAN_POINT('Ctrl Pts',(-2.878215178125,53.7031249993855,4.9852149236284));
#8959=CARTESIAN_POINT('Ctrl Pts',(-1.22102549985663E-15,53.7406249993855,
6.64695323150454));
#8960=CARTESIAN_POINT('Ctrl Pts',(2.878215178125,53.7781249993855,4.98521492362841));
#8961=CARTESIAN_POINT('Ctrl Pts',(5.75643035625,53.8156249993855,3.32347661575227));
#8962=CARTESIAN_POINT('Ctrl Pts',(5.75643035625,53.8531249993855,0.));
#8963=CARTESIAN_POINT('Ctrl Pts',(5.75643035625,53.8906249993855,-3.32347661575227));
#8964=CARTESIAN_POINT('Ctrl Pts',(2.878215178125,53.9281249993855,-4.9852149236284));
#8965=CARTESIAN_POINT('Ctrl Pts',(4.0700849995221E-16,53.9656249993855,
-6.64695323150454));
#8966=CARTESIAN_POINT('Ctrl Pts',(-2.878215178125,54.0031249993855,-4.9852149236284));
#8967=CARTESIAN_POINT('Ctrl Pts',(-5.75643035625,54.0406249993855,-3.32347661575227));
#8968=CARTESIAN_POINT('Ctrl Pts',(-5.75643035625,54.0781249993855,-7.04959401029622E-16));
#8969=CARTESIAN_POINT('Ctrl Pts',(-5.75643035625,54.1156249993855,3.32347661575227));
#8970=CARTESIAN_POINT('Ctrl Pts',(-2.878215178125,54.1531249993855,4.9852149236284));
#8971=CARTESIAN_POINT('Ctrl Pts',(-1.22102549985663E-15,54.1906249993855,
6.64695323150454));
#8972=CARTESIAN_POINT('Ctrl Pts',(2.878215178125,54.2281249993855,4.98521492362841));
#8973=CARTESIAN_POINT('Ctrl Pts',(5.75643035625,54.2656249993855,3.32347661575227));
#8974=CARTESIAN_POINT('Ctrl Pts',(5.75643035625,54.3031249993855,0.));
#8975=CARTESIAN_POINT('Ctrl Pts',(5.75643035625,54.3406249993855,-3.32347661575227));
#8976=CARTESIAN_POINT('Ctrl Pts',(2.878215178125,54.3781249993855,-4.9852149236284));
#8977=CARTESIAN_POINT('Ctrl Pts',(4.0700849995221E-16,54.4156249993855,
-6.64695323150454));
#8978=CARTESIAN_POINT('Ctrl Pts',(-2.878215178125,54.4531249993855,-4.9852149236284));
#8979=CARTESIAN_POINT('Ctrl Pts',(-5.75643035625,54.4906249993855,-3.32347661575227));
#8980=CARTESIAN_POINT('Ctrl Pts',(-5.75643035625,54.5281249993855,-7.04959401029622E-16));
#8981=CARTESIAN_POINT('Ctrl Pts',(-5.75643035625,54.5656249993855,3.32347661575227));
#8982=CARTESIAN_POINT('Ctrl Pts',(-2.878215178125,54.6031249993855,4.9852149236284));
#8983=CARTESIAN_POINT('Ctrl Pts',(-1.22102549985663E-15,54.6406249993855,
6.64695323150454));
#8984=CARTESIAN_POINT('Ctrl Pts',(2.878215178125,54.6781249993855,4.98521492362841));
#8985=CARTESIAN_POINT('Ctrl Pts',(5.75643035625,54.7156249993855,3.32347661575227));
#8986=CARTESIAN_POINT('Ctrl Pts',(5.75643035625,54.7531249993855,0.));
#8987=CARTESIAN_POINT('Ctrl Pts',(5.75643035625,54.7906249993855,-3.32347661575227));
#8988=CARTESIAN_POINT('Ctrl Pts',(2.878215178125,54.8281249993855,-4.9852149236284));
#8989=CARTESIAN_POINT('Ctrl Pts',(4.0700849995221E-16,54.8656249993855,
-6.64695323150454));
#8990=CARTESIAN_POINT('Ctrl Pts',(-2.878215178125,54.9031249993855,-4.9852149236284));
#8991=CARTESIAN_POINT('Ctrl Pts',(-5.75643035625,54.9406249993855,-3.32347661575227));
#8992=CARTESIAN_POINT('Ctrl Pts',(-5.75643035625,54.9781249993855,-7.04959401029622E-16));
#8993=CARTESIAN_POINT('Ctrl Pts',(-5.75643035625,55.0156249993855,3.32347661575227));
#8994=CARTESIAN_POINT('Ctrl Pts',(-2.878215178125,55.0531249993855,4.9852149236284));
#8995=CARTESIAN_POINT('Ctrl Pts',(-1.22102549985663E-15,55.0906249993855,
6.64695323150454));
#8996=CARTESIAN_POINT('Ctrl Pts',(2.878215178125,55.1281249993855,4.98521492362841));
#8997=CARTESIAN_POINT('Ctrl Pts',(5.75643035625,55.1656249993855,3.32347661575227));
#8998=CARTESIAN_POINT('Ctrl Pts',(5.75643035625,55.2031249993855,0.));
#8999=CARTESIAN_POINT('Ctrl Pts',(5.75643035625,55.2406249993855,-3.32347661575227));
#9000=CARTESIAN_POINT('Ctrl Pts',(2.878215178125,55.2781249993855,-4.9852149236284));
#9001=CARTESIAN_POINT('Ctrl Pts',(4.0700849995221E-16,55.3156249993855,
-6.64695323150454));
#9002=CARTESIAN_POINT('Ctrl Pts',(-2.878215178125,55.3531249993855,-4.9852149236284));
#9003=CARTESIAN_POINT('Ctrl Pts',(-5.75643035625,55.3906249993855,-3.32347661575227));
#9004=CARTESIAN_POINT('Ctrl Pts',(-5.75643035625,55.4281249993855,-7.04959401029622E-16));
#9005=CARTESIAN_POINT('Ctrl Pts',(-5.75643035625,55.4656249993855,3.32347661575227));
#9006=CARTESIAN_POINT('Ctrl Pts',(-2.878215178125,55.5031249993855,4.9852149236284));
#9007=CARTESIAN_POINT('Ctrl Pts',(-1.22102549985663E-15,55.5406249993855,
6.64695323150454));
#9008=CARTESIAN_POINT('Ctrl Pts',(2.878215178125,55.5781249993855,4.98521492362841));
#9009=CARTESIAN_POINT('Ctrl Pts',(5.75643035625,55.6156249993855,3.32347661575227));
#9010=CARTESIAN_POINT('Ctrl Pts',(5.75643035625,55.6531249993855,0.));
#9011=CARTESIAN_POINT('Ctrl Pts',(5.75643035625,55.6906249993855,-3.32347661575227));
#9012=CARTESIAN_POINT('Ctrl Pts',(2.878215178125,55.7281249993855,-4.9852149236284));
#9013=CARTESIAN_POINT('Ctrl Pts',(4.0700849995221E-16,55.7656249993855,
-6.64695323150454));
#9014=CARTESIAN_POINT('Ctrl Pts',(-2.878215178125,55.8031249993855,-4.9852149236284));
#9015=CARTESIAN_POINT('Ctrl Pts',(-5.75643035625,55.8406249993855,-3.32347661575227));
#9016=CARTESIAN_POINT('Ctrl Pts',(-5.75643035625,55.8781249993855,-7.04959401029622E-16));
#9017=CARTESIAN_POINT('Ctrl Pts',(-5.75643035625,55.9156249993855,3.32347661575227));
#9018=CARTESIAN_POINT('Ctrl Pts',(-2.878215178125,55.9531249993855,4.9852149236284));
#9019=CARTESIAN_POINT('Ctrl Pts',(-1.22102549985663E-15,55.9906249993855,
6.64695323150454));
#9020=CARTESIAN_POINT('Ctrl Pts',(2.878215178125,56.0281249993855,4.98521492362841));
#9021=CARTESIAN_POINT('Ctrl Pts',(5.75643035625,56.0656249993855,3.32347661575227));
#9022=CARTESIAN_POINT('Ctrl Pts',(5.75643035625,56.1031249993855,0.));
#9023=CARTESIAN_POINT('Ctrl Pts',(5.75643035625,56.1406249993855,-3.32347661575227));
#9024=CARTESIAN_POINT('Ctrl Pts',(2.878215178125,56.1781249993855,-4.9852149236284));
#9025=CARTESIAN_POINT('Ctrl Pts',(4.0700849995221E-16,56.2156249993855,
-6.64695323150454));
#9026=CARTESIAN_POINT('Ctrl Pts',(-2.878215178125,56.2531249993855,-4.9852149236284));
#9027=CARTESIAN_POINT('Ctrl Pts',(-5.75643035625,56.2906249993855,-3.32347661575227));
#9028=CARTESIAN_POINT('Ctrl Pts',(-5.75643035625,56.3281249993855,-7.04959401029622E-16));
#9029=CARTESIAN_POINT('Ctrl Pts',(-5.75643035625,56.3656249993855,3.32347661575227));
#9030=CARTESIAN_POINT('Ctrl Pts',(-2.878215178125,56.4031249993855,4.9852149236284));
#9031=CARTESIAN_POINT('Ctrl Pts',(-1.22102549985663E-15,56.4406249993855,
6.64695323150454));
#9032=CARTESIAN_POINT('Ctrl Pts',(2.878215178125,56.4781249993855,4.98521492362841));
#9033=CARTESIAN_POINT('Ctrl Pts',(5.75643035625,56.5156249993855,3.32347661575227));
#9034=CARTESIAN_POINT('Ctrl Pts',(5.75643035625,56.5531249993855,0.));
#9035=CARTESIAN_POINT('Ctrl Pts',(5.75643035625,56.5906249993855,-3.32347661575227));
#9036=CARTESIAN_POINT('Ctrl Pts',(2.878215178125,56.6281249993855,-4.9852149236284));
#9037=CARTESIAN_POINT('Ctrl Pts',(4.0700849995221E-16,56.6656249993855,
-6.64695323150454));
#9038=CARTESIAN_POINT('Ctrl Pts',(-2.878215178125,56.7031249993855,-4.9852149236284));
#9039=CARTESIAN_POINT('Ctrl Pts',(-5.75643035625,56.7406249993855,-3.32347661575227));
#9040=CARTESIAN_POINT('Ctrl Pts',(-5.75643035625,56.7781249993855,-7.04959401029622E-16));
#9041=CARTESIAN_POINT('Ctrl Pts',(-5.75643035625,56.8156249993855,3.32347661575227));
#9042=CARTESIAN_POINT('Ctrl Pts',(-2.878215178125,56.8531249993855,4.9852149236284));
#9043=CARTESIAN_POINT('Ctrl Pts',(-1.22102549985663E-15,56.8906249993855,
6.64695323150454));
#9044=CARTESIAN_POINT('Ctrl Pts',(2.878215178125,56.9281249993855,4.98521492362841));
#9045=CARTESIAN_POINT('Ctrl Pts',(5.75643035625,56.9656249993855,3.32347661575227));
#9046=CARTESIAN_POINT('Ctrl Pts',(5.75643035625,57.0031249993855,0.));
#9047=CARTESIAN_POINT('Ctrl Pts',(5.75643035625,57.0406249993855,-3.32347661575227));
#9048=CARTESIAN_POINT('Ctrl Pts',(2.878215178125,57.0781249993855,-4.9852149236284));
#9049=CARTESIAN_POINT('Ctrl Pts',(4.0700849995221E-16,57.1156249993855,
-6.64695323150454));
#9050=CARTESIAN_POINT('Ctrl Pts',(-2.878215178125,57.1531249993855,-4.9852149236284));
#9051=CARTESIAN_POINT('Ctrl Pts',(-5.75643035625,57.1906249993855,-3.32347661575227));
#9052=CARTESIAN_POINT('Ctrl Pts',(-5.75643035625,57.2281249993855,-7.04959401029622E-16));
#9053=CARTESIAN_POINT('Ctrl Pts',(-5.75643035625,57.2656249993855,3.32347661575227));
#9054=CARTESIAN_POINT('Ctrl Pts',(-2.878215178125,57.3031249993855,4.9852149236284));
#9055=CARTESIAN_POINT('Ctrl Pts',(-1.22102549985663E-15,57.3406249993855,
6.64695323150454));
#9056=CARTESIAN_POINT('Ctrl Pts',(2.878215178125,57.3781249993855,4.98521492362841));
#9057=CARTESIAN_POINT('Ctrl Pts',(5.75643035625,57.4156249993855,3.32347661575227));
#9058=CARTESIAN_POINT('Ctrl Pts',(5.75643035625,57.4531249993855,0.));
#9059=CARTESIAN_POINT('Ctrl Pts',(5.75643035625,57.4906249993855,-3.32347661575227));
#9060=CARTESIAN_POINT('Ctrl Pts',(2.878215178125,57.5281249993855,-4.9852149236284));
#9061=CARTESIAN_POINT('Ctrl Pts',(4.0700849995221E-16,57.5656249993855,
-6.64695323150454));
#9062=CARTESIAN_POINT('Ctrl Pts',(-2.878215178125,57.6031249993855,-4.9852149236284));
#9063=CARTESIAN_POINT('Ctrl Pts',(-5.75643035625,57.6406249993855,-3.32347661575227));
#9064=CARTESIAN_POINT('Ctrl Pts',(-5.75643035625,57.6781249993855,-7.04959401029622E-16));
#9065=CARTESIAN_POINT('Ctrl Pts',(-5.75643035625,57.7156249993855,3.32347661575227));
#9066=CARTESIAN_POINT('Ctrl Pts',(-2.878215178125,57.7531249993855,4.9852149236284));
#9067=CARTESIAN_POINT('Ctrl Pts',(-1.22102549985663E-15,57.7906249993855,
6.64695323150454));
#9068=CARTESIAN_POINT('Ctrl Pts',(2.878215178125,57.8281249993855,4.98521492362841));
#9069=CARTESIAN_POINT('Ctrl Pts',(5.75643035625,57.8656249993855,3.32347661575227));
#9070=CARTESIAN_POINT('Ctrl Pts',(5.75643035625,57.9031249993855,0.));
#9071=CARTESIAN_POINT('Ctrl Pts',(5.75643035625,57.9406249993855,-3.32347661575227));
#9072=CARTESIAN_POINT('Ctrl Pts',(2.878215178125,57.9781249993855,-4.9852149236284));
#9073=CARTESIAN_POINT('Ctrl Pts',(4.0700849995221E-16,58.0156249993855,
-6.64695323150454));
#9074=CARTESIAN_POINT('Ctrl Pts',(-2.878215178125,58.0531249993855,-4.9852149236284));
#9075=CARTESIAN_POINT('Ctrl Pts',(-5.75643035625,58.0906249993855,-3.32347661575227));
#9076=CARTESIAN_POINT('Ctrl Pts',(-5.75643035625,58.1281249993855,-7.04959401029622E-16));
#9077=CARTESIAN_POINT('Ctrl Pts',(-5.75643035625,58.1656249993855,3.32347661575227));
#9078=CARTESIAN_POINT('Ctrl Pts',(-2.878215178125,58.2031249993855,4.9852149236284));
#9079=CARTESIAN_POINT('Ctrl Pts',(-1.22102549985663E-15,58.2406249993855,
6.64695323150454));
#9080=CARTESIAN_POINT('Ctrl Pts',(2.878215178125,58.2781249993855,4.98521492362841));
#9081=CARTESIAN_POINT('Ctrl Pts',(5.75643035625,58.3156249993855,3.32347661575227));
#9082=CARTESIAN_POINT('Ctrl Pts',(5.75643035625,58.3531249993855,0.));
#9083=CARTESIAN_POINT('Ctrl Pts',(5.75643035625,58.3906249993855,-3.32347661575227));
#9084=CARTESIAN_POINT('Ctrl Pts',(2.878215178125,58.4281249993855,-4.9852149236284));
#9085=CARTESIAN_POINT('Ctrl Pts',(4.0700849995221E-16,58.4656249993855,
-6.64695323150454));
#9086=CARTESIAN_POINT('Ctrl Pts',(-2.878215178125,58.5031249993855,-4.9852149236284));
#9087=CARTESIAN_POINT('Ctrl Pts',(-5.75643035625,58.5406249993855,-3.32347661575227));
#9088=CARTESIAN_POINT('Ctrl Pts',(-5.75643035625,58.5781249993855,-7.04959401029622E-16));
#9089=CARTESIAN_POINT('Ctrl Pts',(-5.75643035625,58.6156249993855,3.32347661575227));
#9090=CARTESIAN_POINT('Ctrl Pts',(-2.878215178125,58.6531249993855,4.9852149236284));
#9091=CARTESIAN_POINT('Ctrl Pts',(-1.22102549985663E-15,58.6906249993855,
6.64695323150454));
#9092=CARTESIAN_POINT('Ctrl Pts',(2.878215178125,58.7281249993855,4.98521492362841));
#9093=CARTESIAN_POINT('Ctrl Pts',(5.75643035625,58.7656249993855,3.32347661575227));
#9094=CARTESIAN_POINT('Ctrl Pts',(5.75643035625,58.8031249993855,0.));
#9095=CARTESIAN_POINT('Ctrl Pts',(5.75643035625,58.8406249993855,-3.32347661575227));
#9096=CARTESIAN_POINT('Ctrl Pts',(2.878215178125,58.8781249993855,-4.9852149236284));
#9097=CARTESIAN_POINT('Ctrl Pts',(4.0700849995221E-16,58.9156249993855,
-6.64695323150454));
#9098=CARTESIAN_POINT('Ctrl Pts',(-2.878215178125,58.9531249993855,-4.9852149236284));
#9099=CARTESIAN_POINT('Ctrl Pts',(-5.75643035625,58.9906249993855,-3.32347661575227));
#9100=CARTESIAN_POINT('Ctrl Pts',(-5.75643035625,59.0281249993855,-7.04959401029622E-16));
#9101=CARTESIAN_POINT('Ctrl Pts',(-5.75643035625,59.0656249993855,3.32347661575227));
#9102=CARTESIAN_POINT('Ctrl Pts',(-2.878215178125,59.1031249993855,4.9852149236284));
#9103=CARTESIAN_POINT('Ctrl Pts',(-1.22102549985663E-15,59.1406249993855,
6.64695323150454));
#9104=CARTESIAN_POINT('Ctrl Pts',(2.878215178125,59.1781249993855,4.98521492362841));
#9105=CARTESIAN_POINT('Ctrl Pts',(5.75643035625,59.2156249993855,3.32347661575227));
#9106=CARTESIAN_POINT('Ctrl Pts',(5.75643035625,59.2531249993855,0.));
#9107=CARTESIAN_POINT('Ctrl Pts',(5.75643035625,59.2906249993855,-3.32347661575227));
#9108=CARTESIAN_POINT('Ctrl Pts',(2.878215178125,59.3281249993855,-4.9852149236284));
#9109=CARTESIAN_POINT('Ctrl Pts',(4.0700849995221E-16,59.3656249993855,
-6.64695323150454));
#9110=CARTESIAN_POINT('Ctrl Pts',(-2.878215178125,59.4031249993855,-4.9852149236284));
#9111=CARTESIAN_POINT('Ctrl Pts',(-5.75643035625,59.4406249993855,-3.32347661575227));
#9112=CARTESIAN_POINT('Ctrl Pts',(-5.75643035625,59.4781249993855,-7.04959401029622E-16));
#9113=CARTESIAN_POINT('Ctrl Pts',(-5.75643035625,59.5156249993855,3.32347661575227));
#9114=CARTESIAN_POINT('Ctrl Pts',(-2.878215178125,59.5531249993855,4.9852149236284));
#9115=CARTESIAN_POINT('Ctrl Pts',(-1.22102549985663E-15,59.5906249993855,
6.64695323150454));
#9116=CARTESIAN_POINT('Ctrl Pts',(2.878215178125,59.6281249993855,4.98521492362841));
#9117=CARTESIAN_POINT('Ctrl Pts',(5.75643035625,59.6656249993855,3.32347661575227));
#9118=CARTESIAN_POINT('Ctrl Pts',(5.75643035625,59.7031249993855,0.));
#9119=CARTESIAN_POINT('Ctrl Pts',(5.75643035625,59.7406249993855,-3.32347661575227));
#9120=CARTESIAN_POINT('Ctrl Pts',(2.878215178125,59.7781249993855,-4.9852149236284));
#9121=CARTESIAN_POINT('Ctrl Pts',(4.0700849995221E-16,59.8156249993855,
-6.64695323150454));
#9122=CARTESIAN_POINT('Ctrl Pts',(-2.878215178125,59.8531249993855,-4.9852149236284));
#9123=CARTESIAN_POINT('Ctrl Pts',(-5.75643035625,59.8906249993855,-3.32347661575227));
#9124=CARTESIAN_POINT('Ctrl Pts',(-5.75643035625,59.9281249993855,-7.04959401029622E-16));
#9125=CARTESIAN_POINT('Ctrl Pts',(-5.75643035625,59.9656249993855,3.32347661575227));
#9126=CARTESIAN_POINT('Ctrl Pts',(-2.878215178125,60.0031249993855,4.9852149236284));
#9127=CARTESIAN_POINT('Ctrl Pts',(-1.22102549985663E-15,60.0406249993855,
6.64695323150454));
#9128=CARTESIAN_POINT('Ctrl Pts',(2.878215178125,60.0781249993855,4.98521492362841));
#9129=CARTESIAN_POINT('Ctrl Pts',(5.75643035625,60.1156249993855,3.32347661575227));
#9130=CARTESIAN_POINT('Ctrl Pts',(5.75643035625,60.1531249993855,0.));
#9131=CARTESIAN_POINT('Ctrl Pts',(5.75643035625,60.1906249993855,-3.32347661575227));
#9132=CARTESIAN_POINT('Ctrl Pts',(2.878215178125,60.2281249993855,-4.9852149236284));
#9133=CARTESIAN_POINT('Ctrl Pts',(4.0700849995221E-16,60.2656249993855,
-6.64695323150454));
#9134=CARTESIAN_POINT('Ctrl Pts',(-2.878215178125,60.3031249993855,-4.9852149236284));
#9135=CARTESIAN_POINT('Ctrl Pts',(-5.75643035625,60.3406249993855,-3.32347661575227));
#9136=CARTESIAN_POINT('Ctrl Pts',(-5.75643035625,60.3781249993855,-7.04959401029622E-16));
#9137=CARTESIAN_POINT('Ctrl Pts',(-5.75643035625,60.4156249993855,3.32347661575227));
#9138=CARTESIAN_POINT('Ctrl Pts',(-2.878215178125,60.4531249993855,4.9852149236284));
#9139=CARTESIAN_POINT('Ctrl Pts',(-1.22102549985663E-15,60.4906249993855,
6.64695323150454));
#9140=CARTESIAN_POINT('Ctrl Pts',(2.878215178125,60.5281249993855,4.98521492362841));
#9141=CARTESIAN_POINT('Ctrl Pts',(5.75643035625,60.5656249993855,3.32347661575227));
#9142=CARTESIAN_POINT('Ctrl Pts',(5.75643035625,60.6031249993855,0.));
#9143=CARTESIAN_POINT('Ctrl Pts',(5.75643035625,60.6406249993855,-3.32347661575227));
#9144=CARTESIAN_POINT('Ctrl Pts',(2.878215178125,60.6781249993855,-4.9852149236284));
#9145=CARTESIAN_POINT('Ctrl Pts',(4.0700849995221E-16,60.7156249993855,
-6.64695323150454));
#9146=CARTESIAN_POINT('Ctrl Pts',(-2.878215178125,60.7531249993855,-4.9852149236284));
#9147=CARTESIAN_POINT('Ctrl Pts',(-5.75643035625,60.7906249993855,-3.32347661575227));
#9148=CARTESIAN_POINT('Ctrl Pts',(-5.75643035625,60.8281249993855,-7.04959401029622E-16));
#9149=CARTESIAN_POINT('Ctrl Pts',(-5.75643035625,60.8656249993855,3.32347661575227));
#9150=CARTESIAN_POINT('Ctrl Pts',(-2.878215178125,60.9031249993855,4.9852149236284));
#9151=CARTESIAN_POINT('Ctrl Pts',(-1.22102549985663E-15,60.9406249993855,
6.64695323150454));
#9152=CARTESIAN_POINT('Ctrl Pts',(2.878215178125,60.9781249993855,4.98521492362841));
#9153=CARTESIAN_POINT('Ctrl Pts',(5.75643035625,61.0156249993855,3.32347661575227));
#9154=CARTESIAN_POINT('Ctrl Pts',(5.75643035625,61.0531249993855,0.));
#9155=CARTESIAN_POINT('Ctrl Pts',(5.75643035625,61.0906249993855,-3.32347661575227));
#9156=CARTESIAN_POINT('Ctrl Pts',(2.878215178125,61.1281249993855,-4.9852149236284));
#9157=CARTESIAN_POINT('Ctrl Pts',(4.0700849995221E-16,61.1656249993855,
-6.64695323150454));
#9158=CARTESIAN_POINT('Ctrl Pts',(-2.878215178125,61.2031249993855,-4.9852149236284));
#9159=CARTESIAN_POINT('Ctrl Pts',(-5.75643035625,61.2406249993855,-3.32347661575227));
#9160=CARTESIAN_POINT('Ctrl Pts',(-5.75643035625,61.2781249993855,-7.04959401029622E-16));
#9161=CARTESIAN_POINT('Ctrl Pts',(-5.75643035625,61.3156249993855,3.32347661575227));
#9162=CARTESIAN_POINT('Ctrl Pts',(-2.878215178125,61.3531249993855,4.9852149236284));
#9163=CARTESIAN_POINT('Ctrl Pts',(-1.22102549985663E-15,61.3906249993855,
6.64695323150454));
#9164=CARTESIAN_POINT('Ctrl Pts',(2.878215178125,61.4281249993855,4.98521492362841));
#9165=CARTESIAN_POINT('Ctrl Pts',(5.75643035625,61.4656249993855,3.32347661575227));
#9166=CARTESIAN_POINT('Ctrl Pts',(5.75643035625,61.5031249993855,0.));
#9167=CARTESIAN_POINT('Ctrl Pts',(5.75643035625,61.5406249993855,-3.32347661575227));
#9168=CARTESIAN_POINT('Ctrl Pts',(2.878215178125,61.5781249993855,-4.9852149236284));
#9169=CARTESIAN_POINT('Ctrl Pts',(4.0700849995221E-16,61.6156249993855,
-6.64695323150454));
#9170=CARTESIAN_POINT('Ctrl Pts',(-2.878215178125,61.6531249993855,-4.9852149236284));
#9171=CARTESIAN_POINT('Ctrl Pts',(-5.75643035625,61.6906249993855,-3.32347661575227));
#9172=CARTESIAN_POINT('Ctrl Pts',(-5.75643035625,61.7281249993855,-7.04959401029622E-16));
#9173=CARTESIAN_POINT('Ctrl Pts',(-5.75643035625,61.7656249993855,3.32347661575227));
#9174=CARTESIAN_POINT('Ctrl Pts',(-2.878215178125,61.8031249993855,4.9852149236284));
#9175=CARTESIAN_POINT('Ctrl Pts',(-1.22102549985663E-15,61.8406249993855,
6.64695323150454));
#9176=CARTESIAN_POINT('Ctrl Pts',(2.878215178125,61.8781249993855,4.98521492362841));
#9177=CARTESIAN_POINT('Ctrl Pts',(5.75643035625,61.9156249993855,3.32347661575227));
#9178=CARTESIAN_POINT('Ctrl Pts',(5.75643035625,61.9531249993855,0.));
#9179=CARTESIAN_POINT('Ctrl Pts',(5.75643035625,61.9906249993855,-3.32347661575227));
#9180=CARTESIAN_POINT('Ctrl Pts',(2.878215178125,62.0281249993855,-4.9852149236284));
#9181=CARTESIAN_POINT('Ctrl Pts',(4.0700849995221E-16,62.0656249993855,
-6.64695323150454));
#9182=CARTESIAN_POINT('Ctrl Pts',(-2.878215178125,62.1031249993855,-4.9852149236284));
#9183=CARTESIAN_POINT('Ctrl Pts',(-5.75643035625,62.1406249993855,-3.32347661575227));
#9184=CARTESIAN_POINT('Ctrl Pts',(-5.75643035625,62.1781249993855,-7.04959401029622E-16));
#9185=CARTESIAN_POINT('Ctrl Pts',(-5.75643035625,62.2156249993855,3.32347661575227));
#9186=CARTESIAN_POINT('Ctrl Pts',(-2.878215178125,62.2531249993855,4.9852149236284));
#14066=UNCERTAINTY_MEASURE_WITH_UNIT(LENGTH_MEASURE(0.01),#14085,
'DISTANCE_ACCURACY_VALUE',
'Maximum model space distance between geometric entities at asserted c
onnectivities');
#14073=UNCERTAINTY_MEASURE_WITH_UNIT(LENGTH_MEASURE(0.01),#14085,
'DISTANCE_ACCURACY_VALUE',
'Maximum model space distance between geometric entities at asserted c
onnectivities');
#14077=(
GEOMETRIC_REPRESENTATION_CONTEXT(3)
GLOBAL_UNCERTAINTY_ASSIGNED_CONTEXT((#14066))
GLOBAL_UNIT_ASSIGNED_CONTEXT((#14085,#14087,#14088))
REPRESENTATION_CONTEXT('','3D')
);
#14084=(
GEOMETRIC_REPRESENTATION_CONTEXT(3)
GLOBAL_UNCERTAINTY_ASSIGNED_CONTEXT((#14073))
GLOBAL_UNIT_ASSIGNED_CONTEXT((#14085,#14087,#14088))
REPRESENTATION_CONTEXT('','3D')
);
#14085=(
LENGTH_UNIT()
NAMED_UNIT(*)
SI_UNIT(.MILLI.,.METRE.)
);
#14087=(
NAMED_UNIT(*)
PLANE_ANGLE_UNIT()
SI_UNIT($,.RADIAN.)
);
#14088=(
NAMED_UNIT(*)
SI_UNIT($,.STERADIAN.)
SOLID_ANGLE_UNIT()
);
#14092=SHAPE_DEFINITION_REPRESENTATION(#14102,#14122);
#14102=PRODUCT_DEFINITION_SHAPE('',$,#14133);
#14122=SHAPE_REPRESENTATION('',(#3649),#14077);
#14129=PRODUCT_DEFINITION_CONTEXT('part definition',#14161,'design');
#14133=PRODUCT_DEFINITION('centre rod','centre rod',#14143,#14129);
#14143=PRODUCT_DEFINITION_FORMATION('',$,#14166);
#14161=APPLICATION_CONTEXT(
'Core Data for Automotive Mechanical Design Process');
#14162=PRODUCT_CONTEXT('part definition',#14161,'mechanical');
#14166=PRODUCT('centre rod','centre rod',$,(#14162));
#14176=PRESENTATION_STYLE_ASSIGNMENT((#14182));
#14182=SURFACE_STYLE_USAGE(.BOTH.,#14188);
#14188=SURFACE_SIDE_STYLE('',(#14194));
#14194=SURFACE_STYLE_FILL_AREA(#14200);
#14200=FILL_AREA_STYLE('Opaque(122,133,145)',(#14206));
#14206=FILL_AREA_STYLE_COLOUR('Opaque(122,133,145)',#14212);
#14212=COLOUR_RGB('Opaque(122,133,145)',0.47843137254902,0.52156862745098,
0.568627450980392);
ENDSEC;
END-ISO-10303-21;
